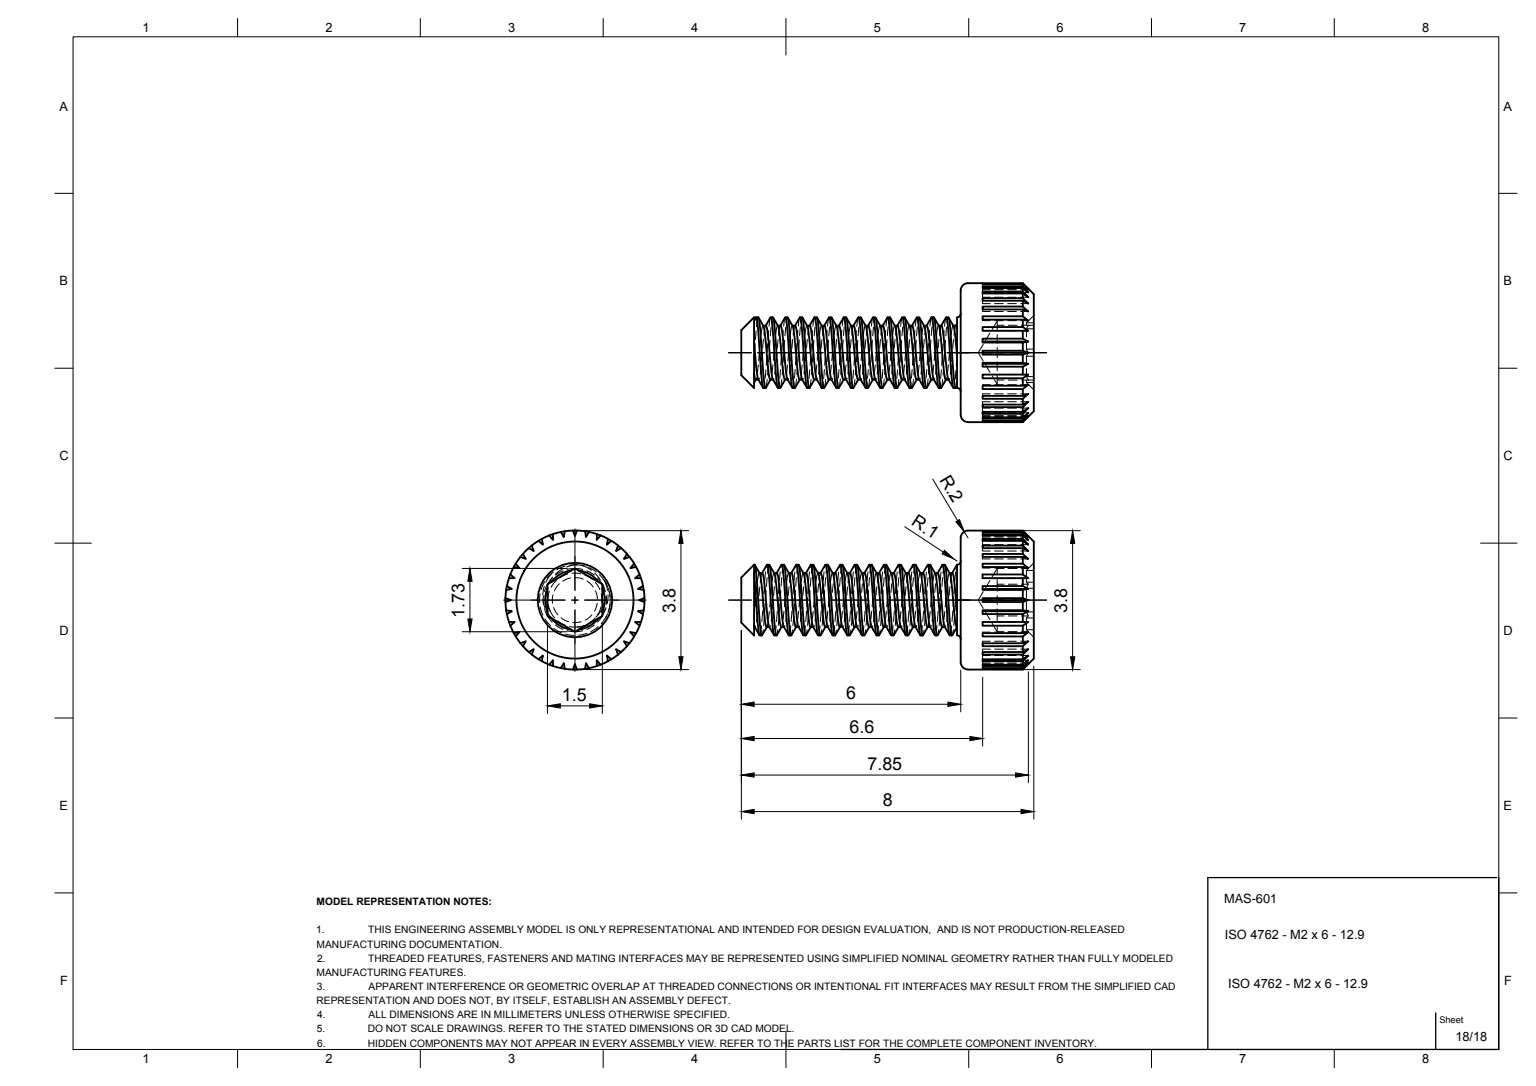
ISO-10303-21;
HEADER;
FILE_DESCRIPTION((''),'2;1');
FILE_NAME('ISO 4762 - M2 x 6 - 12.9.step','2026-10-06T07:37:42+05:00',(''),(''),'','','');
FILE_SCHEMA (('AUTOMOTIVE_DESIGN { 1 0 10303 214 3 1 1 }'));
ENDSEC;
DATA;
#10=MECHANICAL_DESIGN_GEOMETRIC_PRESENTATION_REPRESENTATION('',(#386),#18757);
#243=B_SPLINE_SURFACE_WITH_KNOTS('',3,3,((#16462,#16463,#16464,#16465,#16466,
#16467,#16468,#16469,#16470,#16471,#16472,#16473,#16474,#16475,#16476,#16477,
#16478,#16479,#16480,#16481,#16482,#16483,#16484,#16485,#16486,#16487,#16488,
#16489,#16490,#16491,#16492,#16493,#16494,#16495,#16496,#16497,#16498,#16499,
#16500,#16501,#16502,#16503,#16504,#16505,#16506,#16507,#16508,#16509,#16510,
#16511,#16512,#16513,#16514,#16515,#16516,#16517,#16518,#16519,#16520,#16521,
#16522,#16523,#16524,#16525,#16526,#16527,#16528,#16529,#16530,#16531,#16532,
#16533,#16534,#16535,#16536,#16537,#16538,#16539,#16540,#16541,#16542,#16543,
#16544,#16545,#16546,#16547,#16548,#16549,#16550,#16551,#16552,#16553,#16554),
(#16555,#16556,#16557,#16558,#16559,#16560,#16561,#16562,#16563,#16564,
#16565,#16566,#16567,#16568,#16569,#16570,#16571,#16572,#16573,#16574,#16575,
#16576,#16577,#16578,#16579,#16580,#16581,#16582,#16583,#16584,#16585,#16586,
#16587,#16588,#16589,#16590,#16591,#16592,#16593,#16594,#16595,#16596,#16597,
#16598,#16599,#16600,#16601,#16602,#16603,#16604,#16605,#16606,#16607,#16608,
#16609,#16610,#16611,#16612,#16613,#16614,#16615,#16616,#16617,#16618,#16619,
#16620,#16621,#16622,#16623,#16624,#16625,#16626,#16627,#16628,#16629,#16630,
#16631,#16632,#16633,#16634,#16635,#16636,#16637,#16638,#16639,#16640,#16641,
#16642,#16643,#16644,#16645,#16646,#16647),(#16648,#16649,#16650,#16651,
#16652,#16653,#16654,#16655,#16656,#16657,#16658,#16659,#16660,#16661,#16662,
#16663,#16664,#16665,#16666,#16667,#16668,#16669,#16670,#16671,#16672,#16673,
#16674,#16675,#16676,#16677,#16678,#16679,#16680,#16681,#16682,#16683,#16684,
#16685,#16686,#16687,#16688,#16689,#16690,#16691,#16692,#16693,#16694,#16695,
#16696,#16697,#16698,#16699,#16700,#16701,#16702,#16703,#16704,#16705,#16706,
#16707,#16708,#16709,#16710,#16711,#16712,#16713,#16714,#16715,#16716,#16717,
#16718,#16719,#16720,#16721,#16722,#16723,#16724,#16725,#16726,#16727,#16728,
#16729,#16730,#16731,#16732,#16733,#16734,#16735,#16736,#16737,#16738,#16739,
#16740),(#16741,#16742,#16743,#16744,#16745,#16746,#16747,#16748,#16749,
#16750,#16751,#16752,#16753,#16754,#16755,#16756,#16757,#16758,#16759,#16760,
#16761,#16762,#16763,#16764,#16765,#16766,#16767,#16768,#16769,#16770,#16771,
#16772,#16773,#16774,#16775,#16776,#16777,#16778,#16779,#16780,#16781,#16782,
#16783,#16784,#16785,#16786,#16787,#16788,#16789,#16790,#16791,#16792,#16793,
#16794,#16795,#16796,#16797,#16798,#16799,#16800,#16801,#16802,#16803,#16804,
#16805,#16806,#16807,#16808,#16809,#16810,#16811,#16812,#16813,#16814,#16815,
#16816,#16817,#16818,#16819,#16820,#16821,#16822,#16823,#16824,#16825,#16826,
#16827,#16828,#16829,#16830,#16831,#16832,#16833)),.UNSPECIFIED.,.F.,.F.,
 .F.,(4,4),(4,1,1,1,1,1,1,1,1,1,1,1,1,1,1,1,1,1,1,1,1,1,1,1,1,1,1,1,1,1,
1,1,1,1,1,1,1,1,1,1,1,1,1,1,1,1,1,1,1,1,1,1,1,1,1,1,1,1,1,1,1,1,1,1,1,1,
1,1,1,1,1,1,1,1,1,1,1,1,1,1,1,1,1,1,1,1,1,1,1,1,4),(0.,0.026298304761587),
(8.30929135176524,9.30089868691122,10.2925060220572,11.2841133572032,12.2757206923492,
13.2673280274952,14.2589353626411,15.2505426977871,16.2421500329331,17.2337573680791,
18.2253647032251,19.2169720383711,20.2085793735171,21.200186708663,22.191794043809,
23.183401378955,24.175008714101,25.166616049247,26.158223384393,27.149830719539,
28.1414380546849,29.1330453898309,30.1246527249769,31.1162600601229,32.1078673952689,
33.0994747304149,34.0910820655609,35.0826894007068,36.0742967358528,37.0659040709988,
38.0575114061448,39.0491187412908,40.0407260764368,41.0323334115828,42.0239407467287,
43.0155480818747,44.0071554170207,44.9987627521667,45.9903700873127,46.9819774224587,
47.9735847576047,48.9651920927506,49.9567994278966,50.9484067630426,51.9400140981886,
52.9316214333346,53.9232287684806,54.9148361036265,55.9064434387725,56.8980507739185,
57.8896581090645,58.8812654442105,59.8728727793565,60.8644801145025,61.8560874496484,
62.8476947847944,63.8393021199404,64.8309094550864,65.8225167902324,66.8141241253784,
67.8057314605244,68.7973387956703,69.7889461308163,70.7805534659623,71.7721608011083,
72.7637681362543,73.7553754714003,74.7469828065463,75.7385901416922,76.7301974768382,
77.7218048119842,78.7134121471302,79.7050194822762,80.6966268174222,81.6882341525682,
82.6798414877141,83.6714488228601,84.6630561580061,85.6546634931521,86.6462708282981,
87.6378781634441,88.62948549859,89.621092833736,90.612700168882,91.604307504028,
92.595914839174,93.58752217432,94.579129509466,95.5707368446119,96.5623441797579,
97.5539515149039),.UNSPECIFIED.) ;
#244=B_SPLINE_SURFACE_WITH_KNOTS('',3,3,((#17024,#17025,#17026,#17027,#17028,
#17029,#17030,#17031,#17032,#17033,#17034,#17035,#17036,#17037,#17038,#17039,
#17040,#17041,#17042,#17043,#17044,#17045,#17046,#17047,#17048,#17049,#17050,
#17051,#17052,#17053,#17054,#17055,#17056,#17057,#17058,#17059,#17060,#17061,
#17062,#17063,#17064,#17065,#17066,#17067,#17068,#17069,#17070,#17071,#17072,
#17073,#17074,#17075,#17076,#17077,#17078,#17079,#17080,#17081,#17082,#17083,
#17084,#17085,#17086,#17087,#17088,#17089,#17090,#17091,#17092,#17093,#17094,
#17095,#17096,#17097,#17098,#17099,#17100,#17101,#17102,#17103,#17104,#17105,
#17106,#17107,#17108,#17109,#17110,#17111,#17112,#17113,#17114,#17115,#17116),
(#17117,#17118,#17119,#17120,#17121,#17122,#17123,#17124,#17125,#17126,
#17127,#17128,#17129,#17130,#17131,#17132,#17133,#17134,#17135,#17136,#17137,
#17138,#17139,#17140,#17141,#17142,#17143,#17144,#17145,#17146,#17147,#17148,
#17149,#17150,#17151,#17152,#17153,#17154,#17155,#17156,#17157,#17158,#17159,
#17160,#17161,#17162,#17163,#17164,#17165,#17166,#17167,#17168,#17169,#17170,
#17171,#17172,#17173,#17174,#17175,#17176,#17177,#17178,#17179,#17180,#17181,
#17182,#17183,#17184,#17185,#17186,#17187,#17188,#17189,#17190,#17191,#17192,
#17193,#17194,#17195,#17196,#17197,#17198,#17199,#17200,#17201,#17202,#17203,
#17204,#17205,#17206,#17207,#17208,#17209),(#17210,#17211,#17212,#17213,
#17214,#17215,#17216,#17217,#17218,#17219,#17220,#17221,#17222,#17223,#17224,
#17225,#17226,#17227,#17228,#17229,#17230,#17231,#17232,#17233,#17234,#17235,
#17236,#17237,#17238,#17239,#17240,#17241,#17242,#17243,#17244,#17245,#17246,
#17247,#17248,#17249,#17250,#17251,#17252,#17253,#17254,#17255,#17256,#17257,
#17258,#17259,#17260,#17261,#17262,#17263,#17264,#17265,#17266,#17267,#17268,
#17269,#17270,#17271,#17272,#17273,#17274,#17275,#17276,#17277,#17278,#17279,
#17280,#17281,#17282,#17283,#17284,#17285,#17286,#17287,#17288,#17289,#17290,
#17291,#17292,#17293,#17294,#17295,#17296,#17297,#17298,#17299,#17300,#17301,
#17302),(#17303,#17304,#17305,#17306,#17307,#17308,#17309,#17310,#17311,
#17312,#17313,#17314,#17315,#17316,#17317,#17318,#17319,#17320,#17321,#17322,
#17323,#17324,#17325,#17326,#17327,#17328,#17329,#17330,#17331,#17332,#17333,
#17334,#17335,#17336,#17337,#17338,#17339,#17340,#17341,#17342,#17343,#17344,
#17345,#17346,#17347,#17348,#17349,#17350,#17351,#17352,#17353,#17354,#17355,
#17356,#17357,#17358,#17359,#17360,#17361,#17362,#17363,#17364,#17365,#17366,
#17367,#17368,#17369,#17370,#17371,#17372,#17373,#17374,#17375,#17376,#17377,
#17378,#17379,#17380,#17381,#17382,#17383,#17384,#17385,#17386,#17387,#17388,
#17389,#17390,#17391,#17392,#17393,#17394,#17395)),.UNSPECIFIED.,.F.,.F.,
 .F.,(4,4),(4,1,1,1,1,1,1,1,1,1,1,1,1,1,1,1,1,1,1,1,1,1,1,1,1,1,1,1,1,1,
1,1,1,1,1,1,1,1,1,1,1,1,1,1,1,1,1,1,1,1,1,1,1,1,1,1,1,1,1,1,1,1,1,1,1,1,
1,1,1,1,1,1,1,1,1,1,1,1,1,1,1,1,1,1,1,1,1,1,1,1,4),(0.,0.026298304761587),
(11.6163931973414,12.6080005324874,13.5996078676334,14.5912152027794,15.5828225379253,
16.5744298730713,17.5660372082173,18.5576445433633,19.5492518785093,20.5408592136553,
21.5324665488013,22.5240738839472,23.5156812190932,24.5072885542392,25.4988958893852,
26.4905032245312,27.4821105596772,28.4737178948232,29.4653252299691,30.4569325651151,
31.4485399002611,32.4401472354071,33.4317545705531,34.4233619056991,35.4149692408451,
36.406576575991,37.398183911137,38.389791246283,39.381398581429,40.373005916575,
41.364613251721,42.356220586867,43.3478279220129,44.3394352571589,45.3310425923049,
46.3226499274509,47.3142572625969,48.3058645977429,49.2974719328889,50.2890792680348,
51.2806866031808,52.2722939383268,53.2639012734728,54.2555086086188,55.2471159437648,
56.2387232789108,57.2303306140567,58.2219379492027,59.2135452843487,60.2051526194947,
61.1967599546407,62.1883672897867,63.1799746249327,64.1715819600786,65.1631892952246,
66.1547966303706,67.1464039655166,68.1380113006626,69.1296186358086,70.1212259709546,
71.1128333061005,72.1044406412465,73.0960479763925,74.0876553115385,75.0792626466845,
76.0708699818305,77.0624773169765,78.0540846521224,79.0456919872684,80.0372993224144,
81.0289066575604,82.0205139927064,83.0121213278524,84.0037286629984,84.9953359981443,
85.9869433332903,86.9785506684363,87.9701580035823,88.9617653387283,89.9533726738743,
90.9449800090203,91.9365873441662,92.9281946793122,93.9198020144582,94.9114093496042,
95.9030166847502,96.8946240198962,97.8862313550422,98.8778386901881,99.8694460253341,
100.86105336048),.UNSPECIFIED.) ;
#247=(
BOUNDED_CURVE()
B_SPLINE_CURVE(2,(#17435,#17436,#17437),.UNSPECIFIED.,.F.,.F.)
B_SPLINE_CURVE_WITH_KNOTS((3,3),(0.,0.0208203041101871),.UNSPECIFIED.)
CURVE()
GEOMETRIC_REPRESENTATION_ITEM()
RATIONAL_B_SPLINE_CURVE((1.,1.00198318129131,1.00207919474364))
REPRESENTATION_ITEM('')
) ;
#248=(
BOUNDED_CURVE()
B_SPLINE_CURVE(2,(#17441,#17442,#17443),.UNSPECIFIED.,.F.,.F.)
B_SPLINE_CURVE_WITH_KNOTS((3,3),(0.0229388536475348,0.0437591577578469),
 .UNSPECIFIED.)
CURVE()
GEOMETRIC_REPRESENTATION_ITEM()
RATIONAL_B_SPLINE_CURVE((1.00207919472777,1.00198318127619,1.))
REPRESENTATION_ITEM('')
) ;
#249=(
BOUNDED_CURVE()
B_SPLINE_CURVE(2,(#17736,#17737,#17738),.UNSPECIFIED.,.F.,.F.)
B_SPLINE_CURVE_WITH_KNOTS((3,3),(0.,0.020820304110201),.UNSPECIFIED.)
CURVE()
GEOMETRIC_REPRESENTATION_ITEM()
RATIONAL_B_SPLINE_CURVE((1.,1.00198318127951,1.00207919473126))
REPRESENTATION_ITEM('')
) ;
#250=(
BOUNDED_CURVE()
B_SPLINE_CURVE(2,(#17740,#17741,#17742),.UNSPECIFIED.,.F.,.F.)
B_SPLINE_CURVE_WITH_KNOTS((3,3),(0.0229388536477412,0.043759157757845),
 .UNSPECIFIED.)
CURVE()
GEOMETRIC_REPRESENTATION_ITEM()
RATIONAL_B_SPLINE_CURVE((1.00207919475953,1.00198318130646,1.))
REPRESENTATION_ITEM('')
) ;
#251=(
BOUNDED_CURVE()
B_SPLINE_CURVE(2,(#17750,#17751,#17752),.UNSPECIFIED.,.F.,.F.)
B_SPLINE_CURVE_WITH_KNOTS((3,3),(0.0229388536475751,0.0437591577578467),
 .UNSPECIFIED.)
CURVE()
GEOMETRIC_REPRESENTATION_ITEM()
RATIONAL_B_SPLINE_CURVE((1.00207919474459,1.00198318129223,1.))
REPRESENTATION_ITEM('')
) ;
#252=(
BOUNDED_CURVE()
B_SPLINE_CURVE(2,(#17754,#17755,#17756),.UNSPECIFIED.,.F.,.F.)
B_SPLINE_CURVE_WITH_KNOTS((3,3),(0.,0.0208203041102522),.UNSPECIFIED.)
CURVE()
GEOMETRIC_REPRESENTATION_ITEM()
RATIONAL_B_SPLINE_CURVE((1.,1.00198318129313,1.00207919474555))
REPRESENTATION_ITEM('')
) ;
#253=(
BOUNDED_CURVE()
B_SPLINE_CURVE(2,(#17757,#17758,#17759),.UNSPECIFIED.,.F.,.F.)
B_SPLINE_CURVE_WITH_KNOTS((3,3),(0.0229388536477059,0.0437591577578443),
 .UNSPECIFIED.)
CURVE()
GEOMETRIC_REPRESENTATION_ITEM()
RATIONAL_B_SPLINE_CURVE((1.00207919475079,1.00198318129812,1.))
REPRESENTATION_ITEM('')
) ;
#254=(
BOUNDED_CURVE()
B_SPLINE_CURVE(2,(#17761,#17762,#17763),.UNSPECIFIED.,.F.,.F.)
B_SPLINE_CURVE_WITH_KNOTS((3,3),(0.,0.0208203041101399),.UNSPECIFIED.)
CURVE()
GEOMETRIC_REPRESENTATION_ITEM()
RATIONAL_B_SPLINE_CURVE((1.,1.00198318129313,1.00207919474555))
REPRESENTATION_ITEM('')
) ;
#255=(
BOUNDED_CURVE()
B_SPLINE_CURVE(2,(#17764,#17765,#17766),.UNSPECIFIED.,.F.,.F.)
B_SPLINE_CURVE_WITH_KNOTS((3,3),(0.022938853647565,0.0437591577578454),
 .UNSPECIFIED.)
CURVE()
GEOMETRIC_REPRESENTATION_ITEM()
RATIONAL_B_SPLINE_CURVE((1.00207919472218,1.00198318127084,1.))
REPRESENTATION_ITEM('')
) ;
#256=(
BOUNDED_CURVE()
B_SPLINE_CURVE(2,(#17768,#17769,#17770),.UNSPECIFIED.,.F.,.F.)
B_SPLINE_CURVE_WITH_KNOTS((3,3),(0.,0.0208203041101981),.UNSPECIFIED.)
CURVE()
GEOMETRIC_REPRESENTATION_ITEM()
RATIONAL_B_SPLINE_CURVE((1.,1.00198318127317,1.00207919472462))
REPRESENTATION_ITEM('')
) ;
#257=(
BOUNDED_CURVE()
B_SPLINE_CURVE(2,(#17771,#17772,#17773),.UNSPECIFIED.,.F.,.F.)
B_SPLINE_CURVE_WITH_KNOTS((3,3),(0.0229388536476133,0.0437591577578448),
 .UNSPECIFIED.)
CURVE()
GEOMETRIC_REPRESENTATION_ITEM()
RATIONAL_B_SPLINE_CURVE((1.00207919472699,1.00198318127544,1.))
REPRESENTATION_ITEM('')
) ;
#258=(
BOUNDED_CURVE()
B_SPLINE_CURVE(2,(#17775,#17776,#17777),.UNSPECIFIED.,.F.,.F.)
B_SPLINE_CURVE_WITH_KNOTS((3,3),(0.,0.0208203041102164),.UNSPECIFIED.)
CURVE()
GEOMETRIC_REPRESENTATION_ITEM()
RATIONAL_B_SPLINE_CURVE((1.,1.00198318130011,1.00207919475286))
REPRESENTATION_ITEM('')
) ;
#259=(
BOUNDED_CURVE()
B_SPLINE_CURVE(2,(#17778,#17779,#17780),.UNSPECIFIED.,.F.,.F.)
B_SPLINE_CURVE_WITH_KNOTS((3,3),(0.022938853647606,0.0437591577578459),
 .UNSPECIFIED.)
CURVE()
GEOMETRIC_REPRESENTATION_ITEM()
RATIONAL_B_SPLINE_CURVE((1.00207919473573,1.00198318128377,1.))
REPRESENTATION_ITEM('')
) ;
#260=(
BOUNDED_CURVE()
B_SPLINE_CURVE(2,(#17782,#17783,#17784),.UNSPECIFIED.,.F.,.F.)
B_SPLINE_CURVE_WITH_KNOTS((3,3),(0.,0.0208203041102311),.UNSPECIFIED.)
CURVE()
GEOMETRIC_REPRESENTATION_ITEM()
RATIONAL_B_SPLINE_CURVE((1.,1.00198318129299,1.0020791947454))
REPRESENTATION_ITEM('')
) ;
#261=(
BOUNDED_CURVE()
B_SPLINE_CURVE(2,(#17785,#17786,#17787),.UNSPECIFIED.,.F.,.F.)
B_SPLINE_CURVE_WITH_KNOTS((3,3),(0.0229388536476449,0.0437591577578444),
 .UNSPECIFIED.)
CURVE()
GEOMETRIC_REPRESENTATION_ITEM()
RATIONAL_B_SPLINE_CURVE((1.0020791947485,1.00198318129594,1.))
REPRESENTATION_ITEM('')
) ;
#262=(
BOUNDED_CURVE()
B_SPLINE_CURVE(2,(#17789,#17790,#17791),.UNSPECIFIED.,.F.,.F.)
B_SPLINE_CURVE_WITH_KNOTS((3,3),(0.,0.0208203041101845),.UNSPECIFIED.)
CURVE()
GEOMETRIC_REPRESENTATION_ITEM()
RATIONAL_B_SPLINE_CURVE((1.,1.00198318129298,1.00207919474539))
REPRESENTATION_ITEM('')
) ;
#263=(
BOUNDED_CURVE()
B_SPLINE_CURVE(2,(#17792,#17793,#17794),.UNSPECIFIED.,.F.,.F.)
B_SPLINE_CURVE_WITH_KNOTS((3,3),(0.0229388536476154,0.0437591577578439),
 .UNSPECIFIED.)
CURVE()
GEOMETRIC_REPRESENTATION_ITEM()
RATIONAL_B_SPLINE_CURVE((1.00207919473424,1.00198318128235,1.))
REPRESENTATION_ITEM('')
) ;
#264=(
BOUNDED_CURVE()
B_SPLINE_CURVE(2,(#17796,#17797,#17798),.UNSPECIFIED.,.F.,.F.)
B_SPLINE_CURVE_WITH_KNOTS((3,3),(0.,0.0208203041102815),.UNSPECIFIED.)
CURVE()
GEOMETRIC_REPRESENTATION_ITEM()
RATIONAL_B_SPLINE_CURVE((1.,1.00198318127347,1.00207919472493))
REPRESENTATION_ITEM('')
) ;
#265=(
BOUNDED_CURVE()
B_SPLINE_CURVE(2,(#17799,#17800,#17801),.UNSPECIFIED.,.F.,.F.)
B_SPLINE_CURVE_WITH_KNOTS((3,3),(0.0229388536476481,0.0437591577578452),
 .UNSPECIFIED.)
CURVE()
GEOMETRIC_REPRESENTATION_ITEM()
RATIONAL_B_SPLINE_CURVE((1.00207919474569,1.00198318129326,1.))
REPRESENTATION_ITEM('')
) ;
#266=(
BOUNDED_CURVE()
B_SPLINE_CURVE(2,(#17803,#17804,#17805),.UNSPECIFIED.,.F.,.F.)
B_SPLINE_CURVE_WITH_KNOTS((3,3),(0.,0.0208203041101622),.UNSPECIFIED.)
CURVE()
GEOMETRIC_REPRESENTATION_ITEM()
RATIONAL_B_SPLINE_CURVE((1.,1.00198318130135,1.00207919475417))
REPRESENTATION_ITEM('')
) ;
#267=(
BOUNDED_CURVE()
B_SPLINE_CURVE(2,(#17806,#17807,#17808),.UNSPECIFIED.,.F.,.F.)
B_SPLINE_CURVE_WITH_KNOTS((3,3),(0.0229388536475943,0.0437591577578443),
 .UNSPECIFIED.)
CURVE()
GEOMETRIC_REPRESENTATION_ITEM()
RATIONAL_B_SPLINE_CURVE((1.00207919473131,1.00198318127955,1.))
REPRESENTATION_ITEM('')
) ;
#268=(
BOUNDED_CURVE()
B_SPLINE_CURVE(2,(#17810,#17811,#17812),.UNSPECIFIED.,.F.,.F.)
B_SPLINE_CURVE_WITH_KNOTS((3,3),(0.,0.0208203041102868),.UNSPECIFIED.)
CURVE()
GEOMETRIC_REPRESENTATION_ITEM()
RATIONAL_B_SPLINE_CURVE((1.,1.00198318127515,1.00207919472669))
REPRESENTATION_ITEM('')
) ;
#269=(
BOUNDED_CURVE()
B_SPLINE_CURVE(2,(#17813,#17814,#17815),.UNSPECIFIED.,.F.,.F.)
B_SPLINE_CURVE_WITH_KNOTS((3,3),(0.0229388536476239,0.0437591577578459),
 .UNSPECIFIED.)
CURVE()
GEOMETRIC_REPRESENTATION_ITEM()
RATIONAL_B_SPLINE_CURVE((1.00207919474537,1.00198318129297,1.))
REPRESENTATION_ITEM('')
) ;
#270=(
BOUNDED_CURVE()
B_SPLINE_CURVE(2,(#17817,#17818,#17819),.UNSPECIFIED.,.F.,.F.)
B_SPLINE_CURVE_WITH_KNOTS((3,3),(0.,0.0208203041102119),.UNSPECIFIED.)
CURVE()
GEOMETRIC_REPRESENTATION_ITEM()
RATIONAL_B_SPLINE_CURVE((1.,1.00198318128545,1.00207919473749))
REPRESENTATION_ITEM('')
) ;
#271=(
BOUNDED_CURVE()
B_SPLINE_CURVE(2,(#17820,#17821,#17822),.UNSPECIFIED.,.F.,.F.)
B_SPLINE_CURVE_WITH_KNOTS((3,3),(0.022938853647645,0.0437591577578424),
 .UNSPECIFIED.)
CURVE()
GEOMETRIC_REPRESENTATION_ITEM()
RATIONAL_B_SPLINE_CURVE((1.00207919473173,1.00198318127995,1.))
REPRESENTATION_ITEM('')
) ;
#272=(
BOUNDED_CURVE()
B_SPLINE_CURVE(2,(#17824,#17825,#17826),.UNSPECIFIED.,.F.,.F.)
B_SPLINE_CURVE_WITH_KNOTS((3,3),(0.,0.0208203041101933),.UNSPECIFIED.)
CURVE()
GEOMETRIC_REPRESENTATION_ITEM()
RATIONAL_B_SPLINE_CURVE((1.,1.00198318129507,1.00207919474759))
REPRESENTATION_ITEM('')
) ;
#273=(
BOUNDED_CURVE()
B_SPLINE_CURVE(2,(#17827,#17828,#17829),.UNSPECIFIED.,.F.,.F.)
B_SPLINE_CURVE_WITH_KNOTS((3,3),(0.0229388536476438,0.0437591577578434),
 .UNSPECIFIED.)
CURVE()
GEOMETRIC_REPRESENTATION_ITEM()
RATIONAL_B_SPLINE_CURVE((1.00207919475882,1.00198318130579,1.))
REPRESENTATION_ITEM('')
) ;
#274=(
BOUNDED_CURVE()
B_SPLINE_CURVE(2,(#17831,#17832,#17833),.UNSPECIFIED.,.F.,.F.)
B_SPLINE_CURVE_WITH_KNOTS((3,3),(0.,0.020820304110188),.UNSPECIFIED.)
CURVE()
GEOMETRIC_REPRESENTATION_ITEM()
RATIONAL_B_SPLINE_CURVE((1.,1.0019831812866,1.0020791947387))
REPRESENTATION_ITEM('')
) ;
#275=(
BOUNDED_CURVE()
B_SPLINE_CURVE(2,(#17834,#17835,#17836),.UNSPECIFIED.,.F.,.F.)
B_SPLINE_CURVE_WITH_KNOTS((3,3),(0.0229388536475715,0.0437591577578452),
 .UNSPECIFIED.)
CURVE()
GEOMETRIC_REPRESENTATION_ITEM()
RATIONAL_B_SPLINE_CURVE((1.00207919474451,1.00198318129215,1.))
REPRESENTATION_ITEM('')
) ;
#276=(
BOUNDED_CURVE()
B_SPLINE_CURVE(2,(#17838,#17839,#17840),.UNSPECIFIED.,.F.,.F.)
B_SPLINE_CURVE_WITH_KNOTS((3,3),(0.,0.0208203041102257),.UNSPECIFIED.)
CURVE()
GEOMETRIC_REPRESENTATION_ITEM()
RATIONAL_B_SPLINE_CURVE((1.,1.00198318129643,1.00207919474901))
REPRESENTATION_ITEM('')
) ;
#277=(
BOUNDED_CURVE()
B_SPLINE_CURVE(2,(#17841,#17842,#17843),.UNSPECIFIED.,.F.,.F.)
B_SPLINE_CURVE_WITH_KNOTS((3,3),(0.0229388536476128,0.0437591577578448),
 .UNSPECIFIED.)
CURVE()
GEOMETRIC_REPRESENTATION_ITEM()
RATIONAL_B_SPLINE_CURVE((1.00207919474488,1.0019831812925,1.))
REPRESENTATION_ITEM('')
) ;
#278=(
BOUNDED_CURVE()
B_SPLINE_CURVE(2,(#17845,#17846,#17847),.UNSPECIFIED.,.F.,.F.)
B_SPLINE_CURVE_WITH_KNOTS((3,3),(0.,0.0208203041102548),.UNSPECIFIED.)
CURVE()
GEOMETRIC_REPRESENTATION_ITEM()
RATIONAL_B_SPLINE_CURVE((1.,1.00198318128365,1.0020791947356))
REPRESENTATION_ITEM('')
) ;
#279=(
BOUNDED_CURVE()
B_SPLINE_CURVE(2,(#17848,#17849,#17850),.UNSPECIFIED.,.F.,.F.)
B_SPLINE_CURVE_WITH_KNOTS((3,3),(0.0229388536476842,0.0437591577578424),
 .UNSPECIFIED.)
CURVE()
GEOMETRIC_REPRESENTATION_ITEM()
RATIONAL_B_SPLINE_CURVE((1.00207919473831,1.00198318128623,1.))
REPRESENTATION_ITEM('')
) ;
#280=(
BOUNDED_CURVE()
B_SPLINE_CURVE(2,(#17852,#17853,#17854),.UNSPECIFIED.,.F.,.F.)
B_SPLINE_CURVE_WITH_KNOTS((3,3),(0.,0.0208203041101929),.UNSPECIFIED.)
CURVE()
GEOMETRIC_REPRESENTATION_ITEM()
RATIONAL_B_SPLINE_CURVE((1.,1.00198318129994,1.00207919475269))
REPRESENTATION_ITEM('')
) ;
#281=(
BOUNDED_CURVE()
B_SPLINE_CURVE(2,(#17855,#17856,#17857),.UNSPECIFIED.,.F.,.F.)
B_SPLINE_CURVE_WITH_KNOTS((3,3),(0.0229388536476416,0.0437591577578453),
 .UNSPECIFIED.)
CURVE()
GEOMETRIC_REPRESENTATION_ITEM()
RATIONAL_B_SPLINE_CURVE((1.0020791947507,1.00198318129804,1.))
REPRESENTATION_ITEM('')
) ;
#282=(
BOUNDED_CURVE()
B_SPLINE_CURVE(2,(#17859,#17860,#17861),.UNSPECIFIED.,.F.,.F.)
B_SPLINE_CURVE_WITH_KNOTS((3,3),(0.,0.0208203041102008),.UNSPECIFIED.)
CURVE()
GEOMETRIC_REPRESENTATION_ITEM()
RATIONAL_B_SPLINE_CURVE((1.,1.00198318128547,1.00207919473751))
REPRESENTATION_ITEM('')
) ;
#283=(
BOUNDED_CURVE()
B_SPLINE_CURVE(2,(#17862,#17863,#17864),.UNSPECIFIED.,.F.,.F.)
B_SPLINE_CURVE_WITH_KNOTS((3,3),(0.0229388536475931,0.0437591577578445),
 .UNSPECIFIED.)
CURVE()
GEOMETRIC_REPRESENTATION_ITEM()
RATIONAL_B_SPLINE_CURVE((1.00207919474108,1.00198318128887,1.))
REPRESENTATION_ITEM('')
) ;
#284=(
BOUNDED_CURVE()
B_SPLINE_CURVE(2,(#17866,#17867,#17868),.UNSPECIFIED.,.F.,.F.)
B_SPLINE_CURVE_WITH_KNOTS((3,3),(0.,0.0208203041102136),.UNSPECIFIED.)
CURVE()
GEOMETRIC_REPRESENTATION_ITEM()
RATIONAL_B_SPLINE_CURVE((1.,1.00198318127179,1.00207919472318))
REPRESENTATION_ITEM('')
) ;
#285=(
BOUNDED_CURVE()
B_SPLINE_CURVE(2,(#17869,#17870,#17871),.UNSPECIFIED.,.F.,.F.)
B_SPLINE_CURVE_WITH_KNOTS((3,3),(0.0229388536475417,0.0437591577578453),
 .UNSPECIFIED.)
CURVE()
GEOMETRIC_REPRESENTATION_ITEM()
RATIONAL_B_SPLINE_CURVE((1.00207919475326,1.0019831813005,1.))
REPRESENTATION_ITEM('')
) ;
#286=(
BOUNDED_CURVE()
B_SPLINE_CURVE(2,(#17873,#17874,#17875),.UNSPECIFIED.,.F.,.F.)
B_SPLINE_CURVE_WITH_KNOTS((3,3),(0.,0.0208203041102395),.UNSPECIFIED.)
CURVE()
GEOMETRIC_REPRESENTATION_ITEM()
RATIONAL_B_SPLINE_CURVE((1.,1.00198318130368,1.0020791947566))
REPRESENTATION_ITEM('')
) ;
#287=(
BOUNDED_CURVE()
B_SPLINE_CURVE(2,(#17876,#17877,#17878),.UNSPECIFIED.,.F.,.F.)
B_SPLINE_CURVE_WITH_KNOTS((3,3),(0.0229388536476164,0.0437591577578449),
 .UNSPECIFIED.)
CURVE()
GEOMETRIC_REPRESENTATION_ITEM()
RATIONAL_B_SPLINE_CURVE((1.00207919474665,1.00198318129418,1.))
REPRESENTATION_ITEM('')
) ;
#288=(
BOUNDED_CURVE()
B_SPLINE_CURVE(2,(#17880,#17881,#17882),.UNSPECIFIED.,.F.,.F.)
B_SPLINE_CURVE_WITH_KNOTS((3,3),(0.,0.0208203041102497),.UNSPECIFIED.)
CURVE()
GEOMETRIC_REPRESENTATION_ITEM()
RATIONAL_B_SPLINE_CURVE((1.,1.00198318126206,1.00207919471297))
REPRESENTATION_ITEM('')
) ;
#289=(
BOUNDED_CURVE()
B_SPLINE_CURVE(2,(#17883,#17884,#17885),.UNSPECIFIED.,.F.,.F.)
B_SPLINE_CURVE_WITH_KNOTS((3,3),(0.0229388536475813,0.0437591577578465),
 .UNSPECIFIED.)
CURVE()
GEOMETRIC_REPRESENTATION_ITEM()
RATIONAL_B_SPLINE_CURVE((1.00207919474568,1.00198318129326,1.))
REPRESENTATION_ITEM('')
) ;
#290=(
BOUNDED_CURVE()
B_SPLINE_CURVE(2,(#17887,#17888,#17889),.UNSPECIFIED.,.F.,.F.)
B_SPLINE_CURVE_WITH_KNOTS((3,3),(0.,0.0208203041102125),.UNSPECIFIED.)
CURVE()
GEOMETRIC_REPRESENTATION_ITEM()
RATIONAL_B_SPLINE_CURVE((1.,1.00198318129832,1.00207919475098))
REPRESENTATION_ITEM('')
) ;
#291=(
BOUNDED_CURVE()
B_SPLINE_CURVE(2,(#17890,#17891,#17892),.UNSPECIFIED.,.F.,.F.)
B_SPLINE_CURVE_WITH_KNOTS((3,3),(0.0229388536475884,0.043759157757846),
 .UNSPECIFIED.)
CURVE()
GEOMETRIC_REPRESENTATION_ITEM()
RATIONAL_B_SPLINE_CURVE((1.00207919473695,1.00198318128494,1.))
REPRESENTATION_ITEM('')
) ;
#292=(
BOUNDED_CURVE()
B_SPLINE_CURVE(2,(#17894,#17895,#17896),.UNSPECIFIED.,.F.,.F.)
B_SPLINE_CURVE_WITH_KNOTS((3,3),(0.,0.0208203041102161),.UNSPECIFIED.)
CURVE()
GEOMETRIC_REPRESENTATION_ITEM()
RATIONAL_B_SPLINE_CURVE((1.,1.00198318130551,1.00207919475853))
REPRESENTATION_ITEM('')
) ;
#293=(
BOUNDED_CURVE()
B_SPLINE_CURVE(2,(#17897,#17898,#17899),.UNSPECIFIED.,.F.,.F.)
B_SPLINE_CURVE_WITH_KNOTS((3,3),(0.0229388536476204,0.0437591577578463),
 .UNSPECIFIED.)
CURVE()
GEOMETRIC_REPRESENTATION_ITEM()
RATIONAL_B_SPLINE_CURVE((1.00207919473782,1.00198318128577,1.))
REPRESENTATION_ITEM('')
) ;
#294=(
BOUNDED_CURVE()
B_SPLINE_CURVE(2,(#17901,#17902,#17903),.UNSPECIFIED.,.F.,.F.)
B_SPLINE_CURVE_WITH_KNOTS((3,3),(0.,0.0208203041102228),.UNSPECIFIED.)
CURVE()
GEOMETRIC_REPRESENTATION_ITEM()
RATIONAL_B_SPLINE_CURVE((1.,1.00198318128961,1.00207919474186))
REPRESENTATION_ITEM('')
) ;
#295=(
BOUNDED_CURVE()
B_SPLINE_CURVE(2,(#17904,#17905,#17906),.UNSPECIFIED.,.F.,.F.)
B_SPLINE_CURVE_WITH_KNOTS((3,3),(0.0229388536476005,0.0437591577578455),
 .UNSPECIFIED.)
CURVE()
GEOMETRIC_REPRESENTATION_ITEM()
RATIONAL_B_SPLINE_CURVE((1.00207919472128,1.00198318126998,1.))
REPRESENTATION_ITEM('')
) ;
#296=(
BOUNDED_CURVE()
B_SPLINE_CURVE(2,(#17908,#17909,#17910),.UNSPECIFIED.,.F.,.F.)
B_SPLINE_CURVE_WITH_KNOTS((3,3),(0.,0.0208203041102323),.UNSPECIFIED.)
CURVE()
GEOMETRIC_REPRESENTATION_ITEM()
RATIONAL_B_SPLINE_CURVE((1.,1.00198318129082,1.00207919474313))
REPRESENTATION_ITEM('')
) ;
#297=(
BOUNDED_CURVE()
B_SPLINE_CURVE(2,(#17911,#17912,#17913),.UNSPECIFIED.,.F.,.F.)
B_SPLINE_CURVE_WITH_KNOTS((3,3),(0.0229388536476069,0.0437591577578452),
 .UNSPECIFIED.)
CURVE()
GEOMETRIC_REPRESENTATION_ITEM()
RATIONAL_B_SPLINE_CURVE((1.00207919474246,1.00198318129019,1.))
REPRESENTATION_ITEM('')
) ;
#298=(
BOUNDED_CURVE()
B_SPLINE_CURVE(2,(#17915,#17916,#17917),.UNSPECIFIED.,.F.,.F.)
B_SPLINE_CURVE_WITH_KNOTS((3,3),(0.,0.0208203041102477),.UNSPECIFIED.)
CURVE()
GEOMETRIC_REPRESENTATION_ITEM()
RATIONAL_B_SPLINE_CURVE((1.,1.00198318127836,1.00207919473006))
REPRESENTATION_ITEM('')
) ;
#299=(
BOUNDED_CURVE()
B_SPLINE_CURVE(2,(#17918,#17919,#17920),.UNSPECIFIED.,.F.,.F.)
B_SPLINE_CURVE_WITH_KNOTS((3,3),(0.0229388536476238,0.0437591577578459),
 .UNSPECIFIED.)
CURVE()
GEOMETRIC_REPRESENTATION_ITEM()
RATIONAL_B_SPLINE_CURVE((1.0020791947311,1.00198318127935,1.))
REPRESENTATION_ITEM('')
) ;
#300=(
BOUNDED_CURVE()
B_SPLINE_CURVE(2,(#17922,#17923,#17924),.UNSPECIFIED.,.F.,.F.)
B_SPLINE_CURVE_WITH_KNOTS((3,3),(0.,0.0208203041102102),.UNSPECIFIED.)
CURVE()
GEOMETRIC_REPRESENTATION_ITEM()
RATIONAL_B_SPLINE_CURVE((1.,1.00198318128188,1.00207919473375))
REPRESENTATION_ITEM('')
) ;
#301=(
BOUNDED_CURVE()
B_SPLINE_CURVE(2,(#17925,#17926,#17927),.UNSPECIFIED.,.F.,.F.)
B_SPLINE_CURVE_WITH_KNOTS((3,3),(0.0229388536476158,0.0437591577578472),
 .UNSPECIFIED.)
CURVE()
GEOMETRIC_REPRESENTATION_ITEM()
RATIONAL_B_SPLINE_CURVE((1.00207919475336,1.00198318130059,1.))
REPRESENTATION_ITEM('')
) ;
#302=(
BOUNDED_CURVE()
B_SPLINE_CURVE(2,(#17929,#17930,#17931),.UNSPECIFIED.,.F.,.F.)
B_SPLINE_CURVE_WITH_KNOTS((3,3),(0.,0.0208203041102333),.UNSPECIFIED.)
CURVE()
GEOMETRIC_REPRESENTATION_ITEM()
RATIONAL_B_SPLINE_CURVE((1.,1.00198318128675,1.00207919473886))
REPRESENTATION_ITEM('')
) ;
#303=(
BOUNDED_CURVE()
B_SPLINE_CURVE(2,(#17932,#17933,#17934),.UNSPECIFIED.,.F.,.F.)
B_SPLINE_CURVE_WITH_KNOTS((3,3),(0.0229388536476674,0.0437591577578436),
 .UNSPECIFIED.)
CURVE()
GEOMETRIC_REPRESENTATION_ITEM()
RATIONAL_B_SPLINE_CURVE((1.00207919473716,1.00198318128513,1.))
REPRESENTATION_ITEM('')
) ;
#304=(
BOUNDED_CURVE()
B_SPLINE_CURVE(2,(#17936,#17937,#17938),.UNSPECIFIED.,.F.,.F.)
B_SPLINE_CURVE_WITH_KNOTS((3,3),(0.,0.0208203041101914),.UNSPECIFIED.)
CURVE()
GEOMETRIC_REPRESENTATION_ITEM()
RATIONAL_B_SPLINE_CURVE((1.,1.00198318129795,1.00207919475061))
REPRESENTATION_ITEM('')
) ;
#305=(
BOUNDED_CURVE()
B_SPLINE_CURVE(2,(#17939,#17940,#17941),.UNSPECIFIED.,.F.,.F.)
B_SPLINE_CURVE_WITH_KNOTS((3,3),(0.0229388536476256,0.0437591577578441),
 .UNSPECIFIED.)
CURVE()
GEOMETRIC_REPRESENTATION_ITEM()
RATIONAL_B_SPLINE_CURVE((1.00207919474269,1.00198318129041,1.))
REPRESENTATION_ITEM('')
) ;
#306=(
BOUNDED_CURVE()
B_SPLINE_CURVE(2,(#17943,#17944,#17945),.UNSPECIFIED.,.F.,.F.)
B_SPLINE_CURVE_WITH_KNOTS((3,3),(0.,0.0208203041102649),.UNSPECIFIED.)
CURVE()
GEOMETRIC_REPRESENTATION_ITEM()
RATIONAL_B_SPLINE_CURVE((1.,1.00198318128372,1.00207919473568))
REPRESENTATION_ITEM('')
) ;
#307=(
BOUNDED_CURVE()
B_SPLINE_CURVE(2,(#17946,#17947,#17948),.UNSPECIFIED.,.F.,.F.)
B_SPLINE_CURVE_WITH_KNOTS((3,3),(0.0229388536476116,0.0437591577578462),
 .UNSPECIFIED.)
CURVE()
GEOMETRIC_REPRESENTATION_ITEM()
RATIONAL_B_SPLINE_CURVE((1.00207919474123,1.00198318128901,1.))
REPRESENTATION_ITEM('')
) ;
#308=(
BOUNDED_CURVE()
B_SPLINE_CURVE(2,(#17950,#17951,#17952),.UNSPECIFIED.,.F.,.F.)
B_SPLINE_CURVE_WITH_KNOTS((3,3),(0.,0.0208203041102467),.UNSPECIFIED.)
CURVE()
GEOMETRIC_REPRESENTATION_ITEM()
RATIONAL_B_SPLINE_CURVE((1.,1.00198318128474,1.00207919473675))
REPRESENTATION_ITEM('')
) ;
#309=(
BOUNDED_CURVE()
B_SPLINE_CURVE(2,(#17953,#17954,#17955),.UNSPECIFIED.,.F.,.F.)
B_SPLINE_CURVE_WITH_KNOTS((3,3),(0.0229388536476399,0.0437591577578457),
 .UNSPECIFIED.)
CURVE()
GEOMETRIC_REPRESENTATION_ITEM()
RATIONAL_B_SPLINE_CURVE((1.00207919474381,1.00198318129148,1.))
REPRESENTATION_ITEM('')
) ;
#310=(
BOUNDED_CURVE()
B_SPLINE_CURVE(2,(#17957,#17958,#17959),.UNSPECIFIED.,.F.,.F.)
B_SPLINE_CURVE_WITH_KNOTS((3,3),(0.,0.0208203041102079),.UNSPECIFIED.)
CURVE()
GEOMETRIC_REPRESENTATION_ITEM()
RATIONAL_B_SPLINE_CURVE((1.,1.00198318129612,1.00207919474868))
REPRESENTATION_ITEM('')
) ;
#311=(
BOUNDED_CURVE()
B_SPLINE_CURVE(2,(#17960,#17961,#17962),.UNSPECIFIED.,.F.,.F.)
B_SPLINE_CURVE_WITH_KNOTS((3,3),(0.0229388536475489,0.043759157757846),
 .UNSPECIFIED.)
CURVE()
GEOMETRIC_REPRESENTATION_ITEM()
RATIONAL_B_SPLINE_CURVE((1.00207919471265,1.00198318126176,1.))
REPRESENTATION_ITEM('')
) ;
#312=(
BOUNDED_CURVE()
B_SPLINE_CURVE(2,(#17964,#17965,#17966),.UNSPECIFIED.,.F.,.F.)
B_SPLINE_CURVE_WITH_KNOTS((3,3),(0.,0.020820304110324),.UNSPECIFIED.)
CURVE()
GEOMETRIC_REPRESENTATION_ITEM()
RATIONAL_B_SPLINE_CURVE((1.,1.00198318127347,1.00207919472492))
REPRESENTATION_ITEM('')
) ;
#313=(
BOUNDED_CURVE()
B_SPLINE_CURVE(2,(#17967,#17968,#17969),.UNSPECIFIED.,.F.,.F.)
B_SPLINE_CURVE_WITH_KNOTS((3,3),(0.0229388536476511,0.0437591577578447),
 .UNSPECIFIED.)
CURVE()
GEOMETRIC_REPRESENTATION_ITEM()
RATIONAL_B_SPLINE_CURVE((1.00207919473721,1.00198318128518,1.))
REPRESENTATION_ITEM('')
) ;
#314=(
BOUNDED_CURVE()
B_SPLINE_CURVE(2,(#17971,#17972,#17973),.UNSPECIFIED.,.F.,.F.)
B_SPLINE_CURVE_WITH_KNOTS((3,3),(0.,0.0208203041102687),.UNSPECIFIED.)
CURVE()
GEOMETRIC_REPRESENTATION_ITEM()
RATIONAL_B_SPLINE_CURVE((1.,1.00198318127639,1.002079194728))
REPRESENTATION_ITEM('')
) ;
#315=(
BOUNDED_CURVE()
B_SPLINE_CURVE(2,(#17974,#17975,#17976),.UNSPECIFIED.,.F.,.F.)
B_SPLINE_CURVE_WITH_KNOTS((3,3),(0.0229388536475813,0.0437591577578468),
 .UNSPECIFIED.)
CURVE()
GEOMETRIC_REPRESENTATION_ITEM()
RATIONAL_B_SPLINE_CURVE((1.00207919473967,1.00198318128753,1.))
REPRESENTATION_ITEM('')
) ;
#316=(
BOUNDED_CURVE()
B_SPLINE_CURVE(2,(#17978,#17979,#17980),.UNSPECIFIED.,.F.,.F.)
B_SPLINE_CURVE_WITH_KNOTS((3,3),(0.,0.020820304110235),.UNSPECIFIED.)
CURVE()
GEOMETRIC_REPRESENTATION_ITEM()
RATIONAL_B_SPLINE_CURVE((1.,1.00198318129245,1.00207919474483))
REPRESENTATION_ITEM('')
) ;
#317=(
BOUNDED_CURVE()
B_SPLINE_CURVE(2,(#17981,#17982,#17983),.UNSPECIFIED.,.F.,.F.)
B_SPLINE_CURVE_WITH_KNOTS((3,3),(0.0229388536476187,0.0437591577578467),
 .UNSPECIFIED.)
CURVE()
GEOMETRIC_REPRESENTATION_ITEM()
RATIONAL_B_SPLINE_CURVE((1.00207919475315,1.00198318130038,1.))
REPRESENTATION_ITEM('')
) ;
#318=(
BOUNDED_CURVE()
B_SPLINE_CURVE(2,(#17984,#17985,#17986),.UNSPECIFIED.,.F.,.F.)
B_SPLINE_CURVE_WITH_KNOTS((3,3),(0.,0.0208203041103129),.UNSPECIFIED.)
CURVE()
GEOMETRIC_REPRESENTATION_ITEM()
RATIONAL_B_SPLINE_CURVE((1.,1.00198318126409,1.00207919471509))
REPRESENTATION_ITEM('')
) ;
#319=(
BOUNDED_CURVE()
B_SPLINE_CURVE(2,(#18234,#18235,#18236),.UNSPECIFIED.,.F.,.F.)
B_SPLINE_CURVE_WITH_KNOTS((3,3),(0.,0.0136874154102615),.UNSPECIFIED.)
CURVE()
GEOMETRIC_REPRESENTATION_ITEM()
RATIONAL_B_SPLINE_CURVE((1.,1.0066910623624,1.00897713804962))
REPRESENTATION_ITEM('')
) ;
#320=(
BOUNDED_CURVE()
B_SPLINE_CURVE(2,(#18240,#18241,#18242),.UNSPECIFIED.,.F.,.F.)
B_SPLINE_CURVE_WITH_KNOTS((3,3),(0.0278942541126724,0.0415816695229389),
 .UNSPECIFIED.)
CURVE()
GEOMETRIC_REPRESENTATION_ITEM()
RATIONAL_B_SPLINE_CURVE((1.00897713804904,1.00669106236197,1.))
REPRESENTATION_ITEM('')
) ;
#321=(
BOUNDED_CURVE()
B_SPLINE_CURVE(2,(#18244,#18245,#18246),.UNSPECIFIED.,.F.,.F.)
B_SPLINE_CURVE_WITH_KNOTS((3,3),(0.,0.0136874154102685),.UNSPECIFIED.)
CURVE()
GEOMETRIC_REPRESENTATION_ITEM()
RATIONAL_B_SPLINE_CURVE((1.,1.00669106236162,1.00897713804858))
REPRESENTATION_ITEM('')
) ;
#322=(
BOUNDED_CURVE()
B_SPLINE_CURVE(2,(#18250,#18251,#18252),.UNSPECIFIED.,.F.,.F.)
B_SPLINE_CURVE_WITH_KNOTS((3,3),(0.0278942541126688,0.0415816695229383),
 .UNSPECIFIED.)
CURVE()
GEOMETRIC_REPRESENTATION_ITEM()
RATIONAL_B_SPLINE_CURVE((1.00897713804858,1.00669106236162,1.))
REPRESENTATION_ITEM('')
) ;
#323=(
BOUNDED_CURVE()
B_SPLINE_CURVE(2,(#18254,#18255,#18256),.UNSPECIFIED.,.F.,.F.)
B_SPLINE_CURVE_WITH_KNOTS((3,3),(0.,0.0136874154102617),.UNSPECIFIED.)
CURVE()
GEOMETRIC_REPRESENTATION_ITEM()
RATIONAL_B_SPLINE_CURVE((1.,1.0066910623619,1.00897713804895))
REPRESENTATION_ITEM('')
) ;
#324=(
BOUNDED_CURVE()
B_SPLINE_CURVE(2,(#18260,#18261,#18262),.UNSPECIFIED.,.F.,.F.)
B_SPLINE_CURVE_WITH_KNOTS((3,3),(0.0278942541126742,0.0415816695229357),
 .UNSPECIFIED.)
CURVE()
GEOMETRIC_REPRESENTATION_ITEM()
RATIONAL_B_SPLINE_CURVE((1.0089771380487,1.00669106236171,1.))
REPRESENTATION_ITEM('')
) ;
#325=(
BOUNDED_CURVE()
B_SPLINE_CURVE(2,(#18264,#18265,#18266),.UNSPECIFIED.,.F.,.F.)
B_SPLINE_CURVE_WITH_KNOTS((3,3),(0.,0.0136874154102619),.UNSPECIFIED.)
CURVE()
GEOMETRIC_REPRESENTATION_ITEM()
RATIONAL_B_SPLINE_CURVE((1.,1.00669106236241,1.00897713804963))
REPRESENTATION_ITEM('')
) ;
#326=(
BOUNDED_CURVE()
B_SPLINE_CURVE(2,(#18270,#18271,#18272),.UNSPECIFIED.,.F.,.F.)
B_SPLINE_CURVE_WITH_KNOTS((3,3),(0.0278942541126735,0.0415816695229364),
 .UNSPECIFIED.)
CURVE()
GEOMETRIC_REPRESENTATION_ITEM()
RATIONAL_B_SPLINE_CURVE((1.00897713804995,1.00669106236265,1.))
REPRESENTATION_ITEM('')
) ;
#327=(
BOUNDED_CURVE()
B_SPLINE_CURVE(2,(#18274,#18275,#18276),.UNSPECIFIED.,.F.,.F.)
B_SPLINE_CURVE_WITH_KNOTS((3,3),(0.,0.0136874154102649),.UNSPECIFIED.)
CURVE()
GEOMETRIC_REPRESENTATION_ITEM()
RATIONAL_B_SPLINE_CURVE((1.,1.00669106236169,1.00897713804866))
REPRESENTATION_ITEM('')
) ;
#328=(
BOUNDED_CURVE()
B_SPLINE_CURVE(2,(#18280,#18281,#18282),.UNSPECIFIED.,.F.,.F.)
B_SPLINE_CURVE_WITH_KNOTS((3,3),(0.0278942541126746,0.0415816695229368),
 .UNSPECIFIED.)
CURVE()
GEOMETRIC_REPRESENTATION_ITEM()
RATIONAL_B_SPLINE_CURVE((1.00897713804866,1.00669106236168,1.))
REPRESENTATION_ITEM('')
) ;
#329=(
BOUNDED_CURVE()
B_SPLINE_CURVE(2,(#18284,#18285,#18286),.UNSPECIFIED.,.F.,.F.)
B_SPLINE_CURVE_WITH_KNOTS((3,3),(0.,0.0136874154102616),.UNSPECIFIED.)
CURVE()
GEOMETRIC_REPRESENTATION_ITEM()
RATIONAL_B_SPLINE_CURVE((1.,1.00669106236177,1.00897713804877))
REPRESENTATION_ITEM('')
) ;
#330=(
BOUNDED_CURVE()
B_SPLINE_CURVE(2,(#18289,#18290,#18291),.UNSPECIFIED.,.F.,.F.)
B_SPLINE_CURVE_WITH_KNOTS((3,3),(0.0278942541126769,0.0415816695229329),
 .UNSPECIFIED.)
CURVE()
GEOMETRIC_REPRESENTATION_ITEM()
RATIONAL_B_SPLINE_CURVE((1.00897713804978,1.00669106236252,1.))
REPRESENTATION_ITEM('')
) ;
#337=TOROIDAL_SURFACE('',#10309,1.06675,0.1) ;
#338=TOROIDAL_SURFACE('',#10504,1.69999999999999,0.2) ;
#352=SHAPE_REPRESENTATION_RELATIONSHIP('SRR','None',#18870,#369) ;
#369=ADVANCED_BREP_SHAPE_REPRESENTATION('',(#403),#18753) ;
#386=STYLED_ITEM('',(#18964),#403) ;
#403=MANIFOLD_SOLID_BREP('ISO 4762 - M2 x 6 - 12.9',#9555) ;
#436=B_SPLINE_CURVE_WITH_KNOTS('',3,(#15304,#15305,#15306,#15307,#15308,
#15309,#15310,#15311,#15312,#15313),.UNSPECIFIED.,.F.,.F.,(4,3,3,4),(-4.09157007060749,
-3.96642934058395,-2.97482200543796,-2.06546402602177),.UNSPECIFIED.) ;
#437=B_SPLINE_CURVE_WITH_KNOTS('',3,(#15316,#15317,#15318,#15319,#15320,
#15321,#15322),.UNSPECIFIED.,.F.,.F.,(4,3,4),(0.,0.991607335145971,1.11548660900393),
 .UNSPECIFIED.) ;
#438=B_SPLINE_CURVE_WITH_KNOTS('',3,(#15327,#15328,#15329,#15330,#15331,
#15332,#15333,#15334,#15335,#15336,#15337,#15338,#15339,#15340,#15341,#15342,
#15343,#15344,#15345,#15346,#15347,#15348),.UNSPECIFIED.,.F.,.F.,(4,3,3,
3,3,3,3,4),(-10.3747553777871,-9.91607335145986,-8.92446601631388,-7.93285868116789,
-6.94125134602191,-5.94964401087592,-4.95803667572993,-4.09157007060749),
 .UNSPECIFIED.) ;
#439=B_SPLINE_CURVE_WITH_KNOTS('',3,(#15349,#15350,#15351,#15352,#15353,
#15354,#15355,#15356,#15357,#15358,#15359,#15360,#15361,#15362,#15363,#15364,
#15365,#15366,#15367,#15368,#15369,#15370),.UNSPECIFIED.,.F.,.F.,(4,3,3,
3,3,3,3,4),(1.11548660900393,1.98321467029196,2.97482200543794,3.96642934058392,
4.95803667572991,5.94964401087589,6.94125134602187,7.39867191618352),
 .UNSPECIFIED.) ;
#440=B_SPLINE_CURVE_WITH_KNOTS('',3,(#15375,#15376,#15377,#15378,#15379,
#15380,#15381,#15382,#15383,#15384,#15385,#15386,#15387,#15388,#15389,#15390,
#15391,#15392,#15393,#15394,#15395,#15396),.UNSPECIFIED.,.F.,.F.,(4,3,3,
3,3,3,3,4),(-16.6579406849667,-15.8657173623358,-14.8741100271898,-13.8825026920438,
-12.8908953568978,-11.8992880217518,-10.9076806866059,-10.3747553777871),
 .UNSPECIFIED.) ;
#441=B_SPLINE_CURVE_WITH_KNOTS('',3,(#15397,#15398,#15399,#15400,#15401,
#15402,#15403,#15404,#15405,#15406,#15407,#15408,#15409,#15410,#15411,#15412,
#15413,#15414,#15415,#15416,#15417,#15418),.UNSPECIFIED.,.F.,.F.,(4,3,3,
3,3,3,3,4),(7.39867191618352,7.93285868116786,8.92446601631384,9.91607335145983,
10.9076806866058,11.8992880217518,12.8908953568978,13.6818572233631),
 .UNSPECIFIED.) ;
#442=B_SPLINE_CURVE_WITH_KNOTS('',3,(#15423,#15424,#15425,#15426,#15427,
#15428,#15429,#15430,#15431,#15432,#15433,#15434,#15435,#15436,#15437,#15438,
#15439,#15440,#15441,#15442,#15443,#15444,#15445,#15446,#15447),
 .UNSPECIFIED.,.F.,.F.,(4,3,3,3,3,3,3,3,4),(-22.9411259921463,-22.8069687083577,
-21.8153613732117,-20.8237540380657,-19.8321467029197,-18.8405393677737,
-17.8489320326278,-16.8573246974818,-16.6579406849667),.UNSPECIFIED.) ;
#443=B_SPLINE_CURVE_WITH_KNOTS('',3,(#15448,#15449,#15450,#15451,#15452,
#15453,#15454,#15455,#15456,#15457,#15458,#15459,#15460,#15461,#15462,#15463,
#15464,#15465,#15466,#15467,#15468,#15469,#15470,#15471,#15472),
 .UNSPECIFIED.,.F.,.F.,(4,3,3,3,3,3,3,3,4),(13.6818572233631,13.8825026920438,
14.8741100271898,15.8657173623357,16.8573246974817,17.8489320326277,18.8405393677737,
19.8321467029197,19.9650425305427),.UNSPECIFIED.) ;
#444=B_SPLINE_CURVE_WITH_KNOTS('',3,(#15477,#15478,#15479,#15480,#15481,
#15482,#15483,#15484,#15485,#15486,#15487,#15488,#15489,#15490,#15491,#15492,
#15493,#15494,#15495,#15496,#15497,#15498),.UNSPECIFIED.,.F.,.F.,(4,3,3,
3,3,3,3,4),(-29.2243112993259,-28.7566127192336,-27.7650053840876,-26.7733980489416,
-25.7817907137956,-24.7901833786497,-23.7985760435037,-22.9411259921463),
 .UNSPECIFIED.) ;
#445=B_SPLINE_CURVE_WITH_KNOTS('',3,(#15499,#15500,#15501,#15502,#15503,
#15504,#15505,#15506,#15507,#15508,#15509,#15510,#15511,#15512,#15513,#15514,
#15515,#15516,#15517,#15518,#15519,#15520),.UNSPECIFIED.,.F.,.F.,(4,3,3,
3,3,3,3,4),(19.9650425305427,20.8237540380657,21.8153613732117,22.8069687083576,
23.7985760435036,24.7901833786496,25.7817907137956,26.2482278377223),
 .UNSPECIFIED.) ;
#446=B_SPLINE_CURVE_WITH_KNOTS('',3,(#15525,#15526,#15527,#15528,#15529,
#15530,#15531,#15532,#15533,#15534,#15535,#15536,#15537,#15538,#15539,#15540,
#15541,#15542,#15543,#15544,#15545,#15546),.UNSPECIFIED.,.F.,.F.,(4,3,3,
3,3,3,3,4),(-35.5074966065054,-34.7062567301095,-33.7146493949635,-32.7230420598175,
-31.7314347246716,-30.7398273895256,-29.7482200543796,-29.2243112993259),
 .UNSPECIFIED.) ;
#447=B_SPLINE_CURVE_WITH_KNOTS('',3,(#15547,#15548,#15549,#15550,#15551,
#15552,#15553,#15554,#15555,#15556,#15557,#15558,#15559,#15560,#15561,#15562,
#15563,#15564,#15565,#15566,#15567,#15568),.UNSPECIFIED.,.F.,.F.,(4,3,3,
3,3,3,3,4),(26.2482278377223,26.7733980489416,27.7650053840876,28.7566127192336,
29.7482200543795,30.7398273895255,31.7314347246715,32.5314131449019),
 .UNSPECIFIED.) ;
#448=B_SPLINE_CURVE_WITH_KNOTS('',3,(#15573,#15574,#15575,#15576,#15577,
#15578,#15579,#15580,#15581,#15582,#15583,#15584,#15585,#15586,#15587,#15588,
#15589,#15590,#15591,#15592,#15593,#15594,#15595,#15596,#15597),
 .UNSPECIFIED.,.F.,.F.,(4,3,3,3,3,3,3,3,4),(-41.790681913685,-41.6475080761314,
-40.6559007409854,-39.6642934058394,-38.6726860706935,-37.6810787355475,
-36.6894714004015,-35.6978640652555,-35.5074966065054),.UNSPECIFIED.) ;
#449=B_SPLINE_CURVE_WITH_KNOTS('',3,(#15598,#15599,#15600,#15601,#15602,
#15603,#15604,#15605,#15606,#15607,#15608,#15609,#15610,#15611,#15612,#15613,
#15614,#15615,#15616,#15617,#15618,#15619,#15620,#15621,#15622),
 .UNSPECIFIED.,.F.,.F.,(4,3,3,3,3,3,3,3,4),(32.5314131449019,32.7230420598175,
33.7146493949635,34.7062567301095,35.6978640652555,36.6894714004015,37.6810787355474,
38.6726860706934,38.8145984520815),.UNSPECIFIED.) ;
#450=B_SPLINE_CURVE_WITH_KNOTS('',3,(#15627,#15628,#15629,#15630,#15631,
#15632,#15633,#15634,#15635,#15636,#15637,#15638,#15639,#15640,#15641,#15642,
#15643,#15644,#15645,#15646,#15647,#15648),.UNSPECIFIED.,.F.,.F.,(4,3,3,
3,3,3,3,4),(-48.0738672208646,-47.5971520870073,-46.6055447518613,-45.6139374167154,
-44.6223300815694,-43.6307227464234,-42.6391154112774,-41.790681913685),
 .UNSPECIFIED.) ;
#451=B_SPLINE_CURVE_WITH_KNOTS('',3,(#15649,#15650,#15651,#15652,#15653,
#15654,#15655,#15656,#15657,#15658,#15659,#15660,#15661,#15662,#15663,#15664,
#15665,#15666,#15667,#15668,#15669,#15670),.UNSPECIFIED.,.F.,.F.,(4,3,3,
3,3,3,3,4),(38.8145984520815,39.6642934058394,40.6559007409854,41.6475080761314,
42.6391154112774,43.6307227464233,44.6223300815693,45.0977837592611),
 .UNSPECIFIED.) ;
#452=B_SPLINE_CURVE_WITH_KNOTS('',3,(#15675,#15676,#15677,#15678,#15679,
#15680,#15681,#15682,#15683,#15684,#15685,#15686,#15687,#15688,#15689,#15690,
#15691,#15692,#15693,#15694,#15695,#15696),.UNSPECIFIED.,.F.,.F.,(4,3,3,
3,3,3,3,4),(-54.3570525280442,-53.5467960978832,-52.5551887627373,-51.5635814275913,
-50.5719740924453,-49.5803667572993,-48.5887594221533,-48.0738672208646),
 .UNSPECIFIED.) ;
#453=B_SPLINE_CURVE_WITH_KNOTS('',3,(#15697,#15698,#15699,#15700,#15701,
#15702,#15703,#15704,#15705,#15706,#15707,#15708,#15709,#15710,#15711,#15712,
#15713,#15714,#15715,#15716,#15717,#15718),.UNSPECIFIED.,.F.,.F.,(4,3,3,
3,3,3,3,4),(45.0977837592611,45.6139374167153,46.6055447518613,47.5971520870073,
48.5887594221533,49.5803667572993,50.5719740924452,51.3809690664406),
 .UNSPECIFIED.) ;
#454=B_SPLINE_CURVE_WITH_KNOTS('',3,(#15723,#15724,#15725,#15726,#15727,
#15728,#15729,#15730,#15731,#15732,#15733,#15734,#15735,#15736,#15737,#15738,
#15739,#15740,#15741,#15742,#15743,#15744,#15745,#15746,#15747),
 .UNSPECIFIED.,.F.,.F.,(4,3,3,3,3,3,3,3,4),(-60.6402378352238,-60.4880474439051,
-59.4964401087592,-58.5048327736132,-57.5132254384672,-56.5216181033212,
-55.5300107681752,-54.5384034330292,-54.3570525280442),.UNSPECIFIED.) ;
#455=B_SPLINE_CURVE_WITH_KNOTS('',3,(#15748,#15749,#15750,#15751,#15752,
#15753,#15754,#15755,#15756,#15757,#15758,#15759,#15760,#15761,#15762,#15763,
#15764,#15765,#15766,#15767,#15768,#15769,#15770,#15771,#15772),
 .UNSPECIFIED.,.F.,.F.,(4,3,3,3,3,3,3,3,4),(51.3809690664406,51.5635814275912,
52.5551887627372,53.5467960978832,54.5384034330292,55.5300107681752,56.5216181033212,
57.5132254384671,57.6641543736202),.UNSPECIFIED.) ;
#456=B_SPLINE_CURVE_WITH_KNOTS('',3,(#15777,#15778,#15779,#15780,#15781,
#15782,#15783,#15784,#15785,#15786,#15787,#15788,#15789,#15790,#15791,#15792,
#15793,#15794,#15795,#15796,#15797,#15798),.UNSPECIFIED.,.F.,.F.,(4,3,3,
3,3,3,3,4),(-66.9234231424034,-66.437691454781,-65.4460841196351,-64.4544767844891,
-63.4628694493431,-62.4712621141971,-61.4796547790511,-60.6402378352238),
 .UNSPECIFIED.) ;
#457=B_SPLINE_CURVE_WITH_KNOTS('',3,(#15799,#15800,#15801,#15802,#15803,
#15804,#15805,#15806,#15807,#15808,#15809,#15810,#15811,#15812,#15813,#15814,
#15815,#15816,#15817,#15818,#15819,#15820),.UNSPECIFIED.,.F.,.F.,(4,3,3,
3,3,3,3,4),(57.6641543736202,58.5048327736131,59.4964401087591,60.4880474439051,
61.4796547790511,62.4712621141971,63.4628694493431,63.9473396807998),
 .UNSPECIFIED.) ;
#458=B_SPLINE_CURVE_WITH_KNOTS('',3,(#15825,#15826,#15827,#15828,#15829,
#15830,#15831,#15832,#15833,#15834,#15835,#15836,#15837,#15838,#15839,#15840,
#15841,#15842,#15843,#15844,#15845,#15846),.UNSPECIFIED.,.F.,.F.,(4,3,3,
3,3,3,3,4),(-73.206608449583,-72.387335465657,-71.395728130511,-70.404120795365,
-69.412513460219,-68.420906125073,-67.429298789927,-66.9234231424034),
 .UNSPECIFIED.) ;
#459=B_SPLINE_CURVE_WITH_KNOTS('',3,(#15847,#15848,#15849,#15850,#15851,
#15852,#15853,#15854,#15855,#15856,#15857,#15858,#15859,#15860,#15861,#15862,
#15863,#15864,#15865,#15866,#15867,#15868),.UNSPECIFIED.,.F.,.F.,(4,3,3,
3,3,3,3,4),(63.9473396807998,64.454476784489,65.446084119635,66.437691454781,
67.429298789927,68.420906125073,69.412513460219,70.2305249879794),
 .UNSPECIFIED.) ;
#460=B_SPLINE_CURVE_WITH_KNOTS('',3,(#15873,#15874,#15875,#15876,#15877,
#15878,#15879,#15880,#15881,#15882,#15883,#15884,#15885,#15886,#15887,#15888,
#15889,#15890,#15891,#15892,#15893,#15894,#15895,#15896,#15897),
 .UNSPECIFIED.,.F.,.F.,(4,3,3,3,3,3,3,3,4),(-79.4897937567626,-79.3285868116789,
-78.3369794765329,-77.3453721413869,-76.3537648062409,-75.3621574710949,
-74.3705501359489,-73.3789428008029,-73.206608449583),.UNSPECIFIED.) ;
#461=B_SPLINE_CURVE_WITH_KNOTS('',3,(#15898,#15899,#15900,#15901,#15902,
#15903,#15904,#15905,#15906,#15907,#15908,#15909,#15910,#15911,#15912,#15913,
#15914,#15915,#15916,#15917,#15918,#15919,#15920,#15921,#15922),
 .UNSPECIFIED.,.F.,.F.,(4,3,3,3,3,3,3,3,4),(70.2305249879794,70.4041207953649,
71.3957281305109,72.3873354656569,73.3789428008029,74.3705501359489,75.3621574710949,
76.3537648062409,76.513710295159),.UNSPECIFIED.) ;
#462=B_SPLINE_CURVE_WITH_KNOTS('',3,(#15927,#15928,#15929,#15930,#15931,
#15932,#15933,#15934,#15935,#15936,#15937,#15938,#15939,#15940,#15941,#15942,
#15943,#15944,#15945,#15946,#15947,#15948),.UNSPECIFIED.,.F.,.F.,(4,3,3,
3,3,3,3,4),(-85.7729790639422,-85.2782308225548,-84.2866234874088,-83.2950161522628,
-82.3034088171168,-81.3118014819708,-80.3201941468249,-79.4897937567626),
 .UNSPECIFIED.) ;
#463=B_SPLINE_CURVE_WITH_KNOTS('',3,(#15949,#15950,#15951,#15952,#15953,
#15954,#15955,#15956,#15957,#15958,#15959,#15960,#15961,#15962,#15963,#15964,
#15965,#15966,#15967,#15968,#15969,#15970),.UNSPECIFIED.,.F.,.F.,(4,3,3,
3,3,3,3,4),(76.513710295159,77.3453721413868,78.3369794765328,79.3285868116788,
80.3201941468248,81.3118014819708,82.3034088171167,82.7968956023386),
 .UNSPECIFIED.) ;
#464=B_SPLINE_CURVE_WITH_KNOTS('',3,(#15976,#15977,#15978,#15979,#15980),
 .UNSPECIFIED.,.F.,.F.,(4,1,4),(97.3893722612836,97.8862313550422,98.7955893344583),
 .UNSPECIFIED.) ;
#465=B_SPLINE_CURVE_WITH_KNOTS('',3,(#15983,#15984,#15985,#15986),
 .UNSPECIFIED.,.F.,.F.,(4,4),(97.3893722612836,97.5539515149039),
 .UNSPECIFIED.) ;
#466=B_SPLINE_CURVE_WITH_KNOTS('',3,(#15991,#15992,#15993,#15994,#15995,
#15996,#15997,#15998,#15999,#16000),.UNSPECIFIED.,.F.,.F.,(4,1,1,1,1,1,
1,4),(91.106186954104,91.9365873441662,92.9281946793122,93.9198020144582,
94.9114093496042,95.9030166847502,96.8946240198962,97.3893722612836),
 .UNSPECIFIED.) ;
#467=B_SPLINE_CURVE_WITH_KNOTS('',3,(#16001,#16002,#16003,#16004,#16005,
#16006,#16007,#16008,#16009,#16010),.UNSPECIFIED.,.F.,.F.,(4,1,1,1,1,1,
1,4),(91.106186954104,91.604307504028,92.595914839174,93.58752217432,94.579129509466,
95.5707368446119,96.5623441797579,97.3893722612836),.UNSPECIFIED.) ;
#468=B_SPLINE_CURVE_WITH_KNOTS('',3,(#16015,#16016,#16017,#16018,#16019,
#16020,#16021,#16022,#16023,#16024,#16025),.UNSPECIFIED.,.F.,.F.,(4,1,1,
1,1,1,1,1,4),(84.8230016469244,84.9953359981443,85.9869433332903,86.9785506684363,
87.9701580035823,88.9617653387283,89.9533726738743,90.9449800090203,91.106186954104),
 .UNSPECIFIED.) ;
#469=B_SPLINE_CURVE_WITH_KNOTS('',3,(#16026,#16027,#16028,#16029,#16030,
#16031,#16032,#16033,#16034,#16035),.UNSPECIFIED.,.F.,.F.,(4,1,1,1,1,1,
1,4),(84.8230016469244,85.6546634931521,86.6462708282981,87.6378781634441,
88.62948549859,89.621092833736,90.612700168882,91.106186954104),
 .UNSPECIFIED.) ;
#470=B_SPLINE_CURVE_WITH_KNOTS('',3,(#16040,#16041,#16042,#16043,#16044,
#16045,#16046,#16047,#16048,#16049),.UNSPECIFIED.,.F.,.F.,(4,1,1,1,1,1,
1,4),(78.5398163397448,79.0456919872684,80.0372993224144,81.0289066575604,
82.0205139927064,83.0121213278524,84.0037286629984,84.8230016469244),
 .UNSPECIFIED.) ;
#471=B_SPLINE_CURVE_WITH_KNOTS('',3,(#16050,#16051,#16052,#16053,#16054,
#16055,#16056,#16057,#16058,#16059,#16060),.UNSPECIFIED.,.F.,.F.,(4,1,1,
1,1,1,1,1,4),(78.5398163397448,78.7134121471302,79.7050194822762,80.6966268174222,
81.6882341525682,82.6798414877141,83.6714488228601,84.6630561580061,84.8230016469244),
 .UNSPECIFIED.) ;
#472=B_SPLINE_CURVE_WITH_KNOTS('',3,(#16065,#16066,#16067,#16068,#16069,
#16070,#16071,#16072,#16073,#16074),.UNSPECIFIED.,.F.,.F.,(4,1,1,1,1,1,
1,4),(72.2566310325652,73.0960479763925,74.0876553115385,75.0792626466845,
76.0708699818305,77.0624773169765,78.0540846521224,78.5398163397448),
 .UNSPECIFIED.) ;
#473=B_SPLINE_CURVE_WITH_KNOTS('',3,(#16075,#16076,#16077,#16078,#16079,
#16080,#16081,#16082,#16083,#16084),.UNSPECIFIED.,.F.,.F.,(4,1,1,1,1,1,
1,4),(72.2566310325652,72.7637681362543,73.7553754714003,74.7469828065463,
75.7385901416922,76.7301974768382,77.7218048119842,78.5398163397448),
 .UNSPECIFIED.) ;
#474=B_SPLINE_CURVE_WITH_KNOTS('',3,(#16089,#16090,#16091,#16092,#16093,
#16094,#16095,#16096,#16097,#16098,#16099),.UNSPECIFIED.,.F.,.F.,(4,1,1,
1,1,1,1,1,4),(65.9734457253856,66.1547966303706,67.1464039655166,68.1380113006626,
69.1296186358086,70.1212259709546,71.1128333061005,72.1044406412465,72.2566310325652),
 .UNSPECIFIED.) ;
#475=B_SPLINE_CURVE_WITH_KNOTS('',3,(#16100,#16101,#16102,#16103,#16104,
#16105,#16106,#16107,#16108,#16109),.UNSPECIFIED.,.F.,.F.,(4,1,1,1,1,1,
1,4),(65.9734457253856,66.8141241253784,67.8057314605244,68.7973387956703,
69.7889461308163,70.7805534659623,71.7721608011083,72.2566310325652),
 .UNSPECIFIED.) ;
#476=B_SPLINE_CURVE_WITH_KNOTS('',3,(#16114,#16115,#16116,#16117,#16118,
#16119,#16120,#16121,#16122,#16123),.UNSPECIFIED.,.F.,.F.,(4,1,1,1,1,1,
1,4),(59.690260418206,60.2051526194947,61.1967599546407,62.1883672897867,
63.1799746249327,64.1715819600786,65.1631892952246,65.9734457253856),
 .UNSPECIFIED.) ;
#477=B_SPLINE_CURVE_WITH_KNOTS('',3,(#16124,#16125,#16126,#16127,#16128,
#16129,#16130,#16131,#16132,#16133,#16134),.UNSPECIFIED.,.F.,.F.,(4,1,1,
1,1,1,1,1,4),(59.690260418206,59.8728727793565,60.8644801145025,61.8560874496484,
62.8476947847944,63.8393021199404,64.8309094550864,65.8225167902324,65.9734457253856),
 .UNSPECIFIED.) ;
#478=B_SPLINE_CURVE_WITH_KNOTS('',3,(#16139,#16140,#16141,#16142,#16143,
#16144,#16145,#16146,#16147,#16148),.UNSPECIFIED.,.F.,.F.,(4,1,1,1,1,1,
1,4),(53.4070751110264,54.2555086086188,55.2471159437648,56.2387232789108,
57.2303306140567,58.2219379492027,59.2135452843487,59.690260418206),
 .UNSPECIFIED.) ;
#479=B_SPLINE_CURVE_WITH_KNOTS('',3,(#16149,#16150,#16151,#16152,#16153,
#16154,#16155,#16156,#16157,#16158),.UNSPECIFIED.,.F.,.F.,(4,1,1,1,1,1,
1,4),(53.4070751110264,53.9232287684806,54.9148361036265,55.9064434387725,
56.8980507739185,57.8896581090645,58.8812654442105,59.690260418206),
 .UNSPECIFIED.) ;
#480=B_SPLINE_CURVE_WITH_KNOTS('',3,(#16163,#16164,#16165,#16166,#16167,
#16168,#16169,#16170,#16171,#16172,#16173),.UNSPECIFIED.,.F.,.F.,(4,1,1,
1,1,1,1,1,4),(47.1238898038468,47.3142572625969,48.3058645977429,49.2974719328889,
50.2890792680348,51.2806866031808,52.2722939383268,53.2639012734728,53.4070751110264),
 .UNSPECIFIED.) ;
#481=B_SPLINE_CURVE_WITH_KNOTS('',3,(#16174,#16175,#16176,#16177,#16178,
#16179,#16180,#16181,#16182,#16183),.UNSPECIFIED.,.F.,.F.,(4,1,1,1,1,1,
1,4),(47.1238898038469,47.9735847576047,48.9651920927506,49.9567994278966,
50.9484067630426,51.9400140981886,52.9316214333346,53.4070751110264),
 .UNSPECIFIED.) ;
#482=B_SPLINE_CURVE_WITH_KNOTS('',3,(#16188,#16189,#16190,#16191,#16192,
#16193,#16194,#16195,#16196,#16197),.UNSPECIFIED.,.F.,.F.,(4,1,1,1,1,1,
1,4),(40.8407044966673,41.364613251721,42.356220586867,43.3478279220129,
44.3394352571589,45.3310425923049,46.3226499274509,47.1238898038468),
 .UNSPECIFIED.) ;
#483=B_SPLINE_CURVE_WITH_KNOTS('',3,(#16198,#16199,#16200,#16201,#16202,
#16203,#16204,#16205,#16206,#16207,#16208),.UNSPECIFIED.,.F.,.F.,(4,1,1,
1,1,1,1,1,4),(40.8407044966673,41.0323334115828,42.0239407467287,43.0155480818747,
44.0071554170207,44.9987627521667,45.9903700873127,46.9819774224587,47.1238898038469),
 .UNSPECIFIED.) ;
#484=B_SPLINE_CURVE_WITH_KNOTS('',3,(#16213,#16214,#16215,#16216,#16217,
#16218,#16219,#16220,#16221,#16222),.UNSPECIFIED.,.F.,.F.,(4,1,1,1,1,1,
1,4),(34.5575191894877,35.4149692408451,36.406576575991,37.398183911137,
38.389791246283,39.381398581429,40.373005916575,40.8407044966673),
 .UNSPECIFIED.) ;
#485=B_SPLINE_CURVE_WITH_KNOTS('',3,(#16223,#16224,#16225,#16226,#16227,
#16228,#16229,#16230,#16231,#16232),.UNSPECIFIED.,.F.,.F.,(4,1,1,1,1,1,
1,4),(34.5575191894877,35.0826894007068,36.0742967358528,37.0659040709988,
38.0575114061448,39.0491187412908,40.0407260764368,40.8407044966673),
 .UNSPECIFIED.) ;
#486=B_SPLINE_CURVE_WITH_KNOTS('',3,(#16237,#16238,#16239,#16240,#16241,
#16242,#16243,#16244,#16245,#16246,#16247),.UNSPECIFIED.,.F.,.F.,(4,1,1,
1,1,1,1,1,4),(28.2743338823081,28.4737178948232,29.4653252299691,30.4569325651151,
31.4485399002611,32.4401472354071,33.4317545705531,34.4233619056991,34.5575191894877),
 .UNSPECIFIED.) ;
#487=B_SPLINE_CURVE_WITH_KNOTS('',3,(#16248,#16249,#16250,#16251,#16252,
#16253,#16254,#16255,#16256,#16257),.UNSPECIFIED.,.F.,.F.,(4,1,1,1,1,1,
1,4),(28.2743338823081,29.1330453898309,30.1246527249769,31.1162600601229,
32.1078673952689,33.0994747304149,34.0910820655609,34.5575191894877),
 .UNSPECIFIED.) ;
#488=B_SPLINE_CURVE_WITH_KNOTS('',3,(#16262,#16263,#16264,#16265,#16266,
#16267,#16268,#16269,#16270,#16271),.UNSPECIFIED.,.F.,.F.,(4,1,1,1,1,1,
1,4),(21.9911485751285,22.5240738839472,23.5156812190932,24.5072885542392,
25.4988958893852,26.4905032245312,27.4821105596772,28.2743338823081),
 .UNSPECIFIED.) ;
#489=B_SPLINE_CURVE_WITH_KNOTS('',3,(#16272,#16273,#16274,#16275,#16276,
#16277,#16278,#16279,#16280,#16281,#16282),.UNSPECIFIED.,.F.,.F.,(4,1,1,
1,1,1,1,1,4),(21.9911485751285,22.191794043809,23.183401378955,24.175008714101,
25.166616049247,26.158223384393,27.149830719539,28.1414380546849,28.2743338823081),
 .UNSPECIFIED.) ;
#490=B_SPLINE_CURVE_WITH_KNOTS('',3,(#16287,#16288,#16289,#16290,#16291,
#16292,#16293,#16294,#16295,#16296),.UNSPECIFIED.,.F.,.F.,(4,1,1,1,1,1,
1,4),(15.7079632679489,16.5744298730713,17.5660372082173,18.5576445433633,
19.5492518785093,20.5408592136553,21.5324665488013,21.9911485751285),
 .UNSPECIFIED.) ;
#491=B_SPLINE_CURVE_WITH_KNOTS('',3,(#16297,#16298,#16299,#16300,#16301,
#16302,#16303,#16304,#16305,#16306),.UNSPECIFIED.,.F.,.F.,(4,1,1,1,1,1,
1,4),(15.7079632679489,16.2421500329331,17.2337573680791,18.2253647032251,
19.2169720383711,20.2085793735171,21.200186708663,21.9911485751285),
 .UNSPECIFIED.) ;
#492=B_SPLINE_CURVE_WITH_KNOTS('',3,(#16309,#16310,#16311,#16312,#16313,
#16314,#16315,#16316,#16317,#16318,#16319,#16320,#16321,#16322,#16323,#16324,
#16325,#16326,#16327,#16328,#16329,#16330,#16331,#16332,#16333,#16334,#16335,
#16336,#16337,#16338,#16339,#16340,#16341,#16342,#16343,#16344,#16345,#16346,
#16347,#16348,#16349,#16350,#16351,#16352,#16353,#16354,#16355,#16356,#16357,
#16358,#16359,#16360,#16361,#16362,#16363,#16364,#16365,#16366,#16367,#16368,
#16369,#16370,#16371,#16372,#16373,#16374,#16375,#16376,#16377,#16378,#16379,
#16380,#16381),.UNSPECIFIED.,.F.,.F.,(4,3,3,3,3,3,3,3,3,3,3,3,3,3,3,3,3,
3,3,3,3,3,3,3,4),(-0.178587760439521,-0.172368112300629,-0.16226114537578,
-0.159089326739945,-0.156380108469748,-0.145604887663453,-0.13783812866639,
-0.135347956754248,-0.124003881288268,-0.112570095034531,-0.10661697955651,
-0.103666068884657,-0.0915123769018346,-0.0800733297891053,-0.0748448030148055,
-0.0719656171109528,-0.0694981620716388,-0.0575365254690618,-0.0452971625704305,
-0.0394202376900176,-0.0367681760664848,-0.0343241134637728,-0.0216317222431062,
-0.00902515542907539,0.),.UNSPECIFIED.) ;
#493=B_SPLINE_CURVE_WITH_KNOTS('',3,(#16386,#16387,#16388,#16389,#16390,
#16391,#16392,#16393,#16394,#16395,#16396,#16397,#16398,#16399,#16400,#16401,
#16402,#16403,#16404,#16405,#16406,#16407,#16408,#16409,#16410,#16411,#16412,
#16413,#16414,#16415,#16416,#16417,#16418,#16419,#16420,#16421,#16422,#16423,
#16424,#16425,#16426,#16427,#16428,#16429,#16430,#16431,#16432,#16433,#16434,
#16435,#16436,#16437,#16438,#16439,#16440,#16441,#16442,#16443,#16444,#16445,
#16446,#16447,#16448,#16449,#16450,#16451,#16452,#16453,#16454,#16455,#16456,
#16457,#16458,#16459,#16460,#16461),.UNSPECIFIED.,.F.,.F.,(4,3,3,3,3,3,
3,3,3,3,3,3,3,3,3,3,3,3,3,3,3,3,3,3,3,4),(-0.177567088092163,-0.169632484827244,
-0.158377014174832,-0.153923063489389,-0.149911964322871,-0.137452002442653,
-0.130219092088315,-0.127499132385944,-0.124937415025536,-0.112988182342971,
-0.101315560244917,-0.0957061865006923,-0.0929123724549286,-0.0906079023280744,
-0.0795887196079492,-0.0692772955064041,-0.0637952726223527,-0.0610743545148113,
-0.0587576989570135,-0.0475705807832961,-0.0365043130610792,-0.0315369939310658,
-0.0291564773895128,-0.0185494534857471,-0.00832706897214829,0.),
 .UNSPECIFIED.) ;
#494=B_SPLINE_CURVE_WITH_KNOTS('',3,(#16834,#16835,#16836,#16837,#16838,
#16839,#16840,#16841,#16842,#16843,#16844,#16845,#16846,#16847,#16848,#16849),
 .UNSPECIFIED.,.F.,.F.,(4,3,3,3,3,4),(82.7968956023386,83.2950161522627,
84.2866234874087,85.2782308225547,86.2698381577007,87.1791961371168),
 .UNSPECIFIED.) ;
#495=B_SPLINE_CURVE_WITH_KNOTS('',3,(#16851,#16852,#16853,#16854,#16855,
#16856,#16857,#16858,#16859,#16860,#16861,#16862,#16863,#16864,#16865,#16866,
#16867,#16868,#16869,#16870,#16871,#16872,#16873,#16874,#16875,#16876,#16877,
#16878,#16879,#16880,#16881,#16882,#16883,#16884,#16885,#16886,#16887,#16888,
#16889,#16890,#16891,#16892,#16893,#16894,#16895,#16896,#16897,#16898,#16899,
#16900,#16901,#16902,#16903,#16904,#16905,#16906,#16907,#16908,#16909,#16910,
#16911,#16912,#16913,#16914,#16915,#16916,#16917,#16918,#16919,#16920,#16921,
#16922,#16923),.UNSPECIFIED.,.F.,.F.,(4,3,3,3,3,3,3,3,3,3,3,3,3,3,3,3,3,
3,3,3,3,3,3,3,4),(-0.178587760439465,-0.17236811230058,-0.162261145375735,
-0.159089326536153,-0.156380108199469,-0.145604886686803,-0.137838126692299,
-0.135347954859556,-0.124003879153533,-0.112570093018921,-0.106616976888393,
-0.10366606834618,-0.0915123769018256,-0.0800733297890974,-0.0748448032652592,
-0.0719656187257878,-0.0694981625144281,-0.0575365255268622,-0.0452971622355605,
-0.0394202373519763,-0.0367681765917414,-0.0343241136941139,-0.0216317221625266,
-0.00902515635034675,0.),.UNSPECIFIED.) ;
#496=B_SPLINE_CURVE_WITH_KNOTS('',3,(#16924,#16925,#16926,#16927,#16928,
#16929,#16930,#16931,#16932),.UNSPECIFIED.,.F.,.F.,(4,1,1,1,1,1,4),(10.374755377787,
11.2841133572032,12.2757206923492,13.2673280274952,14.2589353626411,15.2505426977871,
15.7079632679489),.UNSPECIFIED.) ;
#497=B_SPLINE_CURVE_WITH_KNOTS('',3,(#16937,#16938,#16939,#16940,#16941,
#16942,#16943,#16944,#16945,#16946,#16947,#16948,#16949,#16950,#16951,#16952,
#16953,#16954,#16955,#16956,#16957,#16958,#16959,#16960,#16961,#16962,#16963,
#16964,#16965,#16966,#16967,#16968,#16969,#16970,#16971,#16972,#16973,#16974,
#16975,#16976,#16977,#16978,#16979,#16980,#16981,#16982,#16983,#16984,#16985,
#16986,#16987,#16988,#16989,#16990,#16991,#16992,#16993,#16994,#16995,#16996,
#16997,#16998,#16999,#17000,#17001,#17002,#17003,#17004,#17005,#17006,#17007,
#17008,#17009,#17010,#17011,#17012),.UNSPECIFIED.,.F.,.F.,(4,3,3,3,3,3,
3,3,3,3,3,3,3,3,3,3,3,3,3,3,3,3,3,3,3,4),(-0.177567088092174,-0.169632484827252,
-0.158377014174843,-0.153923063868584,-0.149911964428064,-0.13745200265245,
-0.130219092271891,-0.127499133676989,-0.124937417107909,-0.11298818500665,
-0.101315564042759,-0.0957061909767678,-0.0929123852241928,-0.0906079053022808,
-0.0795887196079767,-0.069277289277766,-0.0637952645839567,-0.0610743506682683,
-0.0587576970945015,-0.0475705789278521,-0.0365043101748255,-0.0315369900305327,
-0.0291564755179297,-0.0185494505299689,-0.00832706430112883,0.),
 .UNSPECIFIED.) ;
#498=B_SPLINE_CURVE_WITH_KNOTS('',3,(#17016,#17017,#17018,#17019,#17020,
#17021,#17022,#17023),.UNSPECIFIED.,.F.,.F.,(4,1,1,1,1,4),(11.6163931973414,
12.6080005324874,13.5996078676334,14.5912152027794,15.5828225379253,15.7079632679489),
 .UNSPECIFIED.) ;
#499=B_SPLINE_CURVE_WITH_KNOTS('',3,(#17396,#17397,#17398,#17399,#17400,
#17401,#17402,#17403,#17404,#17405,#17406,#17407,#17408),.UNSPECIFIED.,
 .F.,.F.,(4,3,3,3,4),(-89.2446601631387,-88.2530528279927,-87.2614454928467,
-86.2698381577008,-85.7729790639422),.UNSPECIFIED.) ;
#596=CYLINDRICAL_SURFACE('',#10271,0.96675) ;
#597=CYLINDRICAL_SURFACE('',#10273,0.96675) ;
#598=CYLINDRICAL_SURFACE('',#10274,0.96675) ;
#599=CYLINDRICAL_SURFACE('',#10275,0.96675) ;
#600=CYLINDRICAL_SURFACE('',#10276,0.96675) ;
#601=CYLINDRICAL_SURFACE('',#10277,0.96675) ;
#602=CYLINDRICAL_SURFACE('',#10278,0.96675) ;
#603=CYLINDRICAL_SURFACE('',#10279,0.96675) ;
#604=CYLINDRICAL_SURFACE('',#10280,0.96675) ;
#605=CYLINDRICAL_SURFACE('',#10281,0.96675) ;
#606=CYLINDRICAL_SURFACE('',#10282,0.96675) ;
#607=CYLINDRICAL_SURFACE('',#10283,0.96675) ;
#608=CYLINDRICAL_SURFACE('',#10284,0.96675) ;
#609=CYLINDRICAL_SURFACE('',#10285,0.96675) ;
#610=CYLINDRICAL_SURFACE('',#10286,0.739000000000001) ;
#611=CYLINDRICAL_SURFACE('',#10288,0.739000000000001) ;
#612=CYLINDRICAL_SURFACE('',#10289,0.739000000000001) ;
#613=CYLINDRICAL_SURFACE('',#10290,0.739000000000001) ;
#614=CYLINDRICAL_SURFACE('',#10291,0.739000000000001) ;
#615=CYLINDRICAL_SURFACE('',#10292,0.739000000000001) ;
#616=CYLINDRICAL_SURFACE('',#10293,0.739000000000001) ;
#617=CYLINDRICAL_SURFACE('',#10294,0.739000000000001) ;
#618=CYLINDRICAL_SURFACE('',#10295,0.739000000000001) ;
#619=CYLINDRICAL_SURFACE('',#10296,0.739000000000001) ;
#620=CYLINDRICAL_SURFACE('',#10297,0.739000000000001) ;
#621=CYLINDRICAL_SURFACE('',#10298,0.739000000000001) ;
#622=CYLINDRICAL_SURFACE('',#10299,0.739000000000001) ;
#623=CYLINDRICAL_SURFACE('',#10300,0.739000000000001) ;
#624=CYLINDRICAL_SURFACE('',#10308,0.739000000000001) ;
#625=CYLINDRICAL_SURFACE('',#10312,0.96675) ;
#626=CYLINDRICAL_SURFACE('',#10323,1.9) ;
#627=CYLINDRICAL_SURFACE('',#10515,0.816025403784444) ;
#628=CYLINDRICAL_SURFACE('',#10517,0.816025403784444) ;
#629=CYLINDRICAL_SURFACE('',#10519,0.816025403784444) ;
#630=CYLINDRICAL_SURFACE('',#10521,0.816025403784444) ;
#631=CYLINDRICAL_SURFACE('',#10523,0.816025403784444) ;
#632=CYLINDRICAL_SURFACE('',#10525,0.816025403784444) ;
#733=FACE_BOUND('',#2009,.T.) ;
#734=FACE_BOUND('',#2124,.T.) ;
#920=PLANE('',#10301) ;
#921=PLANE('',#10304) ;
#922=PLANE('',#10314) ;
#923=PLANE('',#10318) ;
#924=PLANE('',#10319) ;
#925=PLANE('',#10321) ;
#926=PLANE('',#10322) ;
#927=PLANE('',#10397) ;
#928=PLANE('',#10398) ;
#929=PLANE('',#10399) ;
#930=PLANE('',#10402) ;
#931=PLANE('',#10403) ;
#932=PLANE('',#10404) ;
#933=PLANE('',#10405) ;
#934=PLANE('',#10406) ;
#935=PLANE('',#10407) ;
#936=PLANE('',#10408) ;
#937=PLANE('',#10409) ;
#938=PLANE('',#10410) ;
#939=PLANE('',#10411) ;
#940=PLANE('',#10412) ;
#941=PLANE('',#10413) ;
#942=PLANE('',#10414) ;
#943=PLANE('',#10415) ;
#944=PLANE('',#10416) ;
#945=PLANE('',#10417) ;
#946=PLANE('',#10418) ;
#947=PLANE('',#10419) ;
#948=PLANE('',#10420) ;
#949=PLANE('',#10421) ;
#950=PLANE('',#10422) ;
#951=PLANE('',#10423) ;
#952=PLANE('',#10424) ;
#953=PLANE('',#10425) ;
#954=PLANE('',#10426) ;
#955=PLANE('',#10427) ;
#956=PLANE('',#10428) ;
#957=PLANE('',#10429) ;
#958=PLANE('',#10430) ;
#959=PLANE('',#10431) ;
#960=PLANE('',#10432) ;
#961=PLANE('',#10433) ;
#962=PLANE('',#10434) ;
#963=PLANE('',#10435) ;
#964=PLANE('',#10436) ;
#965=PLANE('',#10437) ;
#966=PLANE('',#10438) ;
#967=PLANE('',#10439) ;
#968=PLANE('',#10440) ;
#969=PLANE('',#10441) ;
#970=PLANE('',#10442) ;
#971=PLANE('',#10443) ;
#972=PLANE('',#10444) ;
#973=PLANE('',#10445) ;
#974=PLANE('',#10446) ;
#975=PLANE('',#10447) ;
#976=PLANE('',#10448) ;
#977=PLANE('',#10449) ;
#978=PLANE('',#10450) ;
#979=PLANE('',#10451) ;
#980=PLANE('',#10452) ;
#981=PLANE('',#10453) ;
#982=PLANE('',#10454) ;
#983=PLANE('',#10455) ;
#984=PLANE('',#10456) ;
#985=PLANE('',#10457) ;
#986=PLANE('',#10458) ;
#987=PLANE('',#10459) ;
#988=PLANE('',#10460) ;
#989=PLANE('',#10461) ;
#990=PLANE('',#10462) ;
#991=PLANE('',#10463) ;
#992=PLANE('',#10464) ;
#993=PLANE('',#10465) ;
#994=PLANE('',#10466) ;
#995=PLANE('',#10467) ;
#996=PLANE('',#10468) ;
#997=PLANE('',#10469) ;
#998=PLANE('',#10470) ;
#999=PLANE('',#10471) ;
#1000=PLANE('',#10472) ;
#1001=PLANE('',#10473) ;
#1002=PLANE('',#10474) ;
#1003=PLANE('',#10475) ;
#1004=PLANE('',#10476) ;
#1005=PLANE('',#10477) ;
#1006=PLANE('',#10478) ;
#1007=PLANE('',#10479) ;
#1008=PLANE('',#10480) ;
#1009=PLANE('',#10481) ;
#1010=PLANE('',#10482) ;
#1011=PLANE('',#10483) ;
#1012=PLANE('',#10484) ;
#1013=PLANE('',#10485) ;
#1014=PLANE('',#10486) ;
#1015=PLANE('',#10487) ;
#1016=PLANE('',#10488) ;
#1017=PLANE('',#10489) ;
#1018=PLANE('',#10490) ;
#1019=PLANE('',#10491) ;
#1020=PLANE('',#10492) ;
#1021=PLANE('',#10493) ;
#1022=PLANE('',#10494) ;
#1023=PLANE('',#10495) ;
#1024=PLANE('',#10496) ;
#1025=PLANE('',#10497) ;
#1026=PLANE('',#10498) ;
#1027=PLANE('',#10499) ;
#1028=PLANE('',#10500) ;
#1029=PLANE('',#10501) ;
#1030=PLANE('',#10502) ;
#1031=PLANE('',#10503) ;
#1032=PLANE('',#10506) ;
#1033=PLANE('',#10527) ;
#1034=PLANE('',#10528) ;
#1035=PLANE('',#10529) ;
#1036=PLANE('',#10530) ;
#1037=PLANE('',#10531) ;
#1038=PLANE('',#10532) ;
#1039=PLANE('',#10533) ;
#1040=PLANE('',#10534) ;
#1041=PLANE('',#10535) ;
#1042=PLANE('',#10536) ;
#1043=PLANE('',#10538) ;
#1044=PLANE('',#10540) ;
#1045=PLANE('',#10542) ;
#1046=PLANE('',#10544) ;
#1047=PLANE('',#10546) ;
#1048=PLANE('',#10549) ;
#1049=PLANE('',#10550) ;
#1050=PLANE('',#10551) ;
#1372=FACE_OUTER_BOUND('',#1973,.T.) ;
#1373=FACE_OUTER_BOUND('',#1974,.T.) ;
#1374=FACE_OUTER_BOUND('',#1975,.T.) ;
#1375=FACE_OUTER_BOUND('',#1976,.T.) ;
#1376=FACE_OUTER_BOUND('',#1977,.T.) ;
#1377=FACE_OUTER_BOUND('',#1978,.T.) ;
#1378=FACE_OUTER_BOUND('',#1979,.T.) ;
#1379=FACE_OUTER_BOUND('',#1980,.T.) ;
#1380=FACE_OUTER_BOUND('',#1981,.T.) ;
#1381=FACE_OUTER_BOUND('',#1982,.T.) ;
#1382=FACE_OUTER_BOUND('',#1983,.T.) ;
#1383=FACE_OUTER_BOUND('',#1984,.T.) ;
#1384=FACE_OUTER_BOUND('',#1985,.T.) ;
#1385=FACE_OUTER_BOUND('',#1986,.T.) ;
#1386=FACE_OUTER_BOUND('',#1987,.T.) ;
#1387=FACE_OUTER_BOUND('',#1988,.T.) ;
#1388=FACE_OUTER_BOUND('',#1989,.T.) ;
#1389=FACE_OUTER_BOUND('',#1990,.T.) ;
#1390=FACE_OUTER_BOUND('',#1991,.T.) ;
#1391=FACE_OUTER_BOUND('',#1992,.T.) ;
#1392=FACE_OUTER_BOUND('',#1993,.T.) ;
#1393=FACE_OUTER_BOUND('',#1994,.T.) ;
#1394=FACE_OUTER_BOUND('',#1995,.T.) ;
#1395=FACE_OUTER_BOUND('',#1996,.T.) ;
#1396=FACE_OUTER_BOUND('',#1997,.T.) ;
#1397=FACE_OUTER_BOUND('',#1998,.T.) ;
#1398=FACE_OUTER_BOUND('',#1999,.T.) ;
#1399=FACE_OUTER_BOUND('',#2000,.T.) ;
#1400=FACE_OUTER_BOUND('',#2001,.T.) ;
#1401=FACE_OUTER_BOUND('',#2002,.T.) ;
#1402=FACE_OUTER_BOUND('',#2003,.T.) ;
#1403=FACE_OUTER_BOUND('',#2004,.T.) ;
#1404=FACE_OUTER_BOUND('',#2005,.T.) ;
#1405=FACE_OUTER_BOUND('',#2006,.T.) ;
#1406=FACE_OUTER_BOUND('',#2007,.T.) ;
#1407=FACE_OUTER_BOUND('',#2008,.T.) ;
#1408=FACE_OUTER_BOUND('',#2010,.T.) ;
#1409=FACE_OUTER_BOUND('',#2011,.T.) ;
#1410=FACE_OUTER_BOUND('',#2012,.T.) ;
#1411=FACE_OUTER_BOUND('',#2013,.T.) ;
#1412=FACE_OUTER_BOUND('',#2014,.T.) ;
#1413=FACE_OUTER_BOUND('',#2015,.T.) ;
#1414=FACE_OUTER_BOUND('',#2016,.T.) ;
#1415=FACE_OUTER_BOUND('',#2017,.T.) ;
#1416=FACE_OUTER_BOUND('',#2018,.T.) ;
#1417=FACE_OUTER_BOUND('',#2019,.T.) ;
#1418=FACE_OUTER_BOUND('',#2020,.T.) ;
#1419=FACE_OUTER_BOUND('',#2021,.T.) ;
#1420=FACE_OUTER_BOUND('',#2022,.T.) ;
#1421=FACE_OUTER_BOUND('',#2023,.T.) ;
#1422=FACE_OUTER_BOUND('',#2024,.T.) ;
#1423=FACE_OUTER_BOUND('',#2025,.T.) ;
#1424=FACE_OUTER_BOUND('',#2026,.T.) ;
#1425=FACE_OUTER_BOUND('',#2027,.T.) ;
#1426=FACE_OUTER_BOUND('',#2028,.T.) ;
#1427=FACE_OUTER_BOUND('',#2029,.T.) ;
#1428=FACE_OUTER_BOUND('',#2030,.T.) ;
#1429=FACE_OUTER_BOUND('',#2031,.T.) ;
#1430=FACE_OUTER_BOUND('',#2032,.T.) ;
#1431=FACE_OUTER_BOUND('',#2033,.T.) ;
#1432=FACE_OUTER_BOUND('',#2034,.T.) ;
#1433=FACE_OUTER_BOUND('',#2035,.T.) ;
#1434=FACE_OUTER_BOUND('',#2036,.T.) ;
#1435=FACE_OUTER_BOUND('',#2037,.T.) ;
#1436=FACE_OUTER_BOUND('',#2038,.T.) ;
#1437=FACE_OUTER_BOUND('',#2039,.T.) ;
#1438=FACE_OUTER_BOUND('',#2040,.T.) ;
#1439=FACE_OUTER_BOUND('',#2041,.T.) ;
#1440=FACE_OUTER_BOUND('',#2042,.T.) ;
#1441=FACE_OUTER_BOUND('',#2043,.T.) ;
#1442=FACE_OUTER_BOUND('',#2044,.T.) ;
#1443=FACE_OUTER_BOUND('',#2045,.T.) ;
#1444=FACE_OUTER_BOUND('',#2046,.T.) ;
#1445=FACE_OUTER_BOUND('',#2047,.T.) ;
#1446=FACE_OUTER_BOUND('',#2048,.T.) ;
#1447=FACE_OUTER_BOUND('',#2049,.T.) ;
#1448=FACE_OUTER_BOUND('',#2050,.T.) ;
#1449=FACE_OUTER_BOUND('',#2051,.T.) ;
#1450=FACE_OUTER_BOUND('',#2052,.T.) ;
#1451=FACE_OUTER_BOUND('',#2053,.T.) ;
#1452=FACE_OUTER_BOUND('',#2054,.T.) ;
#1453=FACE_OUTER_BOUND('',#2055,.T.) ;
#1454=FACE_OUTER_BOUND('',#2056,.T.) ;
#1455=FACE_OUTER_BOUND('',#2057,.T.) ;
#1456=FACE_OUTER_BOUND('',#2058,.T.) ;
#1457=FACE_OUTER_BOUND('',#2059,.T.) ;
#1458=FACE_OUTER_BOUND('',#2060,.T.) ;
#1459=FACE_OUTER_BOUND('',#2061,.T.) ;
#1460=FACE_OUTER_BOUND('',#2062,.T.) ;
#1461=FACE_OUTER_BOUND('',#2063,.T.) ;
#1462=FACE_OUTER_BOUND('',#2064,.T.) ;
#1463=FACE_OUTER_BOUND('',#2065,.T.) ;
#1464=FACE_OUTER_BOUND('',#2066,.T.) ;
#1465=FACE_OUTER_BOUND('',#2067,.T.) ;
#1466=FACE_OUTER_BOUND('',#2068,.T.) ;
#1467=FACE_OUTER_BOUND('',#2069,.T.) ;
#1468=FACE_OUTER_BOUND('',#2070,.T.) ;
#1469=FACE_OUTER_BOUND('',#2071,.T.) ;
#1470=FACE_OUTER_BOUND('',#2072,.T.) ;
#1471=FACE_OUTER_BOUND('',#2073,.T.) ;
#1472=FACE_OUTER_BOUND('',#2074,.T.) ;
#1473=FACE_OUTER_BOUND('',#2075,.T.) ;
#1474=FACE_OUTER_BOUND('',#2076,.T.) ;
#1475=FACE_OUTER_BOUND('',#2077,.T.) ;
#1476=FACE_OUTER_BOUND('',#2078,.T.) ;
#1477=FACE_OUTER_BOUND('',#2079,.T.) ;
#1478=FACE_OUTER_BOUND('',#2080,.T.) ;
#1479=FACE_OUTER_BOUND('',#2081,.T.) ;
#1480=FACE_OUTER_BOUND('',#2082,.T.) ;
#1481=FACE_OUTER_BOUND('',#2083,.T.) ;
#1482=FACE_OUTER_BOUND('',#2084,.T.) ;
#1483=FACE_OUTER_BOUND('',#2085,.T.) ;
#1484=FACE_OUTER_BOUND('',#2086,.T.) ;
#1485=FACE_OUTER_BOUND('',#2087,.T.) ;
#1486=FACE_OUTER_BOUND('',#2088,.T.) ;
#1487=FACE_OUTER_BOUND('',#2089,.T.) ;
#1488=FACE_OUTER_BOUND('',#2090,.T.) ;
#1489=FACE_OUTER_BOUND('',#2091,.T.) ;
#1490=FACE_OUTER_BOUND('',#2092,.T.) ;
#1491=FACE_OUTER_BOUND('',#2093,.T.) ;
#1492=FACE_OUTER_BOUND('',#2094,.T.) ;
#1493=FACE_OUTER_BOUND('',#2095,.T.) ;
#1494=FACE_OUTER_BOUND('',#2096,.T.) ;
#1495=FACE_OUTER_BOUND('',#2097,.T.) ;
#1496=FACE_OUTER_BOUND('',#2098,.T.) ;
#1497=FACE_OUTER_BOUND('',#2099,.T.) ;
#1498=FACE_OUTER_BOUND('',#2100,.T.) ;
#1499=FACE_OUTER_BOUND('',#2101,.T.) ;
#1500=FACE_OUTER_BOUND('',#2102,.T.) ;
#1501=FACE_OUTER_BOUND('',#2103,.T.) ;
#1502=FACE_OUTER_BOUND('',#2104,.T.) ;
#1503=FACE_OUTER_BOUND('',#2105,.T.) ;
#1504=FACE_OUTER_BOUND('',#2106,.T.) ;
#1505=FACE_OUTER_BOUND('',#2107,.T.) ;
#1506=FACE_OUTER_BOUND('',#2108,.T.) ;
#1507=FACE_OUTER_BOUND('',#2109,.T.) ;
#1508=FACE_OUTER_BOUND('',#2110,.T.) ;
#1509=FACE_OUTER_BOUND('',#2111,.T.) ;
#1510=FACE_OUTER_BOUND('',#2112,.T.) ;
#1511=FACE_OUTER_BOUND('',#2113,.T.) ;
#1512=FACE_OUTER_BOUND('',#2114,.T.) ;
#1513=FACE_OUTER_BOUND('',#2115,.T.) ;
#1514=FACE_OUTER_BOUND('',#2116,.T.) ;
#1515=FACE_OUTER_BOUND('',#2117,.T.) ;
#1516=FACE_OUTER_BOUND('',#2118,.T.) ;
#1517=FACE_OUTER_BOUND('',#2119,.T.) ;
#1518=FACE_OUTER_BOUND('',#2120,.T.) ;
#1519=FACE_OUTER_BOUND('',#2121,.T.) ;
#1520=FACE_OUTER_BOUND('',#2122,.T.) ;
#1521=FACE_OUTER_BOUND('',#2123,.T.) ;
#1522=FACE_OUTER_BOUND('',#2125,.T.) ;
#1523=FACE_OUTER_BOUND('',#2126,.T.) ;
#1524=FACE_OUTER_BOUND('',#2127,.T.) ;
#1525=FACE_OUTER_BOUND('',#2128,.T.) ;
#1526=FACE_OUTER_BOUND('',#2129,.T.) ;
#1527=FACE_OUTER_BOUND('',#2130,.T.) ;
#1528=FACE_OUTER_BOUND('',#2131,.T.) ;
#1529=FACE_OUTER_BOUND('',#2132,.T.) ;
#1530=FACE_OUTER_BOUND('',#2133,.T.) ;
#1531=FACE_OUTER_BOUND('',#2134,.T.) ;
#1532=FACE_OUTER_BOUND('',#2135,.T.) ;
#1533=FACE_OUTER_BOUND('',#2136,.T.) ;
#1534=FACE_OUTER_BOUND('',#2137,.T.) ;
#1535=FACE_OUTER_BOUND('',#2138,.T.) ;
#1536=FACE_OUTER_BOUND('',#2139,.T.) ;
#1537=FACE_OUTER_BOUND('',#2140,.T.) ;
#1538=FACE_OUTER_BOUND('',#2141,.T.) ;
#1539=FACE_OUTER_BOUND('',#2142,.T.) ;
#1540=FACE_OUTER_BOUND('',#2143,.T.) ;
#1541=FACE_OUTER_BOUND('',#2144,.T.) ;
#1542=FACE_OUTER_BOUND('',#2145,.T.) ;
#1543=FACE_OUTER_BOUND('',#2146,.T.) ;
#1544=FACE_OUTER_BOUND('',#2147,.T.) ;
#1545=FACE_OUTER_BOUND('',#2148,.T.) ;
#1546=FACE_OUTER_BOUND('',#2149,.T.) ;
#1547=FACE_OUTER_BOUND('',#2150,.T.) ;
#1973=EDGE_LOOP('',(#7729,#7730,#7731,#7732)) ;
#1974=EDGE_LOOP('',(#7733,#7734,#7735,#7736)) ;
#1975=EDGE_LOOP('',(#7737,#7738,#7739,#7740)) ;
#1976=EDGE_LOOP('',(#7741,#7742,#7743,#7744)) ;
#1977=EDGE_LOOP('',(#7745,#7746,#7747,#7748)) ;
#1978=EDGE_LOOP('',(#7749,#7750,#7751,#7752)) ;
#1979=EDGE_LOOP('',(#7753,#7754,#7755,#7756)) ;
#1980=EDGE_LOOP('',(#7757,#7758,#7759,#7760)) ;
#1981=EDGE_LOOP('',(#7761,#7762,#7763,#7764)) ;
#1982=EDGE_LOOP('',(#7765,#7766,#7767,#7768)) ;
#1983=EDGE_LOOP('',(#7769,#7770,#7771,#7772)) ;
#1984=EDGE_LOOP('',(#7773,#7774,#7775,#7776)) ;
#1985=EDGE_LOOP('',(#7777,#7778,#7779,#7780)) ;
#1986=EDGE_LOOP('',(#7781,#7782,#7783,#7784)) ;
#1987=EDGE_LOOP('',(#7785,#7786,#7787,#7788)) ;
#1988=EDGE_LOOP('',(#7789,#7790,#7791,#7792)) ;
#1989=EDGE_LOOP('',(#7793,#7794,#7795,#7796)) ;
#1990=EDGE_LOOP('',(#7797,#7798,#7799,#7800)) ;
#1991=EDGE_LOOP('',(#7801,#7802,#7803,#7804)) ;
#1992=EDGE_LOOP('',(#7805,#7806,#7807,#7808)) ;
#1993=EDGE_LOOP('',(#7809,#7810,#7811,#7812)) ;
#1994=EDGE_LOOP('',(#7813,#7814,#7815,#7816)) ;
#1995=EDGE_LOOP('',(#7817,#7818,#7819,#7820)) ;
#1996=EDGE_LOOP('',(#7821,#7822,#7823,#7824)) ;
#1997=EDGE_LOOP('',(#7825,#7826,#7827,#7828)) ;
#1998=EDGE_LOOP('',(#7829,#7830,#7831,#7832)) ;
#1999=EDGE_LOOP('',(#7833,#7834,#7835,#7836)) ;
#2000=EDGE_LOOP('',(#7837,#7838,#7839,#7840)) ;
#2001=EDGE_LOOP('',(#7841,#7842,#7843,#7844,#7845)) ;
#2002=EDGE_LOOP('',(#7846,#7847,#7848,#7849,#7850,#7851,#7852,#7853,#7854,
#7855,#7856,#7857,#7858,#7859,#7860,#7861,#7862,#7863,#7864,#7865,#7866,
#7867,#7868,#7869,#7870,#7871,#7872,#7873,#7874,#7875,#7876,#7877)) ;
#2003=EDGE_LOOP('',(#7878,#7879,#7880,#7881,#7882)) ;
#2004=EDGE_LOOP('',(#7883,#7884,#7885,#7886)) ;
#2005=EDGE_LOOP('',(#7887,#7888,#7889,#7890,#7891,#7892,#7893,#7894,#7895,
#7896,#7897,#7898,#7899,#7900,#7901,#7902,#7903,#7904,#7905,#7906,#7907,
#7908,#7909,#7910,#7911,#7912,#7913,#7914,#7915,#7916,#7917,#7918)) ;
#2006=EDGE_LOOP('',(#7919,#7920,#7921,#7922,#7923,#7924)) ;
#2007=EDGE_LOOP('',(#7925,#7926,#7927,#7928)) ;
#2008=EDGE_LOOP('',(#7929)) ;
#2009=EDGE_LOOP('',(#7930)) ;
#2010=EDGE_LOOP('',(#7931,#7932,#7933,#7934,#7935,#7936)) ;
#2011=EDGE_LOOP('',(#7937)) ;
#2012=EDGE_LOOP('',(#7938,#7939,#7940)) ;
#2013=EDGE_LOOP('',(#7941,#7942,#7943,#7944)) ;
#2014=EDGE_LOOP('',(#7945,#7946,#7947,#7948)) ;
#2015=EDGE_LOOP('',(#7949,#7950,#7951,#7952,#7953,#7954,#7955,#7956,#7957,
#7958,#7959,#7960,#7961,#7962,#7963,#7964,#7965,#7966,#7967,#7968,#7969,
#7970,#7971,#7972,#7973,#7974,#7975,#7976,#7977,#7978,#7979,#7980,#7981,
#7982,#7983,#7984,#7985,#7986,#7987,#7988,#7989,#7990,#7991,#7992,#7993,
#7994,#7995,#7996,#7997,#7998,#7999,#8000,#8001,#8002,#8003,#8004,#8005,
#8006,#8007,#8008,#8009,#8010,#8011,#8012,#8013,#8014,#8015,#8016,#8017,
#8018,#8019,#8020,#8021,#8022,#8023,#8024,#8025,#8026,#8027,#8028,#8029,
#8030,#8031,#8032,#8033,#8034,#8035,#8036,#8037,#8038,#8039,#8040,#8041,
#8042,#8043,#8044,#8045,#8046,#8047,#8048,#8049,#8050,#8051,#8052,#8053,
#8054,#8055,#8056,#8057,#8058,#8059,#8060,#8061,#8062,#8063,#8064,#8065,
#8066,#8067,#8068,#8069,#8070,#8071,#8072,#8073,#8074,#8075,#8076,#8077,
#8078,#8079,#8080,#8081,#8082,#8083,#8084,#8085,#8086,#8087,#8088,#8089,
#8090,#8091,#8092,#8093,#8094,#8095,#8096)) ;
#2016=EDGE_LOOP('',(#8097,#8098,#8099,#8100)) ;
#2017=EDGE_LOOP('',(#8101,#8102,#8103,#8104)) ;
#2018=EDGE_LOOP('',(#8105,#8106,#8107)) ;
#2019=EDGE_LOOP('',(#8108,#8109,#8110,#8111,#8112,#8113,#8114,#8115,#8116,
#8117,#8118,#8119,#8120,#8121,#8122,#8123,#8124,#8125,#8126,#8127,#8128,
#8129,#8130,#8131,#8132,#8133,#8134,#8135,#8136,#8137,#8138,#8139,#8140,
#8141,#8142,#8143,#8144,#8145,#8146,#8147,#8148,#8149,#8150,#8151,#8152,
#8153,#8154,#8155,#8156,#8157,#8158,#8159,#8160,#8161,#8162,#8163,#8164,
#8165,#8166,#8167,#8168,#8169,#8170,#8171,#8172,#8173,#8174,#8175,#8176,
#8177,#8178,#8179,#8180,#8181,#8182,#8183,#8184,#8185,#8186,#8187,#8188,
#8189,#8190,#8191,#8192,#8193,#8194,#8195,#8196,#8197,#8198,#8199,#8200,
#8201,#8202,#8203,#8204,#8205,#8206,#8207,#8208,#8209,#8210,#8211,#8212,
#8213,#8214,#8215,#8216,#8217,#8218)) ;
#2020=EDGE_LOOP('',(#8219,#8220,#8221)) ;
#2021=EDGE_LOOP('',(#8222,#8223,#8224,#8225)) ;
#2022=EDGE_LOOP('',(#8226,#8227,#8228,#8229)) ;
#2023=EDGE_LOOP('',(#8230,#8231,#8232,#8233)) ;
#2024=EDGE_LOOP('',(#8234,#8235,#8236,#8237)) ;
#2025=EDGE_LOOP('',(#8238,#8239,#8240)) ;
#2026=EDGE_LOOP('',(#8241,#8242,#8243)) ;
#2027=EDGE_LOOP('',(#8244,#8245,#8246,#8247)) ;
#2028=EDGE_LOOP('',(#8248,#8249,#8250,#8251)) ;
#2029=EDGE_LOOP('',(#8252,#8253,#8254,#8255)) ;
#2030=EDGE_LOOP('',(#8256,#8257,#8258,#8259)) ;
#2031=EDGE_LOOP('',(#8260,#8261,#8262)) ;
#2032=EDGE_LOOP('',(#8263,#8264,#8265)) ;
#2033=EDGE_LOOP('',(#8266,#8267,#8268,#8269)) ;
#2034=EDGE_LOOP('',(#8270,#8271,#8272,#8273)) ;
#2035=EDGE_LOOP('',(#8274,#8275,#8276,#8277)) ;
#2036=EDGE_LOOP('',(#8278,#8279,#8280,#8281)) ;
#2037=EDGE_LOOP('',(#8282,#8283,#8284)) ;
#2038=EDGE_LOOP('',(#8285,#8286,#8287)) ;
#2039=EDGE_LOOP('',(#8288,#8289,#8290,#8291)) ;
#2040=EDGE_LOOP('',(#8292,#8293,#8294,#8295)) ;
#2041=EDGE_LOOP('',(#8296,#8297,#8298,#8299)) ;
#2042=EDGE_LOOP('',(#8300,#8301,#8302,#8303)) ;
#2043=EDGE_LOOP('',(#8304,#8305,#8306)) ;
#2044=EDGE_LOOP('',(#8307,#8308,#8309)) ;
#2045=EDGE_LOOP('',(#8310,#8311,#8312,#8313)) ;
#2046=EDGE_LOOP('',(#8314,#8315,#8316,#8317)) ;
#2047=EDGE_LOOP('',(#8318,#8319,#8320,#8321)) ;
#2048=EDGE_LOOP('',(#8322,#8323,#8324,#8325)) ;
#2049=EDGE_LOOP('',(#8326,#8327,#8328)) ;
#2050=EDGE_LOOP('',(#8329,#8330,#8331)) ;
#2051=EDGE_LOOP('',(#8332,#8333,#8334,#8335)) ;
#2052=EDGE_LOOP('',(#8336,#8337,#8338,#8339)) ;
#2053=EDGE_LOOP('',(#8340,#8341,#8342,#8343)) ;
#2054=EDGE_LOOP('',(#8344,#8345,#8346,#8347)) ;
#2055=EDGE_LOOP('',(#8348,#8349,#8350)) ;
#2056=EDGE_LOOP('',(#8351,#8352,#8353)) ;
#2057=EDGE_LOOP('',(#8354,#8355,#8356,#8357)) ;
#2058=EDGE_LOOP('',(#8358,#8359,#8360,#8361)) ;
#2059=EDGE_LOOP('',(#8362,#8363,#8364,#8365)) ;
#2060=EDGE_LOOP('',(#8366,#8367,#8368,#8369)) ;
#2061=EDGE_LOOP('',(#8370,#8371,#8372)) ;
#2062=EDGE_LOOP('',(#8373,#8374,#8375)) ;
#2063=EDGE_LOOP('',(#8376,#8377,#8378,#8379)) ;
#2064=EDGE_LOOP('',(#8380,#8381,#8382,#8383)) ;
#2065=EDGE_LOOP('',(#8384,#8385,#8386,#8387)) ;
#2066=EDGE_LOOP('',(#8388,#8389,#8390,#8391)) ;
#2067=EDGE_LOOP('',(#8392,#8393,#8394,#8395)) ;
#2068=EDGE_LOOP('',(#8396,#8397,#8398)) ;
#2069=EDGE_LOOP('',(#8399,#8400,#8401,#8402)) ;
#2070=EDGE_LOOP('',(#8403,#8404,#8405,#8406)) ;
#2071=EDGE_LOOP('',(#8407,#8408,#8409,#8410)) ;
#2072=EDGE_LOOP('',(#8411,#8412,#8413,#8414)) ;
#2073=EDGE_LOOP('',(#8415,#8416,#8417)) ;
#2074=EDGE_LOOP('',(#8418,#8419,#8420)) ;
#2075=EDGE_LOOP('',(#8421,#8422,#8423,#8424)) ;
#2076=EDGE_LOOP('',(#8425,#8426,#8427,#8428)) ;
#2077=EDGE_LOOP('',(#8429,#8430,#8431,#8432)) ;
#2078=EDGE_LOOP('',(#8433,#8434,#8435,#8436)) ;
#2079=EDGE_LOOP('',(#8437,#8438,#8439)) ;
#2080=EDGE_LOOP('',(#8440,#8441,#8442)) ;
#2081=EDGE_LOOP('',(#8443,#8444,#8445,#8446)) ;
#2082=EDGE_LOOP('',(#8447,#8448,#8449,#8450)) ;
#2083=EDGE_LOOP('',(#8451,#8452,#8453,#8454)) ;
#2084=EDGE_LOOP('',(#8455,#8456,#8457,#8458)) ;
#2085=EDGE_LOOP('',(#8459,#8460,#8461)) ;
#2086=EDGE_LOOP('',(#8462,#8463,#8464)) ;
#2087=EDGE_LOOP('',(#8465,#8466,#8467,#8468)) ;
#2088=EDGE_LOOP('',(#8469,#8470,#8471,#8472)) ;
#2089=EDGE_LOOP('',(#8473,#8474,#8475,#8476)) ;
#2090=EDGE_LOOP('',(#8477,#8478,#8479,#8480)) ;
#2091=EDGE_LOOP('',(#8481,#8482,#8483)) ;
#2092=EDGE_LOOP('',(#8484,#8485,#8486)) ;
#2093=EDGE_LOOP('',(#8487,#8488,#8489,#8490)) ;
#2094=EDGE_LOOP('',(#8491,#8492,#8493,#8494)) ;
#2095=EDGE_LOOP('',(#8495,#8496,#8497,#8498)) ;
#2096=EDGE_LOOP('',(#8499,#8500,#8501,#8502)) ;
#2097=EDGE_LOOP('',(#8503,#8504,#8505)) ;
#2098=EDGE_LOOP('',(#8506,#8507,#8508)) ;
#2099=EDGE_LOOP('',(#8509,#8510,#8511,#8512)) ;
#2100=EDGE_LOOP('',(#8513,#8514,#8515,#8516)) ;
#2101=EDGE_LOOP('',(#8517,#8518,#8519,#8520)) ;
#2102=EDGE_LOOP('',(#8521,#8522,#8523,#8524)) ;
#2103=EDGE_LOOP('',(#8525,#8526,#8527)) ;
#2104=EDGE_LOOP('',(#8528,#8529,#8530)) ;
#2105=EDGE_LOOP('',(#8531,#8532,#8533,#8534)) ;
#2106=EDGE_LOOP('',(#8535,#8536,#8537,#8538)) ;
#2107=EDGE_LOOP('',(#8539,#8540,#8541,#8542)) ;
#2108=EDGE_LOOP('',(#8543,#8544,#8545,#8546)) ;
#2109=EDGE_LOOP('',(#8547,#8548,#8549)) ;
#2110=EDGE_LOOP('',(#8550,#8551,#8552)) ;
#2111=EDGE_LOOP('',(#8553,#8554,#8555,#8556)) ;
#2112=EDGE_LOOP('',(#8557,#8558,#8559,#8560)) ;
#2113=EDGE_LOOP('',(#8561,#8562,#8563,#8564)) ;
#2114=EDGE_LOOP('',(#8565,#8566,#8567,#8568)) ;
#2115=EDGE_LOOP('',(#8569,#8570,#8571)) ;
#2116=EDGE_LOOP('',(#8572,#8573,#8574)) ;
#2117=EDGE_LOOP('',(#8575,#8576,#8577,#8578)) ;
#2118=EDGE_LOOP('',(#8579,#8580,#8581,#8582)) ;
#2119=EDGE_LOOP('',(#8583,#8584,#8585,#8586)) ;
#2120=EDGE_LOOP('',(#8587,#8588,#8589,#8590)) ;
#2121=EDGE_LOOP('',(#8591,#8592,#8593)) ;
#2122=EDGE_LOOP('',(#8594,#8595,#8596,#8597)) ;
#2123=EDGE_LOOP('',(#8598)) ;
#2124=EDGE_LOOP('',(#8599)) ;
#2125=EDGE_LOOP('',(#8600,#8601,#8602,#8603,#8604,#8605,#8606,#8607,#8608,
#8609,#8610,#8611,#8612,#8613,#8614,#8615,#8616,#8617,#8618,#8619,#8620)) ;
#2126=EDGE_LOOP('',(#8621,#8622,#8623,#8624)) ;
#2127=EDGE_LOOP('',(#8625,#8626,#8627,#8628)) ;
#2128=EDGE_LOOP('',(#8629,#8630,#8631,#8632)) ;
#2129=EDGE_LOOP('',(#8633,#8634,#8635,#8636)) ;
#2130=EDGE_LOOP('',(#8637,#8638,#8639,#8640)) ;
#2131=EDGE_LOOP('',(#8641,#8642,#8643,#8644)) ;
#2132=EDGE_LOOP('',(#8645,#8646,#8647,#8648,#8649,#8650,#8651,#8652)) ;
#2133=EDGE_LOOP('',(#8653,#8654,#8655,#8656,#8657,#8658,#8659,#8660)) ;
#2134=EDGE_LOOP('',(#8661,#8662,#8663,#8664,#8665,#8666,#8667,#8668)) ;
#2135=EDGE_LOOP('',(#8669,#8670)) ;
#2136=EDGE_LOOP('',(#8671,#8672)) ;
#2137=EDGE_LOOP('',(#8673,#8674)) ;
#2138=EDGE_LOOP('',(#8675,#8676)) ;
#2139=EDGE_LOOP('',(#8677,#8678)) ;
#2140=EDGE_LOOP('',(#8679,#8680)) ;
#2141=EDGE_LOOP('',(#8681,#8682)) ;
#2142=EDGE_LOOP('',(#8683,#8684)) ;
#2143=EDGE_LOOP('',(#8685,#8686)) ;
#2144=EDGE_LOOP('',(#8687,#8688)) ;
#2145=EDGE_LOOP('',(#8689,#8690)) ;
#2146=EDGE_LOOP('',(#8691,#8692)) ;
#2147=EDGE_LOOP('',(#8693,#8694,#8695,#8696,#8697,#8698,#8699,#8700)) ;
#2148=EDGE_LOOP('',(#8701,#8702,#8703,#8704,#8705,#8706,#8707,#8708)) ;
#2149=EDGE_LOOP('',(#8709,#8710,#8711,#8712,#8713,#8714,#8715,#8716)) ;
#2150=EDGE_LOOP('',(#8717,#8718,#8719,#8720,#8721,#8722,#8723,#8724)) ;
#2671=LINE('',#15302,#3442) ;
#2672=LINE('',#15326,#3443) ;
#2673=LINE('',#15374,#3444) ;
#2674=LINE('',#15422,#3445) ;
#2675=LINE('',#15476,#3446) ;
#2676=LINE('',#15524,#3447) ;
#2677=LINE('',#15572,#3448) ;
#2678=LINE('',#15626,#3449) ;
#2679=LINE('',#15674,#3450) ;
#2680=LINE('',#15722,#3451) ;
#2681=LINE('',#15776,#3452) ;
#2682=LINE('',#15824,#3453) ;
#2683=LINE('',#15872,#3454) ;
#2684=LINE('',#15926,#3455) ;
#2685=LINE('',#15974,#3456) ;
#2686=LINE('',#15990,#3457) ;
#2687=LINE('',#16014,#3458) ;
#2688=LINE('',#16039,#3459) ;
#2689=LINE('',#16064,#3460) ;
#2690=LINE('',#16088,#3461) ;
#2691=LINE('',#16113,#3462) ;
#2692=LINE('',#16138,#3463) ;
#2693=LINE('',#16162,#3464) ;
#2694=LINE('',#16187,#3465) ;
#2695=LINE('',#16212,#3466) ;
#2696=LINE('',#16236,#3467) ;
#2697=LINE('',#16261,#3468) ;
#2698=LINE('',#16286,#3469) ;
#2699=LINE('',#17420,#3470) ;
#2700=LINE('',#17428,#3471) ;
#2701=LINE('',#17429,#3472) ;
#2702=LINE('',#17432,#3473) ;
#2703=LINE('',#17434,#3474) ;
#2704=LINE('',#17440,#3475) ;
#2705=LINE('',#17448,#3476) ;
#2706=LINE('',#17452,#3477) ;
#2707=LINE('',#17456,#3478) ;
#2708=LINE('',#17460,#3479) ;
#2709=LINE('',#17464,#3480) ;
#2710=LINE('',#17468,#3481) ;
#2711=LINE('',#17472,#3482) ;
#2712=LINE('',#17476,#3483) ;
#2713=LINE('',#17480,#3484) ;
#2714=LINE('',#17484,#3485) ;
#2715=LINE('',#17488,#3486) ;
#2716=LINE('',#17492,#3487) ;
#2717=LINE('',#17496,#3488) ;
#2718=LINE('',#17500,#3489) ;
#2719=LINE('',#17504,#3490) ;
#2720=LINE('',#17508,#3491) ;
#2721=LINE('',#17512,#3492) ;
#2722=LINE('',#17516,#3493) ;
#2723=LINE('',#17520,#3494) ;
#2724=LINE('',#17524,#3495) ;
#2725=LINE('',#17528,#3496) ;
#2726=LINE('',#17532,#3497) ;
#2727=LINE('',#17536,#3498) ;
#2728=LINE('',#17540,#3499) ;
#2729=LINE('',#17544,#3500) ;
#2730=LINE('',#17548,#3501) ;
#2731=LINE('',#17552,#3502) ;
#2732=LINE('',#17556,#3503) ;
#2733=LINE('',#17560,#3504) ;
#2734=LINE('',#17564,#3505) ;
#2735=LINE('',#17568,#3506) ;
#2736=LINE('',#17572,#3507) ;
#2737=LINE('',#17576,#3508) ;
#2738=LINE('',#17580,#3509) ;
#2739=LINE('',#17584,#3510) ;
#2740=LINE('',#17588,#3511) ;
#2741=LINE('',#17592,#3512) ;
#2742=LINE('',#17596,#3513) ;
#2743=LINE('',#17601,#3514) ;
#2744=LINE('',#17605,#3515) ;
#2745=LINE('',#17609,#3516) ;
#2746=LINE('',#17613,#3517) ;
#2747=LINE('',#17617,#3518) ;
#2748=LINE('',#17621,#3519) ;
#2749=LINE('',#17625,#3520) ;
#2750=LINE('',#17629,#3521) ;
#2751=LINE('',#17633,#3522) ;
#2752=LINE('',#17637,#3523) ;
#2753=LINE('',#17641,#3524) ;
#2754=LINE('',#17645,#3525) ;
#2755=LINE('',#17649,#3526) ;
#2756=LINE('',#17653,#3527) ;
#2757=LINE('',#17657,#3528) ;
#2758=LINE('',#17661,#3529) ;
#2759=LINE('',#17665,#3530) ;
#2760=LINE('',#17669,#3531) ;
#2761=LINE('',#17673,#3532) ;
#2762=LINE('',#17677,#3533) ;
#2763=LINE('',#17681,#3534) ;
#2764=LINE('',#17685,#3535) ;
#2765=LINE('',#17689,#3536) ;
#2766=LINE('',#17693,#3537) ;
#2767=LINE('',#17697,#3538) ;
#2768=LINE('',#17701,#3539) ;
#2769=LINE('',#17705,#3540) ;
#2770=LINE('',#17709,#3541) ;
#2771=LINE('',#17713,#3542) ;
#2772=LINE('',#17717,#3543) ;
#2773=LINE('',#17721,#3544) ;
#2774=LINE('',#17725,#3545) ;
#2775=LINE('',#17729,#3546) ;
#2776=LINE('',#17733,#3547) ;
#2777=LINE('',#17735,#3548) ;
#2778=LINE('',#17743,#3549) ;
#2779=LINE('',#17749,#3550) ;
#2780=LINE('',#17989,#3551) ;
#2781=LINE('',#17990,#3552) ;
#2782=LINE('',#17992,#3553) ;
#2783=LINE('',#17996,#3554) ;
#2784=LINE('',#17997,#3555) ;
#2785=LINE('',#17999,#3556) ;
#2786=LINE('',#18003,#3557) ;
#2787=LINE('',#18004,#3558) ;
#2788=LINE('',#18006,#3559) ;
#2789=LINE('',#18010,#3560) ;
#2790=LINE('',#18011,#3561) ;
#2791=LINE('',#18013,#3562) ;
#2792=LINE('',#18017,#3563) ;
#2793=LINE('',#18018,#3564) ;
#2794=LINE('',#18020,#3565) ;
#2795=LINE('',#18024,#3566) ;
#2796=LINE('',#18025,#3567) ;
#2797=LINE('',#18027,#3568) ;
#2798=LINE('',#18031,#3569) ;
#2799=LINE('',#18032,#3570) ;
#2800=LINE('',#18034,#3571) ;
#2801=LINE('',#18038,#3572) ;
#2802=LINE('',#18039,#3573) ;
#2803=LINE('',#18041,#3574) ;
#2804=LINE('',#18045,#3575) ;
#2805=LINE('',#18046,#3576) ;
#2806=LINE('',#18048,#3577) ;
#2807=LINE('',#18052,#3578) ;
#2808=LINE('',#18053,#3579) ;
#2809=LINE('',#18055,#3580) ;
#2810=LINE('',#18059,#3581) ;
#2811=LINE('',#18060,#3582) ;
#2812=LINE('',#18062,#3583) ;
#2813=LINE('',#18066,#3584) ;
#2814=LINE('',#18067,#3585) ;
#2815=LINE('',#18069,#3586) ;
#2816=LINE('',#18073,#3587) ;
#2817=LINE('',#18074,#3588) ;
#2818=LINE('',#18076,#3589) ;
#2819=LINE('',#18080,#3590) ;
#2820=LINE('',#18081,#3591) ;
#2821=LINE('',#18083,#3592) ;
#2822=LINE('',#18087,#3593) ;
#2823=LINE('',#18088,#3594) ;
#2824=LINE('',#18090,#3595) ;
#2825=LINE('',#18094,#3596) ;
#2826=LINE('',#18095,#3597) ;
#2827=LINE('',#18097,#3598) ;
#2828=LINE('',#18101,#3599) ;
#2829=LINE('',#18102,#3600) ;
#2830=LINE('',#18104,#3601) ;
#2831=LINE('',#18108,#3602) ;
#2832=LINE('',#18109,#3603) ;
#2833=LINE('',#18111,#3604) ;
#2834=LINE('',#18115,#3605) ;
#2835=LINE('',#18116,#3606) ;
#2836=LINE('',#18118,#3607) ;
#2837=LINE('',#18122,#3608) ;
#2838=LINE('',#18123,#3609) ;
#2839=LINE('',#18125,#3610) ;
#2840=LINE('',#18129,#3611) ;
#2841=LINE('',#18130,#3612) ;
#2842=LINE('',#18132,#3613) ;
#2843=LINE('',#18136,#3614) ;
#2844=LINE('',#18137,#3615) ;
#2845=LINE('',#18139,#3616) ;
#2846=LINE('',#18143,#3617) ;
#2847=LINE('',#18144,#3618) ;
#2848=LINE('',#18146,#3619) ;
#2849=LINE('',#18150,#3620) ;
#2850=LINE('',#18151,#3621) ;
#2851=LINE('',#18153,#3622) ;
#2852=LINE('',#18157,#3623) ;
#2853=LINE('',#18158,#3624) ;
#2854=LINE('',#18160,#3625) ;
#2855=LINE('',#18164,#3626) ;
#2856=LINE('',#18165,#3627) ;
#2857=LINE('',#18167,#3628) ;
#2858=LINE('',#18171,#3629) ;
#2859=LINE('',#18172,#3630) ;
#2860=LINE('',#18174,#3631) ;
#2861=LINE('',#18178,#3632) ;
#2862=LINE('',#18179,#3633) ;
#2863=LINE('',#18181,#3634) ;
#2864=LINE('',#18185,#3635) ;
#2865=LINE('',#18186,#3636) ;
#2866=LINE('',#18188,#3637) ;
#2867=LINE('',#18192,#3638) ;
#2868=LINE('',#18193,#3639) ;
#2869=LINE('',#18195,#3640) ;
#2870=LINE('',#18199,#3641) ;
#2871=LINE('',#18200,#3642) ;
#2872=LINE('',#18202,#3643) ;
#2873=LINE('',#18206,#3644) ;
#2874=LINE('',#18207,#3645) ;
#2875=LINE('',#18209,#3646) ;
#2876=LINE('',#18213,#3647) ;
#2877=LINE('',#18214,#3648) ;
#2878=LINE('',#18216,#3649) ;
#2879=LINE('',#18220,#3650) ;
#2880=LINE('',#18221,#3651) ;
#2881=LINE('',#18223,#3652) ;
#2882=LINE('',#18232,#3653) ;
#2883=LINE('',#18294,#3654) ;
#2884=LINE('',#18296,#3655) ;
#2885=LINE('',#18300,#3656) ;
#2886=LINE('',#18302,#3657) ;
#2887=LINE('',#18306,#3658) ;
#2888=LINE('',#18309,#3659) ;
#2889=LINE('',#18312,#3660) ;
#2890=LINE('',#18314,#3661) ;
#2891=LINE('',#18318,#3662) ;
#2892=LINE('',#18321,#3663) ;
#2893=LINE('',#18324,#3664) ;
#2894=LINE('',#18327,#3665) ;
#2895=LINE('',#18329,#3666) ;
#2896=LINE('',#18331,#3667) ;
#2897=LINE('',#18333,#3668) ;
#2898=LINE('',#18334,#3669) ;
#2899=LINE('',#18336,#3670) ;
#2900=LINE('',#18338,#3671) ;
#2901=LINE('',#18339,#3672) ;
#2902=LINE('',#18341,#3673) ;
#2903=LINE('',#18343,#3674) ;
#2904=LINE('',#18344,#3675) ;
#2905=LINE('',#18348,#3676) ;
#2906=LINE('',#18351,#3677) ;
#2907=LINE('',#18353,#3678) ;
#2908=LINE('',#18356,#3679) ;
#2909=LINE('',#18366,#3680) ;
#2910=LINE('',#18369,#3681) ;
#2911=LINE('',#18373,#3682) ;
#2912=LINE('',#18375,#3683) ;
#2913=LINE('',#18377,#3684) ;
#3442=VECTOR('',#12203,0.999999999999996) ;
#3443=VECTOR('',#12208,0.999999999999996) ;
#3444=VECTOR('',#12211,0.999999999999996) ;
#3445=VECTOR('',#12214,0.999999999999996) ;
#3446=VECTOR('',#12217,0.999999999999996) ;
#3447=VECTOR('',#12220,0.999999999999996) ;
#3448=VECTOR('',#12223,0.999999999999996) ;
#3449=VECTOR('',#12226,0.999999999999996) ;
#3450=VECTOR('',#12229,0.999999999999996) ;
#3451=VECTOR('',#12232,0.999999999999996) ;
#3452=VECTOR('',#12235,0.999999999999996) ;
#3453=VECTOR('',#12238,0.999999999999996) ;
#3454=VECTOR('',#12241,0.999999999999996) ;
#3455=VECTOR('',#12244,0.999999999999996) ;
#3456=VECTOR('',#12247,0.739000000000001) ;
#3457=VECTOR('',#12252,0.739000000000001) ;
#3458=VECTOR('',#12255,0.739000000000001) ;
#3459=VECTOR('',#12258,0.739000000000001) ;
#3460=VECTOR('',#12261,0.739000000000001) ;
#3461=VECTOR('',#12264,0.739000000000001) ;
#3462=VECTOR('',#12267,0.739000000000001) ;
#3463=VECTOR('',#12270,0.739000000000001) ;
#3464=VECTOR('',#12273,0.739000000000001) ;
#3465=VECTOR('',#12276,0.739000000000001) ;
#3466=VECTOR('',#12279,0.739000000000001) ;
#3467=VECTOR('',#12282,0.739000000000001) ;
#3468=VECTOR('',#12285,0.739000000000001) ;
#3469=VECTOR('',#12288,0.739000000000001) ;
#3470=VECTOR('',#12321,0.79175) ;
#3471=VECTOR('',#12330,10.) ;
#3472=VECTOR('',#12331,10.) ;
#3473=VECTOR('',#12334,10.) ;
#3474=VECTOR('',#12335,10.) ;
#3475=VECTOR('',#12338,10.) ;
#3476=VECTOR('',#12343,10.) ;
#3477=VECTOR('',#12346,10.) ;
#3478=VECTOR('',#12349,10.) ;
#3479=VECTOR('',#12352,10.) ;
#3480=VECTOR('',#12355,10.) ;
#3481=VECTOR('',#12358,10.) ;
#3482=VECTOR('',#12361,10.) ;
#3483=VECTOR('',#12364,10.) ;
#3484=VECTOR('',#12367,10.) ;
#3485=VECTOR('',#12370,10.) ;
#3486=VECTOR('',#12373,10.) ;
#3487=VECTOR('',#12376,10.) ;
#3488=VECTOR('',#12379,10.) ;
#3489=VECTOR('',#12382,10.) ;
#3490=VECTOR('',#12385,10.) ;
#3491=VECTOR('',#12388,10.) ;
#3492=VECTOR('',#12391,10.) ;
#3493=VECTOR('',#12394,10.) ;
#3494=VECTOR('',#12397,10.) ;
#3495=VECTOR('',#12400,10.) ;
#3496=VECTOR('',#12403,10.) ;
#3497=VECTOR('',#12406,10.) ;
#3498=VECTOR('',#12409,10.) ;
#3499=VECTOR('',#12412,10.) ;
#3500=VECTOR('',#12415,10.) ;
#3501=VECTOR('',#12418,10.) ;
#3502=VECTOR('',#12421,10.) ;
#3503=VECTOR('',#12424,10.) ;
#3504=VECTOR('',#12427,10.) ;
#3505=VECTOR('',#12430,10.) ;
#3506=VECTOR('',#12433,10.) ;
#3507=VECTOR('',#12436,10.) ;
#3508=VECTOR('',#12439,10.) ;
#3509=VECTOR('',#12442,10.) ;
#3510=VECTOR('',#12445,10.) ;
#3511=VECTOR('',#12448,10.) ;
#3512=VECTOR('',#12451,10.) ;
#3513=VECTOR('',#12454,1.9) ;
#3514=VECTOR('',#12459,10.) ;
#3515=VECTOR('',#12462,10.) ;
#3516=VECTOR('',#12465,10.) ;
#3517=VECTOR('',#12468,10.) ;
#3518=VECTOR('',#12471,10.) ;
#3519=VECTOR('',#12474,10.) ;
#3520=VECTOR('',#12477,10.) ;
#3521=VECTOR('',#12480,10.) ;
#3522=VECTOR('',#12483,10.) ;
#3523=VECTOR('',#12486,10.) ;
#3524=VECTOR('',#12489,10.) ;
#3525=VECTOR('',#12492,10.) ;
#3526=VECTOR('',#12495,10.) ;
#3527=VECTOR('',#12498,10.) ;
#3528=VECTOR('',#12501,10.) ;
#3529=VECTOR('',#12504,10.) ;
#3530=VECTOR('',#12507,10.) ;
#3531=VECTOR('',#12510,10.) ;
#3532=VECTOR('',#12513,10.) ;
#3533=VECTOR('',#12516,10.) ;
#3534=VECTOR('',#12519,10.) ;
#3535=VECTOR('',#12522,10.) ;
#3536=VECTOR('',#12525,10.) ;
#3537=VECTOR('',#12528,10.) ;
#3538=VECTOR('',#12531,10.) ;
#3539=VECTOR('',#12534,10.) ;
#3540=VECTOR('',#12537,10.) ;
#3541=VECTOR('',#12540,10.) ;
#3542=VECTOR('',#12543,10.) ;
#3543=VECTOR('',#12546,10.) ;
#3544=VECTOR('',#12549,10.) ;
#3545=VECTOR('',#12552,10.) ;
#3546=VECTOR('',#12555,10.) ;
#3547=VECTOR('',#12560,10.) ;
#3548=VECTOR('',#12561,10.) ;
#3549=VECTOR('',#12564,10.) ;
#3550=VECTOR('',#12571,1.75) ;
#3551=VECTOR('',#12574,10.) ;
#3552=VECTOR('',#12575,10.) ;
#3553=VECTOR('',#12578,10.) ;
#3554=VECTOR('',#12583,10.) ;
#3555=VECTOR('',#12584,10.) ;
#3556=VECTOR('',#12587,10.) ;
#3557=VECTOR('',#12592,10.) ;
#3558=VECTOR('',#12593,10.) ;
#3559=VECTOR('',#12596,10.) ;
#3560=VECTOR('',#12601,10.) ;
#3561=VECTOR('',#12602,10.) ;
#3562=VECTOR('',#12605,10.) ;
#3563=VECTOR('',#12610,10.) ;
#3564=VECTOR('',#12611,10.) ;
#3565=VECTOR('',#12614,10.) ;
#3566=VECTOR('',#12619,10.) ;
#3567=VECTOR('',#12620,10.) ;
#3568=VECTOR('',#12623,10.) ;
#3569=VECTOR('',#12628,10.) ;
#3570=VECTOR('',#12629,10.) ;
#3571=VECTOR('',#12632,10.) ;
#3572=VECTOR('',#12637,10.) ;
#3573=VECTOR('',#12638,10.) ;
#3574=VECTOR('',#12641,10.) ;
#3575=VECTOR('',#12646,10.) ;
#3576=VECTOR('',#12647,10.) ;
#3577=VECTOR('',#12650,10.) ;
#3578=VECTOR('',#12655,10.) ;
#3579=VECTOR('',#12656,10.) ;
#3580=VECTOR('',#12659,10.) ;
#3581=VECTOR('',#12664,10.) ;
#3582=VECTOR('',#12665,10.) ;
#3583=VECTOR('',#12668,10.) ;
#3584=VECTOR('',#12673,10.) ;
#3585=VECTOR('',#12674,10.) ;
#3586=VECTOR('',#12677,10.) ;
#3587=VECTOR('',#12682,10.) ;
#3588=VECTOR('',#12683,10.) ;
#3589=VECTOR('',#12686,10.) ;
#3590=VECTOR('',#12691,10.) ;
#3591=VECTOR('',#12692,10.) ;
#3592=VECTOR('',#12695,10.) ;
#3593=VECTOR('',#12700,10.) ;
#3594=VECTOR('',#12701,10.) ;
#3595=VECTOR('',#12704,10.) ;
#3596=VECTOR('',#12709,10.) ;
#3597=VECTOR('',#12710,10.) ;
#3598=VECTOR('',#12713,10.) ;
#3599=VECTOR('',#12718,10.) ;
#3600=VECTOR('',#12719,10.) ;
#3601=VECTOR('',#12722,10.) ;
#3602=VECTOR('',#12727,10.) ;
#3603=VECTOR('',#12728,10.) ;
#3604=VECTOR('',#12731,10.) ;
#3605=VECTOR('',#12736,10.) ;
#3606=VECTOR('',#12737,10.) ;
#3607=VECTOR('',#12740,10.) ;
#3608=VECTOR('',#12745,10.) ;
#3609=VECTOR('',#12746,10.) ;
#3610=VECTOR('',#12749,10.) ;
#3611=VECTOR('',#12754,10.) ;
#3612=VECTOR('',#12755,10.) ;
#3613=VECTOR('',#12758,10.) ;
#3614=VECTOR('',#12763,10.) ;
#3615=VECTOR('',#12764,10.) ;
#3616=VECTOR('',#12767,10.) ;
#3617=VECTOR('',#12772,10.) ;
#3618=VECTOR('',#12773,10.) ;
#3619=VECTOR('',#12776,10.) ;
#3620=VECTOR('',#12781,10.) ;
#3621=VECTOR('',#12782,10.) ;
#3622=VECTOR('',#12785,10.) ;
#3623=VECTOR('',#12790,10.) ;
#3624=VECTOR('',#12791,10.) ;
#3625=VECTOR('',#12794,10.) ;
#3626=VECTOR('',#12799,10.) ;
#3627=VECTOR('',#12800,10.) ;
#3628=VECTOR('',#12803,10.) ;
#3629=VECTOR('',#12808,10.) ;
#3630=VECTOR('',#12809,10.) ;
#3631=VECTOR('',#12812,10.) ;
#3632=VECTOR('',#12817,10.) ;
#3633=VECTOR('',#12818,10.) ;
#3634=VECTOR('',#12821,10.) ;
#3635=VECTOR('',#12826,10.) ;
#3636=VECTOR('',#12827,10.) ;
#3637=VECTOR('',#12830,10.) ;
#3638=VECTOR('',#12835,10.) ;
#3639=VECTOR('',#12836,10.) ;
#3640=VECTOR('',#12839,10.) ;
#3641=VECTOR('',#12844,10.) ;
#3642=VECTOR('',#12845,10.) ;
#3643=VECTOR('',#12848,10.) ;
#3644=VECTOR('',#12853,10.) ;
#3645=VECTOR('',#12854,10.) ;
#3646=VECTOR('',#12857,10.) ;
#3647=VECTOR('',#12862,10.) ;
#3648=VECTOR('',#12863,10.) ;
#3649=VECTOR('',#12866,10.) ;
#3650=VECTOR('',#12871,10.) ;
#3651=VECTOR('',#12872,10.) ;
#3652=VECTOR('',#12875,10.) ;
#3653=VECTOR('',#12888,0.916025403784442) ;
#3654=VECTOR('',#12903,10.) ;
#3655=VECTOR('',#12904,10.) ;
#3656=VECTOR('',#12909,10.) ;
#3657=VECTOR('',#12910,10.) ;
#3658=VECTOR('',#12915,10.) ;
#3659=VECTOR('',#12918,10.) ;
#3660=VECTOR('',#12921,10.) ;
#3661=VECTOR('',#12922,10.) ;
#3662=VECTOR('',#12927,10.) ;
#3663=VECTOR('',#12930,10.) ;
#3664=VECTOR('',#12933,10.) ;
#3665=VECTOR('',#12936,10.) ;
#3666=VECTOR('',#12939,10.) ;
#3667=VECTOR('',#12940,10.) ;
#3668=VECTOR('',#12941,10.) ;
#3669=VECTOR('',#12942,10.) ;
#3670=VECTOR('',#12945,10.) ;
#3671=VECTOR('',#12946,10.) ;
#3672=VECTOR('',#12947,10.) ;
#3673=VECTOR('',#12950,10.) ;
#3674=VECTOR('',#12951,10.) ;
#3675=VECTOR('',#12952,10.) ;
#3676=VECTOR('',#12959,10.) ;
#3677=VECTOR('',#12964,10.) ;
#3678=VECTOR('',#12967,10.) ;
#3679=VECTOR('',#12970,10.) ;
#3680=VECTOR('',#12987,10.) ;
#3681=VECTOR('',#12992,10.) ;
#3682=VECTOR('',#12997,0.866025403784434) ;
#3683=VECTOR('',#13000,10.) ;
#3684=VECTOR('',#13003,10.) ;
#3999=CIRCLE('',#10272,0.96675) ;
#4000=CIRCLE('',#10287,0.739000000000001) ;
#4001=CIRCLE('',#10302,0.96675) ;
#4002=CIRCLE('',#10303,0.96675) ;
#4003=CIRCLE('',#10305,0.96675) ;
#4004=CIRCLE('',#10306,0.739000000000001) ;
#4005=CIRCLE('',#10307,0.96675) ;
#4006=CIRCLE('',#10310,0.1) ;
#4007=CIRCLE('',#10311,1.06675) ;
#4008=CIRCLE('',#10313,0.96675) ;
#4009=CIRCLE('',#10315,1.69999999999999) ;
#4010=CIRCLE('',#10317,0.616749999999999) ;
#4011=CIRCLE('',#10320,1.9) ;
#4012=CIRCLE('',#10324,1.9) ;
#4013=CIRCLE('',#10325,1.9) ;
#4014=CIRCLE('',#10326,1.9) ;
#4015=CIRCLE('',#10327,1.9) ;
#4016=CIRCLE('',#10328,1.9) ;
#4017=CIRCLE('',#10329,1.9) ;
#4018=CIRCLE('',#10330,1.9) ;
#4019=CIRCLE('',#10331,1.9) ;
#4020=CIRCLE('',#10332,1.9) ;
#4021=CIRCLE('',#10333,1.9) ;
#4022=CIRCLE('',#10334,1.9) ;
#4023=CIRCLE('',#10335,1.9) ;
#4024=CIRCLE('',#10336,1.9) ;
#4025=CIRCLE('',#10337,1.9) ;
#4026=CIRCLE('',#10338,1.9) ;
#4027=CIRCLE('',#10339,1.9) ;
#4028=CIRCLE('',#10340,1.9) ;
#4029=CIRCLE('',#10341,1.9) ;
#4030=CIRCLE('',#10342,1.9) ;
#4031=CIRCLE('',#10343,1.9) ;
#4032=CIRCLE('',#10344,1.9) ;
#4033=CIRCLE('',#10345,1.9) ;
#4034=CIRCLE('',#10346,1.9) ;
#4035=CIRCLE('',#10347,1.9) ;
#4036=CIRCLE('',#10348,1.9) ;
#4037=CIRCLE('',#10349,1.9) ;
#4038=CIRCLE('',#10350,1.9) ;
#4039=CIRCLE('',#10351,1.9) ;
#4040=CIRCLE('',#10352,1.9) ;
#4041=CIRCLE('',#10353,1.9) ;
#4042=CIRCLE('',#10354,1.9) ;
#4043=CIRCLE('',#10355,1.9) ;
#4044=CIRCLE('',#10356,1.9) ;
#4045=CIRCLE('',#10357,1.9) ;
#4046=CIRCLE('',#10358,1.9) ;
#4047=CIRCLE('',#10359,1.9) ;
#4048=CIRCLE('',#10360,1.9) ;
#4049=CIRCLE('',#10361,1.9) ;
#4050=CIRCLE('',#10362,1.9) ;
#4051=CIRCLE('',#10363,1.9) ;
#4052=CIRCLE('',#10364,1.9) ;
#4053=CIRCLE('',#10365,1.9) ;
#4054=CIRCLE('',#10366,1.9) ;
#4055=CIRCLE('',#10367,1.9) ;
#4056=CIRCLE('',#10368,1.9) ;
#4057=CIRCLE('',#10369,1.9) ;
#4058=CIRCLE('',#10370,1.9) ;
#4059=CIRCLE('',#10371,1.9) ;
#4060=CIRCLE('',#10372,1.9) ;
#4061=CIRCLE('',#10373,1.9) ;
#4062=CIRCLE('',#10374,1.9) ;
#4063=CIRCLE('',#10375,1.9) ;
#4064=CIRCLE('',#10376,1.9) ;
#4065=CIRCLE('',#10377,1.9) ;
#4066=CIRCLE('',#10378,1.9) ;
#4067=CIRCLE('',#10379,1.9) ;
#4068=CIRCLE('',#10380,1.9) ;
#4069=CIRCLE('',#10381,1.9) ;
#4070=CIRCLE('',#10382,1.9) ;
#4071=CIRCLE('',#10383,1.9) ;
#4072=CIRCLE('',#10384,1.9) ;
#4073=CIRCLE('',#10385,1.9) ;
#4074=CIRCLE('',#10386,1.9) ;
#4075=CIRCLE('',#10387,1.9) ;
#4076=CIRCLE('',#10388,1.9) ;
#4077=CIRCLE('',#10389,1.9) ;
#4078=CIRCLE('',#10390,1.9) ;
#4079=CIRCLE('',#10391,1.9) ;
#4080=CIRCLE('',#10392,1.9) ;
#4081=CIRCLE('',#10393,1.9) ;
#4082=CIRCLE('',#10394,1.9) ;
#4083=CIRCLE('',#10395,1.9) ;
#4084=CIRCLE('',#10396,1.9) ;
#4085=CIRCLE('',#10401,1.6) ;
#4086=CIRCLE('',#10505,0.2) ;
#4087=CIRCLE('',#10507,1.01602540378444) ;
#4088=CIRCLE('',#10509,0.816025403784444) ;
#4089=CIRCLE('',#10510,0.816025403784444) ;
#4090=CIRCLE('',#10511,0.816025403784444) ;
#4091=CIRCLE('',#10512,0.816025403784444) ;
#4092=CIRCLE('',#10513,0.816025403784444) ;
#4093=CIRCLE('',#10514,0.816025403784444) ;
#4094=CIRCLE('',#10516,0.816025403784444) ;
#4095=CIRCLE('',#10518,0.816025403784444) ;
#4096=CIRCLE('',#10520,0.816025403784444) ;
#4097=CIRCLE('',#10522,0.816025403784444) ;
#4098=CIRCLE('',#10524,0.816025403784444) ;
#4099=CIRCLE('',#10526,0.816025403784444) ;
#4100=CIRCLE('',#10537,0.866025403784434) ;
#4101=CIRCLE('',#10539,0.866025403784434) ;
#4102=CIRCLE('',#10541,0.866025403784434) ;
#4103=CIRCLE('',#10543,0.866025403784434) ;
#4104=CIRCLE('',#10545,0.866025403784434) ;
#4105=CIRCLE('',#10547,0.866025403784434) ;
#4604=VERTEX_POINT('',#15300) ;
#4605=VERTEX_POINT('',#15301) ;
#4606=VERTEX_POINT('',#15303) ;
#4607=VERTEX_POINT('',#15314) ;
#4608=VERTEX_POINT('',#15324) ;
#4609=VERTEX_POINT('',#15325) ;
#4610=VERTEX_POINT('',#15372) ;
#4611=VERTEX_POINT('',#15373) ;
#4612=VERTEX_POINT('',#15420) ;
#4613=VERTEX_POINT('',#15421) ;
#4614=VERTEX_POINT('',#15474) ;
#4615=VERTEX_POINT('',#15475) ;
#4616=VERTEX_POINT('',#15522) ;
#4617=VERTEX_POINT('',#15523) ;
#4618=VERTEX_POINT('',#15570) ;
#4619=VERTEX_POINT('',#15571) ;
#4620=VERTEX_POINT('',#15624) ;
#4621=VERTEX_POINT('',#15625) ;
#4622=VERTEX_POINT('',#15672) ;
#4623=VERTEX_POINT('',#15673) ;
#4624=VERTEX_POINT('',#15720) ;
#4625=VERTEX_POINT('',#15721) ;
#4626=VERTEX_POINT('',#15774) ;
#4627=VERTEX_POINT('',#15775) ;
#4628=VERTEX_POINT('',#15822) ;
#4629=VERTEX_POINT('',#15823) ;
#4630=VERTEX_POINT('',#15870) ;
#4631=VERTEX_POINT('',#15871) ;
#4632=VERTEX_POINT('',#15924) ;
#4633=VERTEX_POINT('',#15925) ;
#4634=VERTEX_POINT('',#15972) ;
#4635=VERTEX_POINT('',#15973) ;
#4636=VERTEX_POINT('',#15975) ;
#4637=VERTEX_POINT('',#15981) ;
#4638=VERTEX_POINT('',#15988) ;
#4639=VERTEX_POINT('',#15989) ;
#4640=VERTEX_POINT('',#16012) ;
#4641=VERTEX_POINT('',#16013) ;
#4642=VERTEX_POINT('',#16037) ;
#4643=VERTEX_POINT('',#16038) ;
#4644=VERTEX_POINT('',#16062) ;
#4645=VERTEX_POINT('',#16063) ;
#4646=VERTEX_POINT('',#16086) ;
#4647=VERTEX_POINT('',#16087) ;
#4648=VERTEX_POINT('',#16111) ;
#4649=VERTEX_POINT('',#16112) ;
#4650=VERTEX_POINT('',#16136) ;
#4651=VERTEX_POINT('',#16137) ;
#4652=VERTEX_POINT('',#16160) ;
#4653=VERTEX_POINT('',#16161) ;
#4654=VERTEX_POINT('',#16185) ;
#4655=VERTEX_POINT('',#16186) ;
#4656=VERTEX_POINT('',#16210) ;
#4657=VERTEX_POINT('',#16211) ;
#4658=VERTEX_POINT('',#16234) ;
#4659=VERTEX_POINT('',#16235) ;
#4660=VERTEX_POINT('',#16259) ;
#4661=VERTEX_POINT('',#16260) ;
#4662=VERTEX_POINT('',#16284) ;
#4663=VERTEX_POINT('',#16285) ;
#4664=VERTEX_POINT('',#16308) ;
#4665=VERTEX_POINT('',#16382) ;
#4666=VERTEX_POINT('',#16384) ;
#4667=VERTEX_POINT('',#16850) ;
#4668=VERTEX_POINT('',#16934) ;
#4669=VERTEX_POINT('',#16936) ;
#4670=VERTEX_POINT('',#17410) ;
#4671=VERTEX_POINT('',#17416) ;
#4672=VERTEX_POINT('',#17419) ;
#4673=VERTEX_POINT('',#17424) ;
#4674=VERTEX_POINT('',#17425) ;
#4675=VERTEX_POINT('',#17427) ;
#4676=VERTEX_POINT('',#17431) ;
#4677=VERTEX_POINT('',#17433) ;
#4678=VERTEX_POINT('',#17439) ;
#4679=VERTEX_POINT('',#17445) ;
#4680=VERTEX_POINT('',#17447) ;
#4681=VERTEX_POINT('',#17449) ;
#4682=VERTEX_POINT('',#17451) ;
#4683=VERTEX_POINT('',#17453) ;
#4684=VERTEX_POINT('',#17455) ;
#4685=VERTEX_POINT('',#17457) ;
#4686=VERTEX_POINT('',#17459) ;
#4687=VERTEX_POINT('',#17461) ;
#4688=VERTEX_POINT('',#17463) ;
#4689=VERTEX_POINT('',#17465) ;
#4690=VERTEX_POINT('',#17467) ;
#4691=VERTEX_POINT('',#17469) ;
#4692=VERTEX_POINT('',#17471) ;
#4693=VERTEX_POINT('',#17473) ;
#4694=VERTEX_POINT('',#17475) ;
#4695=VERTEX_POINT('',#17477) ;
#4696=VERTEX_POINT('',#17479) ;
#4697=VERTEX_POINT('',#17481) ;
#4698=VERTEX_POINT('',#17483) ;
#4699=VERTEX_POINT('',#17485) ;
#4700=VERTEX_POINT('',#17487) ;
#4701=VERTEX_POINT('',#17489) ;
#4702=VERTEX_POINT('',#17491) ;
#4703=VERTEX_POINT('',#17493) ;
#4704=VERTEX_POINT('',#17495) ;
#4705=VERTEX_POINT('',#17497) ;
#4706=VERTEX_POINT('',#17499) ;
#4707=VERTEX_POINT('',#17501) ;
#4708=VERTEX_POINT('',#17503) ;
#4709=VERTEX_POINT('',#17505) ;
#4710=VERTEX_POINT('',#17507) ;
#4711=VERTEX_POINT('',#17509) ;
#4712=VERTEX_POINT('',#17511) ;
#4713=VERTEX_POINT('',#17513) ;
#4714=VERTEX_POINT('',#17515) ;
#4715=VERTEX_POINT('',#17517) ;
#4716=VERTEX_POINT('',#17519) ;
#4717=VERTEX_POINT('',#17521) ;
#4718=VERTEX_POINT('',#17523) ;
#4719=VERTEX_POINT('',#17525) ;
#4720=VERTEX_POINT('',#17527) ;
#4721=VERTEX_POINT('',#17529) ;
#4722=VERTEX_POINT('',#17531) ;
#4723=VERTEX_POINT('',#17533) ;
#4724=VERTEX_POINT('',#17535) ;
#4725=VERTEX_POINT('',#17537) ;
#4726=VERTEX_POINT('',#17539) ;
#4727=VERTEX_POINT('',#17541) ;
#4728=VERTEX_POINT('',#17543) ;
#4729=VERTEX_POINT('',#17545) ;
#4730=VERTEX_POINT('',#17547) ;
#4731=VERTEX_POINT('',#17549) ;
#4732=VERTEX_POINT('',#17551) ;
#4733=VERTEX_POINT('',#17553) ;
#4734=VERTEX_POINT('',#17555) ;
#4735=VERTEX_POINT('',#17557) ;
#4736=VERTEX_POINT('',#17559) ;
#4737=VERTEX_POINT('',#17561) ;
#4738=VERTEX_POINT('',#17563) ;
#4739=VERTEX_POINT('',#17565) ;
#4740=VERTEX_POINT('',#17567) ;
#4741=VERTEX_POINT('',#17569) ;
#4742=VERTEX_POINT('',#17571) ;
#4743=VERTEX_POINT('',#17573) ;
#4744=VERTEX_POINT('',#17575) ;
#4745=VERTEX_POINT('',#17577) ;
#4746=VERTEX_POINT('',#17579) ;
#4747=VERTEX_POINT('',#17581) ;
#4748=VERTEX_POINT('',#17583) ;
#4749=VERTEX_POINT('',#17585) ;
#4750=VERTEX_POINT('',#17587) ;
#4751=VERTEX_POINT('',#17589) ;
#4752=VERTEX_POINT('',#17591) ;
#4753=VERTEX_POINT('',#17593) ;
#4754=VERTEX_POINT('',#17595) ;
#4755=VERTEX_POINT('',#17598) ;
#4756=VERTEX_POINT('',#17600) ;
#4757=VERTEX_POINT('',#17602) ;
#4758=VERTEX_POINT('',#17604) ;
#4759=VERTEX_POINT('',#17606) ;
#4760=VERTEX_POINT('',#17608) ;
#4761=VERTEX_POINT('',#17610) ;
#4762=VERTEX_POINT('',#17612) ;
#4763=VERTEX_POINT('',#17614) ;
#4764=VERTEX_POINT('',#17616) ;
#4765=VERTEX_POINT('',#17618) ;
#4766=VERTEX_POINT('',#17620) ;
#4767=VERTEX_POINT('',#17622) ;
#4768=VERTEX_POINT('',#17624) ;
#4769=VERTEX_POINT('',#17626) ;
#4770=VERTEX_POINT('',#17628) ;
#4771=VERTEX_POINT('',#17630) ;
#4772=VERTEX_POINT('',#17632) ;
#4773=VERTEX_POINT('',#17634) ;
#4774=VERTEX_POINT('',#17636) ;
#4775=VERTEX_POINT('',#17638) ;
#4776=VERTEX_POINT('',#17640) ;
#4777=VERTEX_POINT('',#17642) ;
#4778=VERTEX_POINT('',#17644) ;
#4779=VERTEX_POINT('',#17646) ;
#4780=VERTEX_POINT('',#17648) ;
#4781=VERTEX_POINT('',#17650) ;
#4782=VERTEX_POINT('',#17652) ;
#4783=VERTEX_POINT('',#17654) ;
#4784=VERTEX_POINT('',#17656) ;
#4785=VERTEX_POINT('',#17658) ;
#4786=VERTEX_POINT('',#17660) ;
#4787=VERTEX_POINT('',#17662) ;
#4788=VERTEX_POINT('',#17664) ;
#4789=VERTEX_POINT('',#17666) ;
#4790=VERTEX_POINT('',#17668) ;
#4791=VERTEX_POINT('',#17670) ;
#4792=VERTEX_POINT('',#17672) ;
#4793=VERTEX_POINT('',#17674) ;
#4794=VERTEX_POINT('',#17676) ;
#4795=VERTEX_POINT('',#17678) ;
#4796=VERTEX_POINT('',#17680) ;
#4797=VERTEX_POINT('',#17682) ;
#4798=VERTEX_POINT('',#17684) ;
#4799=VERTEX_POINT('',#17686) ;
#4800=VERTEX_POINT('',#17688) ;
#4801=VERTEX_POINT('',#17690) ;
#4802=VERTEX_POINT('',#17692) ;
#4803=VERTEX_POINT('',#17694) ;
#4804=VERTEX_POINT('',#17696) ;
#4805=VERTEX_POINT('',#17698) ;
#4806=VERTEX_POINT('',#17700) ;
#4807=VERTEX_POINT('',#17702) ;
#4808=VERTEX_POINT('',#17704) ;
#4809=VERTEX_POINT('',#17706) ;
#4810=VERTEX_POINT('',#17708) ;
#4811=VERTEX_POINT('',#17710) ;
#4812=VERTEX_POINT('',#17712) ;
#4813=VERTEX_POINT('',#17714) ;
#4814=VERTEX_POINT('',#17716) ;
#4815=VERTEX_POINT('',#17718) ;
#4816=VERTEX_POINT('',#17720) ;
#4817=VERTEX_POINT('',#17722) ;
#4818=VERTEX_POINT('',#17724) ;
#4819=VERTEX_POINT('',#17726) ;
#4820=VERTEX_POINT('',#17728) ;
#4821=VERTEX_POINT('',#17732) ;
#4822=VERTEX_POINT('',#17734) ;
#4823=VERTEX_POINT('',#17746) ;
#4824=VERTEX_POINT('',#17748) ;
#4825=VERTEX_POINT('',#17753) ;
#4826=VERTEX_POINT('',#17760) ;
#4827=VERTEX_POINT('',#17767) ;
#4828=VERTEX_POINT('',#17774) ;
#4829=VERTEX_POINT('',#17781) ;
#4830=VERTEX_POINT('',#17788) ;
#4831=VERTEX_POINT('',#17795) ;
#4832=VERTEX_POINT('',#17802) ;
#4833=VERTEX_POINT('',#17809) ;
#4834=VERTEX_POINT('',#17816) ;
#4835=VERTEX_POINT('',#17823) ;
#4836=VERTEX_POINT('',#17830) ;
#4837=VERTEX_POINT('',#17837) ;
#4838=VERTEX_POINT('',#17844) ;
#4839=VERTEX_POINT('',#17851) ;
#4840=VERTEX_POINT('',#17858) ;
#4841=VERTEX_POINT('',#17865) ;
#4842=VERTEX_POINT('',#17872) ;
#4843=VERTEX_POINT('',#17879) ;
#4844=VERTEX_POINT('',#17886) ;
#4845=VERTEX_POINT('',#17893) ;
#4846=VERTEX_POINT('',#17900) ;
#4847=VERTEX_POINT('',#17907) ;
#4848=VERTEX_POINT('',#17914) ;
#4849=VERTEX_POINT('',#17921) ;
#4850=VERTEX_POINT('',#17928) ;
#4851=VERTEX_POINT('',#17935) ;
#4852=VERTEX_POINT('',#17942) ;
#4853=VERTEX_POINT('',#17949) ;
#4854=VERTEX_POINT('',#17956) ;
#4855=VERTEX_POINT('',#17963) ;
#4856=VERTEX_POINT('',#17970) ;
#4857=VERTEX_POINT('',#17977) ;
#4858=VERTEX_POINT('',#17988) ;
#4859=VERTEX_POINT('',#17995) ;
#4860=VERTEX_POINT('',#18002) ;
#4861=VERTEX_POINT('',#18009) ;
#4862=VERTEX_POINT('',#18016) ;
#4863=VERTEX_POINT('',#18023) ;
#4864=VERTEX_POINT('',#18030) ;
#4865=VERTEX_POINT('',#18037) ;
#4866=VERTEX_POINT('',#18044) ;
#4867=VERTEX_POINT('',#18051) ;
#4868=VERTEX_POINT('',#18058) ;
#4869=VERTEX_POINT('',#18065) ;
#4870=VERTEX_POINT('',#18072) ;
#4871=VERTEX_POINT('',#18079) ;
#4872=VERTEX_POINT('',#18086) ;
#4873=VERTEX_POINT('',#18093) ;
#4874=VERTEX_POINT('',#18100) ;
#4875=VERTEX_POINT('',#18107) ;
#4876=VERTEX_POINT('',#18114) ;
#4877=VERTEX_POINT('',#18121) ;
#4878=VERTEX_POINT('',#18128) ;
#4879=VERTEX_POINT('',#18135) ;
#4880=VERTEX_POINT('',#18142) ;
#4881=VERTEX_POINT('',#18149) ;
#4882=VERTEX_POINT('',#18156) ;
#4883=VERTEX_POINT('',#18163) ;
#4884=VERTEX_POINT('',#18170) ;
#4885=VERTEX_POINT('',#18177) ;
#4886=VERTEX_POINT('',#18184) ;
#4887=VERTEX_POINT('',#18191) ;
#4888=VERTEX_POINT('',#18198) ;
#4889=VERTEX_POINT('',#18205) ;
#4890=VERTEX_POINT('',#18212) ;
#4891=VERTEX_POINT('',#18219) ;
#4892=VERTEX_POINT('',#18228) ;
#4893=VERTEX_POINT('',#18231) ;
#4894=VERTEX_POINT('',#18233) ;
#4895=VERTEX_POINT('',#18237) ;
#4896=VERTEX_POINT('',#18239) ;
#4897=VERTEX_POINT('',#18243) ;
#4898=VERTEX_POINT('',#18247) ;
#4899=VERTEX_POINT('',#18249) ;
#4900=VERTEX_POINT('',#18253) ;
#4901=VERTEX_POINT('',#18257) ;
#4902=VERTEX_POINT('',#18259) ;
#4903=VERTEX_POINT('',#18263) ;
#4904=VERTEX_POINT('',#18267) ;
#4905=VERTEX_POINT('',#18269) ;
#4906=VERTEX_POINT('',#18273) ;
#4907=VERTEX_POINT('',#18277) ;
#4908=VERTEX_POINT('',#18279) ;
#4909=VERTEX_POINT('',#18283) ;
#4910=VERTEX_POINT('',#18287) ;
#4911=VERTEX_POINT('',#18293) ;
#4912=VERTEX_POINT('',#18295) ;
#4913=VERTEX_POINT('',#18299) ;
#4914=VERTEX_POINT('',#18301) ;
#4915=VERTEX_POINT('',#18305) ;
#4916=VERTEX_POINT('',#18307) ;
#4917=VERTEX_POINT('',#18311) ;
#4918=VERTEX_POINT('',#18313) ;
#4919=VERTEX_POINT('',#18317) ;
#4920=VERTEX_POINT('',#18319) ;
#4921=VERTEX_POINT('',#18323) ;
#4922=VERTEX_POINT('',#18325) ;
#4923=VERTEX_POINT('',#18330) ;
#4924=VERTEX_POINT('',#18332) ;
#4925=VERTEX_POINT('',#18337) ;
#4926=VERTEX_POINT('',#18342) ;
#4927=VERTEX_POINT('',#18355) ;
#4928=VERTEX_POINT('',#18365) ;
#4929=VERTEX_POINT('',#18372) ;
#5711=EDGE_CURVE('',#4604,#4605,#2671,.T.) ;
#5712=EDGE_CURVE('',#4604,#4606,#436,.T.) ;
#5713=EDGE_CURVE('',#4607,#4606,#3999,.T.) ;
#5714=EDGE_CURVE('',#4607,#4605,#437,.T.) ;
#5715=EDGE_CURVE('',#4608,#4609,#2672,.T.) ;
#5716=EDGE_CURVE('',#4608,#4604,#438,.T.) ;
#5717=EDGE_CURVE('',#4605,#4609,#439,.T.) ;
#5718=EDGE_CURVE('',#4610,#4611,#2673,.T.) ;
#5719=EDGE_CURVE('',#4610,#4608,#440,.T.) ;
#5720=EDGE_CURVE('',#4609,#4611,#441,.T.) ;
#5721=EDGE_CURVE('',#4612,#4613,#2674,.T.) ;
#5722=EDGE_CURVE('',#4612,#4610,#442,.T.) ;
#5723=EDGE_CURVE('',#4611,#4613,#443,.T.) ;
#5724=EDGE_CURVE('',#4614,#4615,#2675,.T.) ;
#5725=EDGE_CURVE('',#4614,#4612,#444,.T.) ;
#5726=EDGE_CURVE('',#4613,#4615,#445,.T.) ;
#5727=EDGE_CURVE('',#4616,#4617,#2676,.T.) ;
#5728=EDGE_CURVE('',#4616,#4614,#446,.T.) ;
#5729=EDGE_CURVE('',#4615,#4617,#447,.T.) ;
#5730=EDGE_CURVE('',#4618,#4619,#2677,.T.) ;
#5731=EDGE_CURVE('',#4618,#4616,#448,.T.) ;
#5732=EDGE_CURVE('',#4617,#4619,#449,.T.) ;
#5733=EDGE_CURVE('',#4620,#4621,#2678,.T.) ;
#5734=EDGE_CURVE('',#4620,#4618,#450,.T.) ;
#5735=EDGE_CURVE('',#4619,#4621,#451,.T.) ;
#5736=EDGE_CURVE('',#4622,#4623,#2679,.T.) ;
#5737=EDGE_CURVE('',#4622,#4620,#452,.T.) ;
#5738=EDGE_CURVE('',#4621,#4623,#453,.T.) ;
#5739=EDGE_CURVE('',#4624,#4625,#2680,.T.) ;
#5740=EDGE_CURVE('',#4624,#4622,#454,.T.) ;
#5741=EDGE_CURVE('',#4623,#4625,#455,.T.) ;
#5742=EDGE_CURVE('',#4626,#4627,#2681,.T.) ;
#5743=EDGE_CURVE('',#4626,#4624,#456,.T.) ;
#5744=EDGE_CURVE('',#4625,#4627,#457,.T.) ;
#5745=EDGE_CURVE('',#4628,#4629,#2682,.T.) ;
#5746=EDGE_CURVE('',#4628,#4626,#458,.T.) ;
#5747=EDGE_CURVE('',#4627,#4629,#459,.T.) ;
#5748=EDGE_CURVE('',#4630,#4631,#2683,.T.) ;
#5749=EDGE_CURVE('',#4630,#4628,#460,.T.) ;
#5750=EDGE_CURVE('',#4629,#4631,#461,.T.) ;
#5751=EDGE_CURVE('',#4632,#4633,#2684,.T.) ;
#5752=EDGE_CURVE('',#4632,#4630,#462,.T.) ;
#5753=EDGE_CURVE('',#4631,#4633,#463,.T.) ;
#5754=EDGE_CURVE('',#4634,#4635,#2685,.T.) ;
#5755=EDGE_CURVE('',#4634,#4636,#464,.T.) ;
#5756=EDGE_CURVE('',#4637,#4636,#4000,.T.) ;
#5757=EDGE_CURVE('',#4635,#4637,#465,.T.) ;
#5758=EDGE_CURVE('',#4638,#4639,#2686,.T.) ;
#5759=EDGE_CURVE('',#4638,#4634,#466,.T.) ;
#5760=EDGE_CURVE('',#4639,#4635,#467,.T.) ;
#5761=EDGE_CURVE('',#4640,#4641,#2687,.T.) ;
#5762=EDGE_CURVE('',#4640,#4638,#468,.T.) ;
#5763=EDGE_CURVE('',#4641,#4639,#469,.T.) ;
#5764=EDGE_CURVE('',#4642,#4643,#2688,.T.) ;
#5765=EDGE_CURVE('',#4642,#4640,#470,.T.) ;
#5766=EDGE_CURVE('',#4643,#4641,#471,.T.) ;
#5767=EDGE_CURVE('',#4644,#4645,#2689,.T.) ;
#5768=EDGE_CURVE('',#4644,#4642,#472,.T.) ;
#5769=EDGE_CURVE('',#4645,#4643,#473,.T.) ;
#5770=EDGE_CURVE('',#4646,#4647,#2690,.T.) ;
#5771=EDGE_CURVE('',#4646,#4644,#474,.T.) ;
#5772=EDGE_CURVE('',#4647,#4645,#475,.T.) ;
#5773=EDGE_CURVE('',#4648,#4649,#2691,.T.) ;
#5774=EDGE_CURVE('',#4648,#4646,#476,.T.) ;
#5775=EDGE_CURVE('',#4649,#4647,#477,.T.) ;
#5776=EDGE_CURVE('',#4650,#4651,#2692,.T.) ;
#5777=EDGE_CURVE('',#4650,#4648,#478,.T.) ;
#5778=EDGE_CURVE('',#4651,#4649,#479,.T.) ;
#5779=EDGE_CURVE('',#4652,#4653,#2693,.T.) ;
#5780=EDGE_CURVE('',#4652,#4650,#480,.T.) ;
#5781=EDGE_CURVE('',#4653,#4651,#481,.T.) ;
#5782=EDGE_CURVE('',#4654,#4655,#2694,.T.) ;
#5783=EDGE_CURVE('',#4654,#4652,#482,.T.) ;
#5784=EDGE_CURVE('',#4655,#4653,#483,.T.) ;
#5785=EDGE_CURVE('',#4656,#4657,#2695,.T.) ;
#5786=EDGE_CURVE('',#4656,#4654,#484,.T.) ;
#5787=EDGE_CURVE('',#4657,#4655,#485,.T.) ;
#5788=EDGE_CURVE('',#4658,#4659,#2696,.T.) ;
#5789=EDGE_CURVE('',#4658,#4656,#486,.T.) ;
#5790=EDGE_CURVE('',#4659,#4657,#487,.T.) ;
#5791=EDGE_CURVE('',#4660,#4661,#2697,.T.) ;
#5792=EDGE_CURVE('',#4660,#4658,#488,.T.) ;
#5793=EDGE_CURVE('',#4661,#4659,#489,.T.) ;
#5794=EDGE_CURVE('',#4662,#4663,#2698,.T.) ;
#5795=EDGE_CURVE('',#4662,#4660,#490,.T.) ;
#5796=EDGE_CURVE('',#4663,#4661,#491,.T.) ;
#5797=EDGE_CURVE('',#4636,#4664,#492,.T.) ;
#5798=EDGE_CURVE('',#4665,#4664,#4001,.T.) ;
#5799=EDGE_CURVE('',#4666,#4665,#4002,.T.) ;
#5800=EDGE_CURVE('',#4666,#4637,#493,.T.) ;
#5801=EDGE_CURVE('',#4633,#4666,#494,.T.) ;
#5802=EDGE_CURVE('',#4667,#4607,#495,.T.) ;
#5803=EDGE_CURVE('',#4667,#4663,#496,.T.) ;
#5804=EDGE_CURVE('',#4606,#4668,#4003,.T.) ;
#5805=EDGE_CURVE('',#4606,#4669,#497,.T.) ;
#5806=EDGE_CURVE('',#4669,#4667,#4004,.T.) ;
#5807=EDGE_CURVE('',#4668,#4607,#4005,.T.) ;
#5808=EDGE_CURVE('',#4669,#4662,#498,.T.) ;
#5809=EDGE_CURVE('',#4664,#4632,#499,.T.) ;
#5810=EDGE_CURVE('',#4668,#4670,#4006,.T.) ;
#5811=EDGE_CURVE('',#4670,#4670,#4007,.T.) ;
#5812=EDGE_CURVE('',#4664,#4666,#4008,.T.) ;
#5813=EDGE_CURVE('',#4671,#4671,#4009,.T.) ;
#5814=EDGE_CURVE('',#4665,#4672,#2699,.T.) ;
#5815=EDGE_CURVE('',#4672,#4672,#4010,.T.) ;
#5816=EDGE_CURVE('',#4673,#4674,#4011,.T.) ;
#5817=EDGE_CURVE('',#4675,#4673,#2700,.T.) ;
#5818=EDGE_CURVE('',#4674,#4675,#2701,.T.) ;
#5819=EDGE_CURVE('',#4674,#4676,#2702,.T.) ;
#5820=EDGE_CURVE('',#4677,#4675,#2703,.T.) ;
#5821=EDGE_CURVE('',#4676,#4677,#247,.T.) ;
#5822=EDGE_CURVE('',#4678,#4673,#2704,.T.) ;
#5823=EDGE_CURVE('',#4677,#4678,#248,.T.) ;
#5824=EDGE_CURVE('',#4679,#4676,#4012,.T.) ;
#5825=EDGE_CURVE('',#4679,#4680,#2705,.T.) ;
#5826=EDGE_CURVE('',#4680,#4681,#4013,.T.) ;
#5827=EDGE_CURVE('',#4681,#4682,#2706,.T.) ;
#5828=EDGE_CURVE('',#4683,#4682,#4014,.T.) ;
#5829=EDGE_CURVE('',#4683,#4684,#2707,.T.) ;
#5830=EDGE_CURVE('',#4684,#4685,#4015,.T.) ;
#5831=EDGE_CURVE('',#4685,#4686,#2708,.T.) ;
#5832=EDGE_CURVE('',#4687,#4686,#4016,.T.) ;
#5833=EDGE_CURVE('',#4687,#4688,#2709,.T.) ;
#5834=EDGE_CURVE('',#4688,#4689,#4017,.T.) ;
#5835=EDGE_CURVE('',#4689,#4690,#2710,.T.) ;
#5836=EDGE_CURVE('',#4691,#4690,#4018,.T.) ;
#5837=EDGE_CURVE('',#4691,#4692,#2711,.T.) ;
#5838=EDGE_CURVE('',#4692,#4693,#4019,.T.) ;
#5839=EDGE_CURVE('',#4693,#4694,#2712,.T.) ;
#5840=EDGE_CURVE('',#4695,#4694,#4020,.T.) ;
#5841=EDGE_CURVE('',#4695,#4696,#2713,.T.) ;
#5842=EDGE_CURVE('',#4696,#4697,#4021,.T.) ;
#5843=EDGE_CURVE('',#4697,#4698,#2714,.T.) ;
#5844=EDGE_CURVE('',#4699,#4698,#4022,.T.) ;
#5845=EDGE_CURVE('',#4699,#4700,#2715,.T.) ;
#5846=EDGE_CURVE('',#4700,#4701,#4023,.T.) ;
#5847=EDGE_CURVE('',#4701,#4702,#2716,.T.) ;
#5848=EDGE_CURVE('',#4703,#4702,#4024,.T.) ;
#5849=EDGE_CURVE('',#4703,#4704,#2717,.T.) ;
#5850=EDGE_CURVE('',#4704,#4705,#4025,.T.) ;
#5851=EDGE_CURVE('',#4705,#4706,#2718,.T.) ;
#5852=EDGE_CURVE('',#4707,#4706,#4026,.T.) ;
#5853=EDGE_CURVE('',#4707,#4708,#2719,.T.) ;
#5854=EDGE_CURVE('',#4708,#4709,#4027,.T.) ;
#5855=EDGE_CURVE('',#4709,#4710,#2720,.T.) ;
#5856=EDGE_CURVE('',#4711,#4710,#4028,.T.) ;
#5857=EDGE_CURVE('',#4711,#4712,#2721,.T.) ;
#5858=EDGE_CURVE('',#4712,#4713,#4029,.T.) ;
#5859=EDGE_CURVE('',#4713,#4714,#2722,.T.) ;
#5860=EDGE_CURVE('',#4715,#4714,#4030,.T.) ;
#5861=EDGE_CURVE('',#4715,#4716,#2723,.T.) ;
#5862=EDGE_CURVE('',#4716,#4717,#4031,.T.) ;
#5863=EDGE_CURVE('',#4717,#4718,#2724,.T.) ;
#5864=EDGE_CURVE('',#4719,#4718,#4032,.T.) ;
#5865=EDGE_CURVE('',#4719,#4720,#2725,.T.) ;
#5866=EDGE_CURVE('',#4720,#4721,#4033,.T.) ;
#5867=EDGE_CURVE('',#4721,#4722,#2726,.T.) ;
#5868=EDGE_CURVE('',#4723,#4722,#4034,.T.) ;
#5869=EDGE_CURVE('',#4723,#4724,#2727,.T.) ;
#5870=EDGE_CURVE('',#4724,#4725,#4035,.T.) ;
#5871=EDGE_CURVE('',#4725,#4726,#2728,.T.) ;
#5872=EDGE_CURVE('',#4727,#4726,#4036,.T.) ;
#5873=EDGE_CURVE('',#4727,#4728,#2729,.T.) ;
#5874=EDGE_CURVE('',#4728,#4729,#4037,.T.) ;
#5875=EDGE_CURVE('',#4729,#4730,#2730,.T.) ;
#5876=EDGE_CURVE('',#4731,#4730,#4038,.T.) ;
#5877=EDGE_CURVE('',#4731,#4732,#2731,.T.) ;
#5878=EDGE_CURVE('',#4732,#4733,#4039,.T.) ;
#5879=EDGE_CURVE('',#4733,#4734,#2732,.T.) ;
#5880=EDGE_CURVE('',#4735,#4734,#4040,.T.) ;
#5881=EDGE_CURVE('',#4735,#4736,#2733,.T.) ;
#5882=EDGE_CURVE('',#4736,#4737,#4041,.T.) ;
#5883=EDGE_CURVE('',#4737,#4738,#2734,.T.) ;
#5884=EDGE_CURVE('',#4739,#4738,#4042,.T.) ;
#5885=EDGE_CURVE('',#4739,#4740,#2735,.T.) ;
#5886=EDGE_CURVE('',#4740,#4741,#4043,.T.) ;
#5887=EDGE_CURVE('',#4741,#4742,#2736,.T.) ;
#5888=EDGE_CURVE('',#4743,#4742,#4044,.T.) ;
#5889=EDGE_CURVE('',#4743,#4744,#2737,.T.) ;
#5890=EDGE_CURVE('',#4744,#4745,#4045,.T.) ;
#5891=EDGE_CURVE('',#4745,#4746,#2738,.T.) ;
#5892=EDGE_CURVE('',#4747,#4746,#4046,.T.) ;
#5893=EDGE_CURVE('',#4747,#4748,#2739,.T.) ;
#5894=EDGE_CURVE('',#4748,#4749,#4047,.T.) ;
#5895=EDGE_CURVE('',#4749,#4750,#2740,.T.) ;
#5896=EDGE_CURVE('',#4751,#4750,#4048,.T.) ;
#5897=EDGE_CURVE('',#4751,#4752,#2741,.T.) ;
#5898=EDGE_CURVE('',#4752,#4753,#4049,.T.) ;
#5899=EDGE_CURVE('',#4753,#4754,#2742,.T.) ;
#5900=EDGE_CURVE('',#4754,#4754,#4050,.T.) ;
#5901=EDGE_CURVE('',#4753,#4755,#4051,.T.) ;
#5902=EDGE_CURVE('',#4755,#4756,#2743,.T.) ;
#5903=EDGE_CURVE('',#4757,#4756,#4052,.T.) ;
#5904=EDGE_CURVE('',#4757,#4758,#2744,.T.) ;
#5905=EDGE_CURVE('',#4758,#4759,#4053,.T.) ;
#5906=EDGE_CURVE('',#4759,#4760,#2745,.T.) ;
#5907=EDGE_CURVE('',#4761,#4760,#4054,.T.) ;
#5908=EDGE_CURVE('',#4761,#4762,#2746,.T.) ;
#5909=EDGE_CURVE('',#4762,#4763,#4055,.T.) ;
#5910=EDGE_CURVE('',#4763,#4764,#2747,.T.) ;
#5911=EDGE_CURVE('',#4765,#4764,#4056,.T.) ;
#5912=EDGE_CURVE('',#4765,#4766,#2748,.T.) ;
#5913=EDGE_CURVE('',#4766,#4767,#4057,.T.) ;
#5914=EDGE_CURVE('',#4767,#4768,#2749,.T.) ;
#5915=EDGE_CURVE('',#4769,#4768,#4058,.T.) ;
#5916=EDGE_CURVE('',#4769,#4770,#2750,.T.) ;
#5917=EDGE_CURVE('',#4770,#4771,#4059,.T.) ;
#5918=EDGE_CURVE('',#4771,#4772,#2751,.T.) ;
#5919=EDGE_CURVE('',#4773,#4772,#4060,.T.) ;
#5920=EDGE_CURVE('',#4773,#4774,#2752,.T.) ;
#5921=EDGE_CURVE('',#4774,#4775,#4061,.T.) ;
#5922=EDGE_CURVE('',#4775,#4776,#2753,.T.) ;
#5923=EDGE_CURVE('',#4777,#4776,#4062,.T.) ;
#5924=EDGE_CURVE('',#4777,#4778,#2754,.T.) ;
#5925=EDGE_CURVE('',#4778,#4779,#4063,.T.) ;
#5926=EDGE_CURVE('',#4779,#4780,#2755,.T.) ;
#5927=EDGE_CURVE('',#4781,#4780,#4064,.T.) ;
#5928=EDGE_CURVE('',#4781,#4782,#2756,.T.) ;
#5929=EDGE_CURVE('',#4782,#4783,#4065,.T.) ;
#5930=EDGE_CURVE('',#4783,#4784,#2757,.T.) ;
#5931=EDGE_CURVE('',#4785,#4784,#4066,.T.) ;
#5932=EDGE_CURVE('',#4785,#4786,#2758,.T.) ;
#5933=EDGE_CURVE('',#4786,#4787,#4067,.T.) ;
#5934=EDGE_CURVE('',#4787,#4788,#2759,.T.) ;
#5935=EDGE_CURVE('',#4789,#4788,#4068,.T.) ;
#5936=EDGE_CURVE('',#4789,#4790,#2760,.T.) ;
#5937=EDGE_CURVE('',#4790,#4791,#4069,.T.) ;
#5938=EDGE_CURVE('',#4791,#4792,#2761,.T.) ;
#5939=EDGE_CURVE('',#4793,#4792,#4070,.T.) ;
#5940=EDGE_CURVE('',#4793,#4794,#2762,.T.) ;
#5941=EDGE_CURVE('',#4794,#4795,#4071,.T.) ;
#5942=EDGE_CURVE('',#4795,#4796,#2763,.T.) ;
#5943=EDGE_CURVE('',#4797,#4796,#4072,.T.) ;
#5944=EDGE_CURVE('',#4797,#4798,#2764,.T.) ;
#5945=EDGE_CURVE('',#4798,#4799,#4073,.T.) ;
#5946=EDGE_CURVE('',#4799,#4800,#2765,.T.) ;
#5947=EDGE_CURVE('',#4801,#4800,#4074,.T.) ;
#5948=EDGE_CURVE('',#4801,#4802,#2766,.T.) ;
#5949=EDGE_CURVE('',#4802,#4803,#4075,.T.) ;
#5950=EDGE_CURVE('',#4803,#4804,#2767,.T.) ;
#5951=EDGE_CURVE('',#4805,#4804,#4076,.T.) ;
#5952=EDGE_CURVE('',#4805,#4806,#2768,.T.) ;
#5953=EDGE_CURVE('',#4806,#4807,#4077,.T.) ;
#5954=EDGE_CURVE('',#4807,#4808,#2769,.T.) ;
#5955=EDGE_CURVE('',#4809,#4808,#4078,.T.) ;
#5956=EDGE_CURVE('',#4809,#4810,#2770,.T.) ;
#5957=EDGE_CURVE('',#4810,#4811,#4079,.T.) ;
#5958=EDGE_CURVE('',#4811,#4812,#2771,.T.) ;
#5959=EDGE_CURVE('',#4813,#4812,#4080,.T.) ;
#5960=EDGE_CURVE('',#4813,#4814,#2772,.T.) ;
#5961=EDGE_CURVE('',#4814,#4815,#4081,.T.) ;
#5962=EDGE_CURVE('',#4815,#4816,#2773,.T.) ;
#5963=EDGE_CURVE('',#4817,#4816,#4082,.T.) ;
#5964=EDGE_CURVE('',#4817,#4818,#2774,.T.) ;
#5965=EDGE_CURVE('',#4818,#4819,#4083,.T.) ;
#5966=EDGE_CURVE('',#4819,#4820,#2775,.T.) ;
#5967=EDGE_CURVE('',#4678,#4820,#4084,.T.) ;
#5968=EDGE_CURVE('',#4819,#4821,#2776,.T.) ;
#5969=EDGE_CURVE('',#4822,#4821,#2777,.T.) ;
#5970=EDGE_CURVE('',#4820,#4822,#249,.T.) ;
#5971=EDGE_CURVE('',#4822,#4817,#250,.T.) ;
#5972=EDGE_CURVE('',#4821,#4818,#2778,.T.) ;
#5973=EDGE_CURVE('',#4823,#4823,#4085,.T.) ;
#5974=EDGE_CURVE('',#4823,#4824,#2779,.T.) ;
#5975=EDGE_CURVE('',#4824,#4751,#251,.T.) ;
#5976=EDGE_CURVE('',#4750,#4825,#252,.T.) ;
#5977=EDGE_CURVE('',#4825,#4747,#253,.T.) ;
#5978=EDGE_CURVE('',#4746,#4826,#254,.T.) ;
#5979=EDGE_CURVE('',#4826,#4743,#255,.T.) ;
#5980=EDGE_CURVE('',#4742,#4827,#256,.T.) ;
#5981=EDGE_CURVE('',#4827,#4739,#257,.T.) ;
#5982=EDGE_CURVE('',#4738,#4828,#258,.T.) ;
#5983=EDGE_CURVE('',#4828,#4735,#259,.T.) ;
#5984=EDGE_CURVE('',#4734,#4829,#260,.T.) ;
#5985=EDGE_CURVE('',#4829,#4731,#261,.T.) ;
#5986=EDGE_CURVE('',#4730,#4830,#262,.T.) ;
#5987=EDGE_CURVE('',#4830,#4727,#263,.T.) ;
#5988=EDGE_CURVE('',#4726,#4831,#264,.T.) ;
#5989=EDGE_CURVE('',#4831,#4723,#265,.T.) ;
#5990=EDGE_CURVE('',#4722,#4832,#266,.T.) ;
#5991=EDGE_CURVE('',#4832,#4719,#267,.T.) ;
#5992=EDGE_CURVE('',#4718,#4833,#268,.T.) ;
#5993=EDGE_CURVE('',#4833,#4715,#269,.T.) ;
#5994=EDGE_CURVE('',#4714,#4834,#270,.T.) ;
#5995=EDGE_CURVE('',#4834,#4711,#271,.T.) ;
#5996=EDGE_CURVE('',#4710,#4835,#272,.T.) ;
#5997=EDGE_CURVE('',#4835,#4707,#273,.T.) ;
#5998=EDGE_CURVE('',#4706,#4836,#274,.T.) ;
#5999=EDGE_CURVE('',#4836,#4703,#275,.T.) ;
#6000=EDGE_CURVE('',#4702,#4837,#276,.T.) ;
#6001=EDGE_CURVE('',#4837,#4699,#277,.T.) ;
#6002=EDGE_CURVE('',#4698,#4838,#278,.T.) ;
#6003=EDGE_CURVE('',#4838,#4695,#279,.T.) ;
#6004=EDGE_CURVE('',#4694,#4839,#280,.T.) ;
#6005=EDGE_CURVE('',#4839,#4691,#281,.T.) ;
#6006=EDGE_CURVE('',#4690,#4840,#282,.T.) ;
#6007=EDGE_CURVE('',#4840,#4687,#283,.T.) ;
#6008=EDGE_CURVE('',#4686,#4841,#284,.T.) ;
#6009=EDGE_CURVE('',#4841,#4683,#285,.T.) ;
#6010=EDGE_CURVE('',#4682,#4842,#286,.T.) ;
#6011=EDGE_CURVE('',#4842,#4679,#287,.T.) ;
#6012=EDGE_CURVE('',#4816,#4843,#288,.T.) ;
#6013=EDGE_CURVE('',#4843,#4813,#289,.T.) ;
#6014=EDGE_CURVE('',#4812,#4844,#290,.T.) ;
#6015=EDGE_CURVE('',#4844,#4809,#291,.T.) ;
#6016=EDGE_CURVE('',#4808,#4845,#292,.T.) ;
#6017=EDGE_CURVE('',#4845,#4805,#293,.T.) ;
#6018=EDGE_CURVE('',#4804,#4846,#294,.T.) ;
#6019=EDGE_CURVE('',#4846,#4801,#295,.T.) ;
#6020=EDGE_CURVE('',#4800,#4847,#296,.T.) ;
#6021=EDGE_CURVE('',#4847,#4797,#297,.T.) ;
#6022=EDGE_CURVE('',#4796,#4848,#298,.T.) ;
#6023=EDGE_CURVE('',#4848,#4793,#299,.T.) ;
#6024=EDGE_CURVE('',#4792,#4849,#300,.T.) ;
#6025=EDGE_CURVE('',#4849,#4789,#301,.T.) ;
#6026=EDGE_CURVE('',#4788,#4850,#302,.T.) ;
#6027=EDGE_CURVE('',#4850,#4785,#303,.T.) ;
#6028=EDGE_CURVE('',#4784,#4851,#304,.T.) ;
#6029=EDGE_CURVE('',#4851,#4781,#305,.T.) ;
#6030=EDGE_CURVE('',#4780,#4852,#306,.T.) ;
#6031=EDGE_CURVE('',#4852,#4777,#307,.T.) ;
#6032=EDGE_CURVE('',#4776,#4853,#308,.T.) ;
#6033=EDGE_CURVE('',#4853,#4773,#309,.T.) ;
#6034=EDGE_CURVE('',#4772,#4854,#310,.T.) ;
#6035=EDGE_CURVE('',#4854,#4769,#311,.T.) ;
#6036=EDGE_CURVE('',#4768,#4855,#312,.T.) ;
#6037=EDGE_CURVE('',#4855,#4765,#313,.T.) ;
#6038=EDGE_CURVE('',#4764,#4856,#314,.T.) ;
#6039=EDGE_CURVE('',#4856,#4761,#315,.T.) ;
#6040=EDGE_CURVE('',#4760,#4857,#316,.T.) ;
#6041=EDGE_CURVE('',#4857,#4757,#317,.T.) ;
#6042=EDGE_CURVE('',#4756,#4824,#318,.T.) ;
#6043=EDGE_CURVE('',#4858,#4814,#2780,.T.) ;
#6044=EDGE_CURVE('',#4815,#4858,#2781,.T.) ;
#6045=EDGE_CURVE('',#4843,#4858,#2782,.T.) ;
#6046=EDGE_CURVE('',#4811,#4859,#2783,.T.) ;
#6047=EDGE_CURVE('',#4844,#4859,#2784,.T.) ;
#6048=EDGE_CURVE('',#4859,#4810,#2785,.T.) ;
#6049=EDGE_CURVE('',#4860,#4806,#2786,.T.) ;
#6050=EDGE_CURVE('',#4807,#4860,#2787,.T.) ;
#6051=EDGE_CURVE('',#4845,#4860,#2788,.T.) ;
#6052=EDGE_CURVE('',#4803,#4861,#2789,.T.) ;
#6053=EDGE_CURVE('',#4846,#4861,#2790,.T.) ;
#6054=EDGE_CURVE('',#4861,#4802,#2791,.T.) ;
#6055=EDGE_CURVE('',#4862,#4798,#2792,.T.) ;
#6056=EDGE_CURVE('',#4799,#4862,#2793,.T.) ;
#6057=EDGE_CURVE('',#4847,#4862,#2794,.T.) ;
#6058=EDGE_CURVE('',#4795,#4863,#2795,.T.) ;
#6059=EDGE_CURVE('',#4848,#4863,#2796,.T.) ;
#6060=EDGE_CURVE('',#4863,#4794,#2797,.T.) ;
#6061=EDGE_CURVE('',#4864,#4790,#2798,.T.) ;
#6062=EDGE_CURVE('',#4791,#4864,#2799,.T.) ;
#6063=EDGE_CURVE('',#4849,#4864,#2800,.T.) ;
#6064=EDGE_CURVE('',#4787,#4865,#2801,.T.) ;
#6065=EDGE_CURVE('',#4850,#4865,#2802,.T.) ;
#6066=EDGE_CURVE('',#4865,#4786,#2803,.T.) ;
#6067=EDGE_CURVE('',#4866,#4782,#2804,.T.) ;
#6068=EDGE_CURVE('',#4783,#4866,#2805,.T.) ;
#6069=EDGE_CURVE('',#4851,#4866,#2806,.T.) ;
#6070=EDGE_CURVE('',#4779,#4867,#2807,.T.) ;
#6071=EDGE_CURVE('',#4852,#4867,#2808,.T.) ;
#6072=EDGE_CURVE('',#4867,#4778,#2809,.T.) ;
#6073=EDGE_CURVE('',#4868,#4774,#2810,.T.) ;
#6074=EDGE_CURVE('',#4775,#4868,#2811,.T.) ;
#6075=EDGE_CURVE('',#4853,#4868,#2812,.T.) ;
#6076=EDGE_CURVE('',#4771,#4869,#2813,.T.) ;
#6077=EDGE_CURVE('',#4854,#4869,#2814,.T.) ;
#6078=EDGE_CURVE('',#4869,#4770,#2815,.T.) ;
#6079=EDGE_CURVE('',#4870,#4766,#2816,.T.) ;
#6080=EDGE_CURVE('',#4767,#4870,#2817,.T.) ;
#6081=EDGE_CURVE('',#4855,#4870,#2818,.T.) ;
#6082=EDGE_CURVE('',#4763,#4871,#2819,.T.) ;
#6083=EDGE_CURVE('',#4856,#4871,#2820,.T.) ;
#6084=EDGE_CURVE('',#4871,#4762,#2821,.T.) ;
#6085=EDGE_CURVE('',#4872,#4758,#2822,.T.) ;
#6086=EDGE_CURVE('',#4759,#4872,#2823,.T.) ;
#6087=EDGE_CURVE('',#4857,#4872,#2824,.T.) ;
#6088=EDGE_CURVE('',#4755,#4873,#2825,.T.) ;
#6089=EDGE_CURVE('',#4824,#4873,#2826,.T.) ;
#6090=EDGE_CURVE('',#4873,#4752,#2827,.T.) ;
#6091=EDGE_CURVE('',#4874,#4748,#2828,.T.) ;
#6092=EDGE_CURVE('',#4749,#4874,#2829,.T.) ;
#6093=EDGE_CURVE('',#4825,#4874,#2830,.T.) ;
#6094=EDGE_CURVE('',#4745,#4875,#2831,.T.) ;
#6095=EDGE_CURVE('',#4826,#4875,#2832,.T.) ;
#6096=EDGE_CURVE('',#4875,#4744,#2833,.T.) ;
#6097=EDGE_CURVE('',#4876,#4740,#2834,.T.) ;
#6098=EDGE_CURVE('',#4741,#4876,#2835,.T.) ;
#6099=EDGE_CURVE('',#4827,#4876,#2836,.T.) ;
#6100=EDGE_CURVE('',#4737,#4877,#2837,.T.) ;
#6101=EDGE_CURVE('',#4828,#4877,#2838,.T.) ;
#6102=EDGE_CURVE('',#4877,#4736,#2839,.T.) ;
#6103=EDGE_CURVE('',#4878,#4732,#2840,.T.) ;
#6104=EDGE_CURVE('',#4733,#4878,#2841,.T.) ;
#6105=EDGE_CURVE('',#4829,#4878,#2842,.T.) ;
#6106=EDGE_CURVE('',#4729,#4879,#2843,.T.) ;
#6107=EDGE_CURVE('',#4830,#4879,#2844,.T.) ;
#6108=EDGE_CURVE('',#4879,#4728,#2845,.T.) ;
#6109=EDGE_CURVE('',#4880,#4724,#2846,.T.) ;
#6110=EDGE_CURVE('',#4725,#4880,#2847,.T.) ;
#6111=EDGE_CURVE('',#4831,#4880,#2848,.T.) ;
#6112=EDGE_CURVE('',#4721,#4881,#2849,.T.) ;
#6113=EDGE_CURVE('',#4832,#4881,#2850,.T.) ;
#6114=EDGE_CURVE('',#4881,#4720,#2851,.T.) ;
#6115=EDGE_CURVE('',#4882,#4716,#2852,.T.) ;
#6116=EDGE_CURVE('',#4717,#4882,#2853,.T.) ;
#6117=EDGE_CURVE('',#4833,#4882,#2854,.T.) ;
#6118=EDGE_CURVE('',#4713,#4883,#2855,.T.) ;
#6119=EDGE_CURVE('',#4834,#4883,#2856,.T.) ;
#6120=EDGE_CURVE('',#4883,#4712,#2857,.T.) ;
#6121=EDGE_CURVE('',#4884,#4708,#2858,.T.) ;
#6122=EDGE_CURVE('',#4709,#4884,#2859,.T.) ;
#6123=EDGE_CURVE('',#4835,#4884,#2860,.T.) ;
#6124=EDGE_CURVE('',#4705,#4885,#2861,.T.) ;
#6125=EDGE_CURVE('',#4836,#4885,#2862,.T.) ;
#6126=EDGE_CURVE('',#4885,#4704,#2863,.T.) ;
#6127=EDGE_CURVE('',#4886,#4700,#2864,.T.) ;
#6128=EDGE_CURVE('',#4701,#4886,#2865,.T.) ;
#6129=EDGE_CURVE('',#4837,#4886,#2866,.T.) ;
#6130=EDGE_CURVE('',#4697,#4887,#2867,.T.) ;
#6131=EDGE_CURVE('',#4838,#4887,#2868,.T.) ;
#6132=EDGE_CURVE('',#4887,#4696,#2869,.T.) ;
#6133=EDGE_CURVE('',#4888,#4692,#2870,.T.) ;
#6134=EDGE_CURVE('',#4693,#4888,#2871,.T.) ;
#6135=EDGE_CURVE('',#4839,#4888,#2872,.T.) ;
#6136=EDGE_CURVE('',#4689,#4889,#2873,.T.) ;
#6137=EDGE_CURVE('',#4840,#4889,#2874,.T.) ;
#6138=EDGE_CURVE('',#4889,#4688,#2875,.T.) ;
#6139=EDGE_CURVE('',#4890,#4684,#2876,.T.) ;
#6140=EDGE_CURVE('',#4685,#4890,#2877,.T.) ;
#6141=EDGE_CURVE('',#4841,#4890,#2878,.T.) ;
#6142=EDGE_CURVE('',#4681,#4891,#2879,.T.) ;
#6143=EDGE_CURVE('',#4842,#4891,#2880,.T.) ;
#6144=EDGE_CURVE('',#4891,#4680,#2881,.T.) ;
#6145=EDGE_CURVE('',#4671,#4754,#4086,.T.) ;
#6146=EDGE_CURVE('',#4892,#4892,#4087,.T.) ;
#6147=EDGE_CURVE('',#4892,#4893,#2882,.T.) ;
#6148=EDGE_CURVE('',#4894,#4893,#319,.T.) ;
#6149=EDGE_CURVE('',#4894,#4895,#4088,.T.) ;
#6150=EDGE_CURVE('',#4896,#4895,#320,.T.) ;
#6151=EDGE_CURVE('',#4897,#4896,#321,.T.) ;
#6152=EDGE_CURVE('',#4897,#4898,#4089,.T.) ;
#6153=EDGE_CURVE('',#4899,#4898,#322,.T.) ;
#6154=EDGE_CURVE('',#4900,#4899,#323,.T.) ;
#6155=EDGE_CURVE('',#4900,#4901,#4090,.T.) ;
#6156=EDGE_CURVE('',#4902,#4901,#324,.T.) ;
#6157=EDGE_CURVE('',#4903,#4902,#325,.T.) ;
#6158=EDGE_CURVE('',#4903,#4904,#4091,.T.) ;
#6159=EDGE_CURVE('',#4905,#4904,#326,.T.) ;
#6160=EDGE_CURVE('',#4906,#4905,#327,.T.) ;
#6161=EDGE_CURVE('',#4906,#4907,#4092,.T.) ;
#6162=EDGE_CURVE('',#4908,#4907,#328,.T.) ;
#6163=EDGE_CURVE('',#4909,#4908,#329,.T.) ;
#6164=EDGE_CURVE('',#4909,#4910,#4093,.T.) ;
#6165=EDGE_CURVE('',#4893,#4910,#330,.T.) ;
#6166=EDGE_CURVE('',#4901,#4911,#2883,.T.) ;
#6167=EDGE_CURVE('',#4912,#4900,#2884,.T.) ;
#6168=EDGE_CURVE('',#4911,#4912,#4094,.T.) ;
#6169=EDGE_CURVE('',#4904,#4913,#2885,.T.) ;
#6170=EDGE_CURVE('',#4914,#4903,#2886,.T.) ;
#6171=EDGE_CURVE('',#4913,#4914,#4095,.T.) ;
#6172=EDGE_CURVE('',#4915,#4897,#2887,.T.) ;
#6173=EDGE_CURVE('',#4916,#4915,#4096,.T.) ;
#6174=EDGE_CURVE('',#4898,#4916,#2888,.T.) ;
#6175=EDGE_CURVE('',#4907,#4917,#2889,.T.) ;
#6176=EDGE_CURVE('',#4918,#4906,#2890,.T.) ;
#6177=EDGE_CURVE('',#4917,#4918,#4097,.T.) ;
#6178=EDGE_CURVE('',#4919,#4894,#2891,.T.) ;
#6179=EDGE_CURVE('',#4920,#4919,#4098,.T.) ;
#6180=EDGE_CURVE('',#4895,#4920,#2892,.T.) ;
#6181=EDGE_CURVE('',#4921,#4909,#2893,.T.) ;
#6182=EDGE_CURVE('',#4922,#4921,#4099,.T.) ;
#6183=EDGE_CURVE('',#4910,#4922,#2894,.T.) ;
#6184=EDGE_CURVE('',#4918,#4917,#2895,.T.) ;
#6185=EDGE_CURVE('',#4905,#4923,#2896,.T.) ;
#6186=EDGE_CURVE('',#4923,#4924,#2897,.T.) ;
#6187=EDGE_CURVE('',#4908,#4924,#2898,.T.) ;
#6188=EDGE_CURVE('',#4914,#4913,#2899,.T.) ;
#6189=EDGE_CURVE('',#4902,#4925,#2900,.T.) ;
#6190=EDGE_CURVE('',#4925,#4923,#2901,.T.) ;
#6191=EDGE_CURVE('',#4912,#4911,#2902,.T.) ;
#6192=EDGE_CURVE('',#4899,#4926,#2903,.T.) ;
#6193=EDGE_CURVE('',#4926,#4925,#2904,.T.) ;
#6194=EDGE_CURVE('',#4915,#4916,#2905,.T.) ;
#6195=EDGE_CURVE('',#4919,#4920,#2906,.T.) ;
#6196=EDGE_CURVE('',#4921,#4922,#2907,.T.) ;
#6197=EDGE_CURVE('',#4927,#4926,#2908,.T.) ;
#6198=EDGE_CURVE('',#4927,#4926,#4100,.T.) ;
#6199=EDGE_CURVE('',#4926,#4925,#4101,.T.) ;
#6200=EDGE_CURVE('',#4925,#4923,#4102,.T.) ;
#6201=EDGE_CURVE('',#4923,#4924,#4103,.T.) ;
#6202=EDGE_CURVE('',#4924,#4928,#2909,.T.) ;
#6203=EDGE_CURVE('',#4924,#4928,#4104,.T.) ;
#6204=EDGE_CURVE('',#4928,#4927,#2910,.T.) ;
#6205=EDGE_CURVE('',#4928,#4927,#4105,.T.) ;
#6206=EDGE_CURVE('',#4928,#4929,#2911,.T.) ;
#6207=EDGE_CURVE('',#4896,#4927,#2912,.T.) ;
#6208=EDGE_CURVE('',#4893,#4928,#2913,.T.) ;
#7729=ORIENTED_EDGE('',*,*,#5711,.F.) ;
#7730=ORIENTED_EDGE('',*,*,#5712,.T.) ;
#7731=ORIENTED_EDGE('',*,*,#5713,.F.) ;
#7732=ORIENTED_EDGE('',*,*,#5714,.T.) ;
#7733=ORIENTED_EDGE('',*,*,#5715,.F.) ;
#7734=ORIENTED_EDGE('',*,*,#5716,.T.) ;
#7735=ORIENTED_EDGE('',*,*,#5711,.T.) ;
#7736=ORIENTED_EDGE('',*,*,#5717,.T.) ;
#7737=ORIENTED_EDGE('',*,*,#5718,.F.) ;
#7738=ORIENTED_EDGE('',*,*,#5719,.T.) ;
#7739=ORIENTED_EDGE('',*,*,#5715,.T.) ;
#7740=ORIENTED_EDGE('',*,*,#5720,.T.) ;
#7741=ORIENTED_EDGE('',*,*,#5721,.F.) ;
#7742=ORIENTED_EDGE('',*,*,#5722,.T.) ;
#7743=ORIENTED_EDGE('',*,*,#5718,.T.) ;
#7744=ORIENTED_EDGE('',*,*,#5723,.T.) ;
#7745=ORIENTED_EDGE('',*,*,#5724,.F.) ;
#7746=ORIENTED_EDGE('',*,*,#5725,.T.) ;
#7747=ORIENTED_EDGE('',*,*,#5721,.T.) ;
#7748=ORIENTED_EDGE('',*,*,#5726,.T.) ;
#7749=ORIENTED_EDGE('',*,*,#5727,.F.) ;
#7750=ORIENTED_EDGE('',*,*,#5728,.T.) ;
#7751=ORIENTED_EDGE('',*,*,#5724,.T.) ;
#7752=ORIENTED_EDGE('',*,*,#5729,.T.) ;
#7753=ORIENTED_EDGE('',*,*,#5730,.F.) ;
#7754=ORIENTED_EDGE('',*,*,#5731,.T.) ;
#7755=ORIENTED_EDGE('',*,*,#5727,.T.) ;
#7756=ORIENTED_EDGE('',*,*,#5732,.T.) ;
#7757=ORIENTED_EDGE('',*,*,#5733,.F.) ;
#7758=ORIENTED_EDGE('',*,*,#5734,.T.) ;
#7759=ORIENTED_EDGE('',*,*,#5730,.T.) ;
#7760=ORIENTED_EDGE('',*,*,#5735,.T.) ;
#7761=ORIENTED_EDGE('',*,*,#5736,.F.) ;
#7762=ORIENTED_EDGE('',*,*,#5737,.T.) ;
#7763=ORIENTED_EDGE('',*,*,#5733,.T.) ;
#7764=ORIENTED_EDGE('',*,*,#5738,.T.) ;
#7765=ORIENTED_EDGE('',*,*,#5739,.F.) ;
#7766=ORIENTED_EDGE('',*,*,#5740,.T.) ;
#7767=ORIENTED_EDGE('',*,*,#5736,.T.) ;
#7768=ORIENTED_EDGE('',*,*,#5741,.T.) ;
#7769=ORIENTED_EDGE('',*,*,#5742,.F.) ;
#7770=ORIENTED_EDGE('',*,*,#5743,.T.) ;
#7771=ORIENTED_EDGE('',*,*,#5739,.T.) ;
#7772=ORIENTED_EDGE('',*,*,#5744,.T.) ;
#7773=ORIENTED_EDGE('',*,*,#5745,.F.) ;
#7774=ORIENTED_EDGE('',*,*,#5746,.T.) ;
#7775=ORIENTED_EDGE('',*,*,#5742,.T.) ;
#7776=ORIENTED_EDGE('',*,*,#5747,.T.) ;
#7777=ORIENTED_EDGE('',*,*,#5748,.F.) ;
#7778=ORIENTED_EDGE('',*,*,#5749,.T.) ;
#7779=ORIENTED_EDGE('',*,*,#5745,.T.) ;
#7780=ORIENTED_EDGE('',*,*,#5750,.T.) ;
#7781=ORIENTED_EDGE('',*,*,#5751,.F.) ;
#7782=ORIENTED_EDGE('',*,*,#5752,.T.) ;
#7783=ORIENTED_EDGE('',*,*,#5748,.T.) ;
#7784=ORIENTED_EDGE('',*,*,#5753,.T.) ;
#7785=ORIENTED_EDGE('',*,*,#5754,.F.) ;
#7786=ORIENTED_EDGE('',*,*,#5755,.T.) ;
#7787=ORIENTED_EDGE('',*,*,#5756,.F.) ;
#7788=ORIENTED_EDGE('',*,*,#5757,.F.) ;
#7789=ORIENTED_EDGE('',*,*,#5758,.F.) ;
#7790=ORIENTED_EDGE('',*,*,#5759,.T.) ;
#7791=ORIENTED_EDGE('',*,*,#5754,.T.) ;
#7792=ORIENTED_EDGE('',*,*,#5760,.F.) ;
#7793=ORIENTED_EDGE('',*,*,#5761,.F.) ;
#7794=ORIENTED_EDGE('',*,*,#5762,.T.) ;
#7795=ORIENTED_EDGE('',*,*,#5758,.T.) ;
#7796=ORIENTED_EDGE('',*,*,#5763,.F.) ;
#7797=ORIENTED_EDGE('',*,*,#5764,.F.) ;
#7798=ORIENTED_EDGE('',*,*,#5765,.T.) ;
#7799=ORIENTED_EDGE('',*,*,#5761,.T.) ;
#7800=ORIENTED_EDGE('',*,*,#5766,.F.) ;
#7801=ORIENTED_EDGE('',*,*,#5767,.F.) ;
#7802=ORIENTED_EDGE('',*,*,#5768,.T.) ;
#7803=ORIENTED_EDGE('',*,*,#5764,.T.) ;
#7804=ORIENTED_EDGE('',*,*,#5769,.F.) ;
#7805=ORIENTED_EDGE('',*,*,#5770,.F.) ;
#7806=ORIENTED_EDGE('',*,*,#5771,.T.) ;
#7807=ORIENTED_EDGE('',*,*,#5767,.T.) ;
#7808=ORIENTED_EDGE('',*,*,#5772,.F.) ;
#7809=ORIENTED_EDGE('',*,*,#5773,.F.) ;
#7810=ORIENTED_EDGE('',*,*,#5774,.T.) ;
#7811=ORIENTED_EDGE('',*,*,#5770,.T.) ;
#7812=ORIENTED_EDGE('',*,*,#5775,.F.) ;
#7813=ORIENTED_EDGE('',*,*,#5776,.F.) ;
#7814=ORIENTED_EDGE('',*,*,#5777,.T.) ;
#7815=ORIENTED_EDGE('',*,*,#5773,.T.) ;
#7816=ORIENTED_EDGE('',*,*,#5778,.F.) ;
#7817=ORIENTED_EDGE('',*,*,#5779,.F.) ;
#7818=ORIENTED_EDGE('',*,*,#5780,.T.) ;
#7819=ORIENTED_EDGE('',*,*,#5776,.T.) ;
#7820=ORIENTED_EDGE('',*,*,#5781,.F.) ;
#7821=ORIENTED_EDGE('',*,*,#5782,.F.) ;
#7822=ORIENTED_EDGE('',*,*,#5783,.T.) ;
#7823=ORIENTED_EDGE('',*,*,#5779,.T.) ;
#7824=ORIENTED_EDGE('',*,*,#5784,.F.) ;
#7825=ORIENTED_EDGE('',*,*,#5785,.F.) ;
#7826=ORIENTED_EDGE('',*,*,#5786,.T.) ;
#7827=ORIENTED_EDGE('',*,*,#5782,.T.) ;
#7828=ORIENTED_EDGE('',*,*,#5787,.F.) ;
#7829=ORIENTED_EDGE('',*,*,#5788,.F.) ;
#7830=ORIENTED_EDGE('',*,*,#5789,.T.) ;
#7831=ORIENTED_EDGE('',*,*,#5785,.T.) ;
#7832=ORIENTED_EDGE('',*,*,#5790,.F.) ;
#7833=ORIENTED_EDGE('',*,*,#5791,.F.) ;
#7834=ORIENTED_EDGE('',*,*,#5792,.T.) ;
#7835=ORIENTED_EDGE('',*,*,#5788,.T.) ;
#7836=ORIENTED_EDGE('',*,*,#5793,.F.) ;
#7837=ORIENTED_EDGE('',*,*,#5794,.F.) ;
#7838=ORIENTED_EDGE('',*,*,#5795,.T.) ;
#7839=ORIENTED_EDGE('',*,*,#5791,.T.) ;
#7840=ORIENTED_EDGE('',*,*,#5796,.F.) ;
#7841=ORIENTED_EDGE('',*,*,#5756,.T.) ;
#7842=ORIENTED_EDGE('',*,*,#5797,.T.) ;
#7843=ORIENTED_EDGE('',*,*,#5798,.F.) ;
#7844=ORIENTED_EDGE('',*,*,#5799,.F.) ;
#7845=ORIENTED_EDGE('',*,*,#5800,.T.) ;
#7846=ORIENTED_EDGE('',*,*,#5800,.F.) ;
#7847=ORIENTED_EDGE('',*,*,#5801,.F.) ;
#7848=ORIENTED_EDGE('',*,*,#5753,.F.) ;
#7849=ORIENTED_EDGE('',*,*,#5750,.F.) ;
#7850=ORIENTED_EDGE('',*,*,#5747,.F.) ;
#7851=ORIENTED_EDGE('',*,*,#5744,.F.) ;
#7852=ORIENTED_EDGE('',*,*,#5741,.F.) ;
#7853=ORIENTED_EDGE('',*,*,#5738,.F.) ;
#7854=ORIENTED_EDGE('',*,*,#5735,.F.) ;
#7855=ORIENTED_EDGE('',*,*,#5732,.F.) ;
#7856=ORIENTED_EDGE('',*,*,#5729,.F.) ;
#7857=ORIENTED_EDGE('',*,*,#5726,.F.) ;
#7858=ORIENTED_EDGE('',*,*,#5723,.F.) ;
#7859=ORIENTED_EDGE('',*,*,#5720,.F.) ;
#7860=ORIENTED_EDGE('',*,*,#5717,.F.) ;
#7861=ORIENTED_EDGE('',*,*,#5714,.F.) ;
#7862=ORIENTED_EDGE('',*,*,#5802,.F.) ;
#7863=ORIENTED_EDGE('',*,*,#5803,.T.) ;
#7864=ORIENTED_EDGE('',*,*,#5796,.T.) ;
#7865=ORIENTED_EDGE('',*,*,#5793,.T.) ;
#7866=ORIENTED_EDGE('',*,*,#5790,.T.) ;
#7867=ORIENTED_EDGE('',*,*,#5787,.T.) ;
#7868=ORIENTED_EDGE('',*,*,#5784,.T.) ;
#7869=ORIENTED_EDGE('',*,*,#5781,.T.) ;
#7870=ORIENTED_EDGE('',*,*,#5778,.T.) ;
#7871=ORIENTED_EDGE('',*,*,#5775,.T.) ;
#7872=ORIENTED_EDGE('',*,*,#5772,.T.) ;
#7873=ORIENTED_EDGE('',*,*,#5769,.T.) ;
#7874=ORIENTED_EDGE('',*,*,#5766,.T.) ;
#7875=ORIENTED_EDGE('',*,*,#5763,.T.) ;
#7876=ORIENTED_EDGE('',*,*,#5760,.T.) ;
#7877=ORIENTED_EDGE('',*,*,#5757,.T.) ;
#7878=ORIENTED_EDGE('',*,*,#5804,.F.) ;
#7879=ORIENTED_EDGE('',*,*,#5805,.T.) ;
#7880=ORIENTED_EDGE('',*,*,#5806,.T.) ;
#7881=ORIENTED_EDGE('',*,*,#5802,.T.) ;
#7882=ORIENTED_EDGE('',*,*,#5807,.F.) ;
#7883=ORIENTED_EDGE('',*,*,#5794,.T.) ;
#7884=ORIENTED_EDGE('',*,*,#5803,.F.) ;
#7885=ORIENTED_EDGE('',*,*,#5806,.F.) ;
#7886=ORIENTED_EDGE('',*,*,#5808,.T.) ;
#7887=ORIENTED_EDGE('',*,*,#5797,.F.) ;
#7888=ORIENTED_EDGE('',*,*,#5755,.F.) ;
#7889=ORIENTED_EDGE('',*,*,#5759,.F.) ;
#7890=ORIENTED_EDGE('',*,*,#5762,.F.) ;
#7891=ORIENTED_EDGE('',*,*,#5765,.F.) ;
#7892=ORIENTED_EDGE('',*,*,#5768,.F.) ;
#7893=ORIENTED_EDGE('',*,*,#5771,.F.) ;
#7894=ORIENTED_EDGE('',*,*,#5774,.F.) ;
#7895=ORIENTED_EDGE('',*,*,#5777,.F.) ;
#7896=ORIENTED_EDGE('',*,*,#5780,.F.) ;
#7897=ORIENTED_EDGE('',*,*,#5783,.F.) ;
#7898=ORIENTED_EDGE('',*,*,#5786,.F.) ;
#7899=ORIENTED_EDGE('',*,*,#5789,.F.) ;
#7900=ORIENTED_EDGE('',*,*,#5792,.F.) ;
#7901=ORIENTED_EDGE('',*,*,#5795,.F.) ;
#7902=ORIENTED_EDGE('',*,*,#5808,.F.) ;
#7903=ORIENTED_EDGE('',*,*,#5805,.F.) ;
#7904=ORIENTED_EDGE('',*,*,#5712,.F.) ;
#7905=ORIENTED_EDGE('',*,*,#5716,.F.) ;
#7906=ORIENTED_EDGE('',*,*,#5719,.F.) ;
#7907=ORIENTED_EDGE('',*,*,#5722,.F.) ;
#7908=ORIENTED_EDGE('',*,*,#5725,.F.) ;
#7909=ORIENTED_EDGE('',*,*,#5728,.F.) ;
#7910=ORIENTED_EDGE('',*,*,#5731,.F.) ;
#7911=ORIENTED_EDGE('',*,*,#5734,.F.) ;
#7912=ORIENTED_EDGE('',*,*,#5737,.F.) ;
#7913=ORIENTED_EDGE('',*,*,#5740,.F.) ;
#7914=ORIENTED_EDGE('',*,*,#5743,.F.) ;
#7915=ORIENTED_EDGE('',*,*,#5746,.F.) ;
#7916=ORIENTED_EDGE('',*,*,#5749,.F.) ;
#7917=ORIENTED_EDGE('',*,*,#5752,.F.) ;
#7918=ORIENTED_EDGE('',*,*,#5809,.F.) ;
#7919=ORIENTED_EDGE('',*,*,#5804,.T.) ;
#7920=ORIENTED_EDGE('',*,*,#5810,.T.) ;
#7921=ORIENTED_EDGE('',*,*,#5811,.T.) ;
#7922=ORIENTED_EDGE('',*,*,#5810,.F.) ;
#7923=ORIENTED_EDGE('',*,*,#5807,.T.) ;
#7924=ORIENTED_EDGE('',*,*,#5713,.T.) ;
#7925=ORIENTED_EDGE('',*,*,#5751,.T.) ;
#7926=ORIENTED_EDGE('',*,*,#5801,.T.) ;
#7927=ORIENTED_EDGE('',*,*,#5812,.F.) ;
#7928=ORIENTED_EDGE('',*,*,#5809,.T.) ;
#7929=ORIENTED_EDGE('',*,*,#5813,.F.) ;
#7930=ORIENTED_EDGE('',*,*,#5811,.F.) ;
#7931=ORIENTED_EDGE('',*,*,#5799,.T.) ;
#7932=ORIENTED_EDGE('',*,*,#5814,.T.) ;
#7933=ORIENTED_EDGE('',*,*,#5815,.T.) ;
#7934=ORIENTED_EDGE('',*,*,#5814,.F.) ;
#7935=ORIENTED_EDGE('',*,*,#5798,.T.) ;
#7936=ORIENTED_EDGE('',*,*,#5812,.T.) ;
#7937=ORIENTED_EDGE('',*,*,#5815,.F.) ;
#7938=ORIENTED_EDGE('',*,*,#5816,.F.) ;
#7939=ORIENTED_EDGE('',*,*,#5817,.F.) ;
#7940=ORIENTED_EDGE('',*,*,#5818,.F.) ;
#7941=ORIENTED_EDGE('',*,*,#5819,.F.) ;
#7942=ORIENTED_EDGE('',*,*,#5818,.T.) ;
#7943=ORIENTED_EDGE('',*,*,#5820,.F.) ;
#7944=ORIENTED_EDGE('',*,*,#5821,.F.) ;
#7945=ORIENTED_EDGE('',*,*,#5822,.F.) ;
#7946=ORIENTED_EDGE('',*,*,#5823,.F.) ;
#7947=ORIENTED_EDGE('',*,*,#5820,.T.) ;
#7948=ORIENTED_EDGE('',*,*,#5817,.T.) ;
#7949=ORIENTED_EDGE('',*,*,#5822,.T.) ;
#7950=ORIENTED_EDGE('',*,*,#5816,.T.) ;
#7951=ORIENTED_EDGE('',*,*,#5819,.T.) ;
#7952=ORIENTED_EDGE('',*,*,#5824,.F.) ;
#7953=ORIENTED_EDGE('',*,*,#5825,.T.) ;
#7954=ORIENTED_EDGE('',*,*,#5826,.T.) ;
#7955=ORIENTED_EDGE('',*,*,#5827,.T.) ;
#7956=ORIENTED_EDGE('',*,*,#5828,.F.) ;
#7957=ORIENTED_EDGE('',*,*,#5829,.T.) ;
#7958=ORIENTED_EDGE('',*,*,#5830,.T.) ;
#7959=ORIENTED_EDGE('',*,*,#5831,.T.) ;
#7960=ORIENTED_EDGE('',*,*,#5832,.F.) ;
#7961=ORIENTED_EDGE('',*,*,#5833,.T.) ;
#7962=ORIENTED_EDGE('',*,*,#5834,.T.) ;
#7963=ORIENTED_EDGE('',*,*,#5835,.T.) ;
#7964=ORIENTED_EDGE('',*,*,#5836,.F.) ;
#7965=ORIENTED_EDGE('',*,*,#5837,.T.) ;
#7966=ORIENTED_EDGE('',*,*,#5838,.T.) ;
#7967=ORIENTED_EDGE('',*,*,#5839,.T.) ;
#7968=ORIENTED_EDGE('',*,*,#5840,.F.) ;
#7969=ORIENTED_EDGE('',*,*,#5841,.T.) ;
#7970=ORIENTED_EDGE('',*,*,#5842,.T.) ;
#7971=ORIENTED_EDGE('',*,*,#5843,.T.) ;
#7972=ORIENTED_EDGE('',*,*,#5844,.F.) ;
#7973=ORIENTED_EDGE('',*,*,#5845,.T.) ;
#7974=ORIENTED_EDGE('',*,*,#5846,.T.) ;
#7975=ORIENTED_EDGE('',*,*,#5847,.T.) ;
#7976=ORIENTED_EDGE('',*,*,#5848,.F.) ;
#7977=ORIENTED_EDGE('',*,*,#5849,.T.) ;
#7978=ORIENTED_EDGE('',*,*,#5850,.T.) ;
#7979=ORIENTED_EDGE('',*,*,#5851,.T.) ;
#7980=ORIENTED_EDGE('',*,*,#5852,.F.) ;
#7981=ORIENTED_EDGE('',*,*,#5853,.T.) ;
#7982=ORIENTED_EDGE('',*,*,#5854,.T.) ;
#7983=ORIENTED_EDGE('',*,*,#5855,.T.) ;
#7984=ORIENTED_EDGE('',*,*,#5856,.F.) ;
#7985=ORIENTED_EDGE('',*,*,#5857,.T.) ;
#7986=ORIENTED_EDGE('',*,*,#5858,.T.) ;
#7987=ORIENTED_EDGE('',*,*,#5859,.T.) ;
#7988=ORIENTED_EDGE('',*,*,#5860,.F.) ;
#7989=ORIENTED_EDGE('',*,*,#5861,.T.) ;
#7990=ORIENTED_EDGE('',*,*,#5862,.T.) ;
#7991=ORIENTED_EDGE('',*,*,#5863,.T.) ;
#7992=ORIENTED_EDGE('',*,*,#5864,.F.) ;
#7993=ORIENTED_EDGE('',*,*,#5865,.T.) ;
#7994=ORIENTED_EDGE('',*,*,#5866,.T.) ;
#7995=ORIENTED_EDGE('',*,*,#5867,.T.) ;
#7996=ORIENTED_EDGE('',*,*,#5868,.F.) ;
#7997=ORIENTED_EDGE('',*,*,#5869,.T.) ;
#7998=ORIENTED_EDGE('',*,*,#5870,.T.) ;
#7999=ORIENTED_EDGE('',*,*,#5871,.T.) ;
#8000=ORIENTED_EDGE('',*,*,#5872,.F.) ;
#8001=ORIENTED_EDGE('',*,*,#5873,.T.) ;
#8002=ORIENTED_EDGE('',*,*,#5874,.T.) ;
#8003=ORIENTED_EDGE('',*,*,#5875,.T.) ;
#8004=ORIENTED_EDGE('',*,*,#5876,.F.) ;
#8005=ORIENTED_EDGE('',*,*,#5877,.T.) ;
#8006=ORIENTED_EDGE('',*,*,#5878,.T.) ;
#8007=ORIENTED_EDGE('',*,*,#5879,.T.) ;
#8008=ORIENTED_EDGE('',*,*,#5880,.F.) ;
#8009=ORIENTED_EDGE('',*,*,#5881,.T.) ;
#8010=ORIENTED_EDGE('',*,*,#5882,.T.) ;
#8011=ORIENTED_EDGE('',*,*,#5883,.T.) ;
#8012=ORIENTED_EDGE('',*,*,#5884,.F.) ;
#8013=ORIENTED_EDGE('',*,*,#5885,.T.) ;
#8014=ORIENTED_EDGE('',*,*,#5886,.T.) ;
#8015=ORIENTED_EDGE('',*,*,#5887,.T.) ;
#8016=ORIENTED_EDGE('',*,*,#5888,.F.) ;
#8017=ORIENTED_EDGE('',*,*,#5889,.T.) ;
#8018=ORIENTED_EDGE('',*,*,#5890,.T.) ;
#8019=ORIENTED_EDGE('',*,*,#5891,.T.) ;
#8020=ORIENTED_EDGE('',*,*,#5892,.F.) ;
#8021=ORIENTED_EDGE('',*,*,#5893,.T.) ;
#8022=ORIENTED_EDGE('',*,*,#5894,.T.) ;
#8023=ORIENTED_EDGE('',*,*,#5895,.T.) ;
#8024=ORIENTED_EDGE('',*,*,#5896,.F.) ;
#8025=ORIENTED_EDGE('',*,*,#5897,.T.) ;
#8026=ORIENTED_EDGE('',*,*,#5898,.T.) ;
#8027=ORIENTED_EDGE('',*,*,#5899,.T.) ;
#8028=ORIENTED_EDGE('',*,*,#5900,.F.) ;
#8029=ORIENTED_EDGE('',*,*,#5899,.F.) ;
#8030=ORIENTED_EDGE('',*,*,#5901,.T.) ;
#8031=ORIENTED_EDGE('',*,*,#5902,.T.) ;
#8032=ORIENTED_EDGE('',*,*,#5903,.F.) ;
#8033=ORIENTED_EDGE('',*,*,#5904,.T.) ;
#8034=ORIENTED_EDGE('',*,*,#5905,.T.) ;
#8035=ORIENTED_EDGE('',*,*,#5906,.T.) ;
#8036=ORIENTED_EDGE('',*,*,#5907,.F.) ;
#8037=ORIENTED_EDGE('',*,*,#5908,.T.) ;
#8038=ORIENTED_EDGE('',*,*,#5909,.T.) ;
#8039=ORIENTED_EDGE('',*,*,#5910,.T.) ;
#8040=ORIENTED_EDGE('',*,*,#5911,.F.) ;
#8041=ORIENTED_EDGE('',*,*,#5912,.T.) ;
#8042=ORIENTED_EDGE('',*,*,#5913,.T.) ;
#8043=ORIENTED_EDGE('',*,*,#5914,.T.) ;
#8044=ORIENTED_EDGE('',*,*,#5915,.F.) ;
#8045=ORIENTED_EDGE('',*,*,#5916,.T.) ;
#8046=ORIENTED_EDGE('',*,*,#5917,.T.) ;
#8047=ORIENTED_EDGE('',*,*,#5918,.T.) ;
#8048=ORIENTED_EDGE('',*,*,#5919,.F.) ;
#8049=ORIENTED_EDGE('',*,*,#5920,.T.) ;
#8050=ORIENTED_EDGE('',*,*,#5921,.T.) ;
#8051=ORIENTED_EDGE('',*,*,#5922,.T.) ;
#8052=ORIENTED_EDGE('',*,*,#5923,.F.) ;
#8053=ORIENTED_EDGE('',*,*,#5924,.T.) ;
#8054=ORIENTED_EDGE('',*,*,#5925,.T.) ;
#8055=ORIENTED_EDGE('',*,*,#5926,.T.) ;
#8056=ORIENTED_EDGE('',*,*,#5927,.F.) ;
#8057=ORIENTED_EDGE('',*,*,#5928,.T.) ;
#8058=ORIENTED_EDGE('',*,*,#5929,.T.) ;
#8059=ORIENTED_EDGE('',*,*,#5930,.T.) ;
#8060=ORIENTED_EDGE('',*,*,#5931,.F.) ;
#8061=ORIENTED_EDGE('',*,*,#5932,.T.) ;
#8062=ORIENTED_EDGE('',*,*,#5933,.T.) ;
#8063=ORIENTED_EDGE('',*,*,#5934,.T.) ;
#8064=ORIENTED_EDGE('',*,*,#5935,.F.) ;
#8065=ORIENTED_EDGE('',*,*,#5936,.T.) ;
#8066=ORIENTED_EDGE('',*,*,#5937,.T.) ;
#8067=ORIENTED_EDGE('',*,*,#5938,.T.) ;
#8068=ORIENTED_EDGE('',*,*,#5939,.F.) ;
#8069=ORIENTED_EDGE('',*,*,#5940,.T.) ;
#8070=ORIENTED_EDGE('',*,*,#5941,.T.) ;
#8071=ORIENTED_EDGE('',*,*,#5942,.T.) ;
#8072=ORIENTED_EDGE('',*,*,#5943,.F.) ;
#8073=ORIENTED_EDGE('',*,*,#5944,.T.) ;
#8074=ORIENTED_EDGE('',*,*,#5945,.T.) ;
#8075=ORIENTED_EDGE('',*,*,#5946,.T.) ;
#8076=ORIENTED_EDGE('',*,*,#5947,.F.) ;
#8077=ORIENTED_EDGE('',*,*,#5948,.T.) ;
#8078=ORIENTED_EDGE('',*,*,#5949,.T.) ;
#8079=ORIENTED_EDGE('',*,*,#5950,.T.) ;
#8080=ORIENTED_EDGE('',*,*,#5951,.F.) ;
#8081=ORIENTED_EDGE('',*,*,#5952,.T.) ;
#8082=ORIENTED_EDGE('',*,*,#5953,.T.) ;
#8083=ORIENTED_EDGE('',*,*,#5954,.T.) ;
#8084=ORIENTED_EDGE('',*,*,#5955,.F.) ;
#8085=ORIENTED_EDGE('',*,*,#5956,.T.) ;
#8086=ORIENTED_EDGE('',*,*,#5957,.T.) ;
#8087=ORIENTED_EDGE('',*,*,#5958,.T.) ;
#8088=ORIENTED_EDGE('',*,*,#5959,.F.) ;
#8089=ORIENTED_EDGE('',*,*,#5960,.T.) ;
#8090=ORIENTED_EDGE('',*,*,#5961,.T.) ;
#8091=ORIENTED_EDGE('',*,*,#5962,.T.) ;
#8092=ORIENTED_EDGE('',*,*,#5963,.F.) ;
#8093=ORIENTED_EDGE('',*,*,#5964,.T.) ;
#8094=ORIENTED_EDGE('',*,*,#5965,.T.) ;
#8095=ORIENTED_EDGE('',*,*,#5966,.T.) ;
#8096=ORIENTED_EDGE('',*,*,#5967,.F.) ;
#8097=ORIENTED_EDGE('',*,*,#5966,.F.) ;
#8098=ORIENTED_EDGE('',*,*,#5968,.T.) ;
#8099=ORIENTED_EDGE('',*,*,#5969,.F.) ;
#8100=ORIENTED_EDGE('',*,*,#5970,.F.) ;
#8101=ORIENTED_EDGE('',*,*,#5971,.F.) ;
#8102=ORIENTED_EDGE('',*,*,#5969,.T.) ;
#8103=ORIENTED_EDGE('',*,*,#5972,.T.) ;
#8104=ORIENTED_EDGE('',*,*,#5964,.F.) ;
#8105=ORIENTED_EDGE('',*,*,#5965,.F.) ;
#8106=ORIENTED_EDGE('',*,*,#5972,.F.) ;
#8107=ORIENTED_EDGE('',*,*,#5968,.F.) ;
#8108=ORIENTED_EDGE('',*,*,#5973,.T.) ;
#8109=ORIENTED_EDGE('',*,*,#5974,.T.) ;
#8110=ORIENTED_EDGE('',*,*,#5975,.T.) ;
#8111=ORIENTED_EDGE('',*,*,#5896,.T.) ;
#8112=ORIENTED_EDGE('',*,*,#5976,.T.) ;
#8113=ORIENTED_EDGE('',*,*,#5977,.T.) ;
#8114=ORIENTED_EDGE('',*,*,#5892,.T.) ;
#8115=ORIENTED_EDGE('',*,*,#5978,.T.) ;
#8116=ORIENTED_EDGE('',*,*,#5979,.T.) ;
#8117=ORIENTED_EDGE('',*,*,#5888,.T.) ;
#8118=ORIENTED_EDGE('',*,*,#5980,.T.) ;
#8119=ORIENTED_EDGE('',*,*,#5981,.T.) ;
#8120=ORIENTED_EDGE('',*,*,#5884,.T.) ;
#8121=ORIENTED_EDGE('',*,*,#5982,.T.) ;
#8122=ORIENTED_EDGE('',*,*,#5983,.T.) ;
#8123=ORIENTED_EDGE('',*,*,#5880,.T.) ;
#8124=ORIENTED_EDGE('',*,*,#5984,.T.) ;
#8125=ORIENTED_EDGE('',*,*,#5985,.T.) ;
#8126=ORIENTED_EDGE('',*,*,#5876,.T.) ;
#8127=ORIENTED_EDGE('',*,*,#5986,.T.) ;
#8128=ORIENTED_EDGE('',*,*,#5987,.T.) ;
#8129=ORIENTED_EDGE('',*,*,#5872,.T.) ;
#8130=ORIENTED_EDGE('',*,*,#5988,.T.) ;
#8131=ORIENTED_EDGE('',*,*,#5989,.T.) ;
#8132=ORIENTED_EDGE('',*,*,#5868,.T.) ;
#8133=ORIENTED_EDGE('',*,*,#5990,.T.) ;
#8134=ORIENTED_EDGE('',*,*,#5991,.T.) ;
#8135=ORIENTED_EDGE('',*,*,#5864,.T.) ;
#8136=ORIENTED_EDGE('',*,*,#5992,.T.) ;
#8137=ORIENTED_EDGE('',*,*,#5993,.T.) ;
#8138=ORIENTED_EDGE('',*,*,#5860,.T.) ;
#8139=ORIENTED_EDGE('',*,*,#5994,.T.) ;
#8140=ORIENTED_EDGE('',*,*,#5995,.T.) ;
#8141=ORIENTED_EDGE('',*,*,#5856,.T.) ;
#8142=ORIENTED_EDGE('',*,*,#5996,.T.) ;
#8143=ORIENTED_EDGE('',*,*,#5997,.T.) ;
#8144=ORIENTED_EDGE('',*,*,#5852,.T.) ;
#8145=ORIENTED_EDGE('',*,*,#5998,.T.) ;
#8146=ORIENTED_EDGE('',*,*,#5999,.T.) ;
#8147=ORIENTED_EDGE('',*,*,#5848,.T.) ;
#8148=ORIENTED_EDGE('',*,*,#6000,.T.) ;
#8149=ORIENTED_EDGE('',*,*,#6001,.T.) ;
#8150=ORIENTED_EDGE('',*,*,#5844,.T.) ;
#8151=ORIENTED_EDGE('',*,*,#6002,.T.) ;
#8152=ORIENTED_EDGE('',*,*,#6003,.T.) ;
#8153=ORIENTED_EDGE('',*,*,#5840,.T.) ;
#8154=ORIENTED_EDGE('',*,*,#6004,.T.) ;
#8155=ORIENTED_EDGE('',*,*,#6005,.T.) ;
#8156=ORIENTED_EDGE('',*,*,#5836,.T.) ;
#8157=ORIENTED_EDGE('',*,*,#6006,.T.) ;
#8158=ORIENTED_EDGE('',*,*,#6007,.T.) ;
#8159=ORIENTED_EDGE('',*,*,#5832,.T.) ;
#8160=ORIENTED_EDGE('',*,*,#6008,.T.) ;
#8161=ORIENTED_EDGE('',*,*,#6009,.T.) ;
#8162=ORIENTED_EDGE('',*,*,#5828,.T.) ;
#8163=ORIENTED_EDGE('',*,*,#6010,.T.) ;
#8164=ORIENTED_EDGE('',*,*,#6011,.T.) ;
#8165=ORIENTED_EDGE('',*,*,#5824,.T.) ;
#8166=ORIENTED_EDGE('',*,*,#5821,.T.) ;
#8167=ORIENTED_EDGE('',*,*,#5823,.T.) ;
#8168=ORIENTED_EDGE('',*,*,#5967,.T.) ;
#8169=ORIENTED_EDGE('',*,*,#5970,.T.) ;
#8170=ORIENTED_EDGE('',*,*,#5971,.T.) ;
#8171=ORIENTED_EDGE('',*,*,#5963,.T.) ;
#8172=ORIENTED_EDGE('',*,*,#6012,.T.) ;
#8173=ORIENTED_EDGE('',*,*,#6013,.T.) ;
#8174=ORIENTED_EDGE('',*,*,#5959,.T.) ;
#8175=ORIENTED_EDGE('',*,*,#6014,.T.) ;
#8176=ORIENTED_EDGE('',*,*,#6015,.T.) ;
#8177=ORIENTED_EDGE('',*,*,#5955,.T.) ;
#8178=ORIENTED_EDGE('',*,*,#6016,.T.) ;
#8179=ORIENTED_EDGE('',*,*,#6017,.T.) ;
#8180=ORIENTED_EDGE('',*,*,#5951,.T.) ;
#8181=ORIENTED_EDGE('',*,*,#6018,.T.) ;
#8182=ORIENTED_EDGE('',*,*,#6019,.T.) ;
#8183=ORIENTED_EDGE('',*,*,#5947,.T.) ;
#8184=ORIENTED_EDGE('',*,*,#6020,.T.) ;
#8185=ORIENTED_EDGE('',*,*,#6021,.T.) ;
#8186=ORIENTED_EDGE('',*,*,#5943,.T.) ;
#8187=ORIENTED_EDGE('',*,*,#6022,.T.) ;
#8188=ORIENTED_EDGE('',*,*,#6023,.T.) ;
#8189=ORIENTED_EDGE('',*,*,#5939,.T.) ;
#8190=ORIENTED_EDGE('',*,*,#6024,.T.) ;
#8191=ORIENTED_EDGE('',*,*,#6025,.T.) ;
#8192=ORIENTED_EDGE('',*,*,#5935,.T.) ;
#8193=ORIENTED_EDGE('',*,*,#6026,.T.) ;
#8194=ORIENTED_EDGE('',*,*,#6027,.T.) ;
#8195=ORIENTED_EDGE('',*,*,#5931,.T.) ;
#8196=ORIENTED_EDGE('',*,*,#6028,.T.) ;
#8197=ORIENTED_EDGE('',*,*,#6029,.T.) ;
#8198=ORIENTED_EDGE('',*,*,#5927,.T.) ;
#8199=ORIENTED_EDGE('',*,*,#6030,.T.) ;
#8200=ORIENTED_EDGE('',*,*,#6031,.T.) ;
#8201=ORIENTED_EDGE('',*,*,#5923,.T.) ;
#8202=ORIENTED_EDGE('',*,*,#6032,.T.) ;
#8203=ORIENTED_EDGE('',*,*,#6033,.T.) ;
#8204=ORIENTED_EDGE('',*,*,#5919,.T.) ;
#8205=ORIENTED_EDGE('',*,*,#6034,.T.) ;
#8206=ORIENTED_EDGE('',*,*,#6035,.T.) ;
#8207=ORIENTED_EDGE('',*,*,#5915,.T.) ;
#8208=ORIENTED_EDGE('',*,*,#6036,.T.) ;
#8209=ORIENTED_EDGE('',*,*,#6037,.T.) ;
#8210=ORIENTED_EDGE('',*,*,#5911,.T.) ;
#8211=ORIENTED_EDGE('',*,*,#6038,.T.) ;
#8212=ORIENTED_EDGE('',*,*,#6039,.T.) ;
#8213=ORIENTED_EDGE('',*,*,#5907,.T.) ;
#8214=ORIENTED_EDGE('',*,*,#6040,.T.) ;
#8215=ORIENTED_EDGE('',*,*,#6041,.T.) ;
#8216=ORIENTED_EDGE('',*,*,#5903,.T.) ;
#8217=ORIENTED_EDGE('',*,*,#6042,.T.) ;
#8218=ORIENTED_EDGE('',*,*,#5974,.F.) ;
#8219=ORIENTED_EDGE('',*,*,#5961,.F.) ;
#8220=ORIENTED_EDGE('',*,*,#6043,.F.) ;
#8221=ORIENTED_EDGE('',*,*,#6044,.F.) ;
#8222=ORIENTED_EDGE('',*,*,#5962,.F.) ;
#8223=ORIENTED_EDGE('',*,*,#6044,.T.) ;
#8224=ORIENTED_EDGE('',*,*,#6045,.F.) ;
#8225=ORIENTED_EDGE('',*,*,#6012,.F.) ;
#8226=ORIENTED_EDGE('',*,*,#5960,.F.) ;
#8227=ORIENTED_EDGE('',*,*,#6013,.F.) ;
#8228=ORIENTED_EDGE('',*,*,#6045,.T.) ;
#8229=ORIENTED_EDGE('',*,*,#6043,.T.) ;
#8230=ORIENTED_EDGE('',*,*,#5958,.F.) ;
#8231=ORIENTED_EDGE('',*,*,#6046,.T.) ;
#8232=ORIENTED_EDGE('',*,*,#6047,.F.) ;
#8233=ORIENTED_EDGE('',*,*,#6014,.F.) ;
#8234=ORIENTED_EDGE('',*,*,#6015,.F.) ;
#8235=ORIENTED_EDGE('',*,*,#6047,.T.) ;
#8236=ORIENTED_EDGE('',*,*,#6048,.T.) ;
#8237=ORIENTED_EDGE('',*,*,#5956,.F.) ;
#8238=ORIENTED_EDGE('',*,*,#5957,.F.) ;
#8239=ORIENTED_EDGE('',*,*,#6048,.F.) ;
#8240=ORIENTED_EDGE('',*,*,#6046,.F.) ;
#8241=ORIENTED_EDGE('',*,*,#5953,.F.) ;
#8242=ORIENTED_EDGE('',*,*,#6049,.F.) ;
#8243=ORIENTED_EDGE('',*,*,#6050,.F.) ;
#8244=ORIENTED_EDGE('',*,*,#5954,.F.) ;
#8245=ORIENTED_EDGE('',*,*,#6050,.T.) ;
#8246=ORIENTED_EDGE('',*,*,#6051,.F.) ;
#8247=ORIENTED_EDGE('',*,*,#6016,.F.) ;
#8248=ORIENTED_EDGE('',*,*,#5952,.F.) ;
#8249=ORIENTED_EDGE('',*,*,#6017,.F.) ;
#8250=ORIENTED_EDGE('',*,*,#6051,.T.) ;
#8251=ORIENTED_EDGE('',*,*,#6049,.T.) ;
#8252=ORIENTED_EDGE('',*,*,#5950,.F.) ;
#8253=ORIENTED_EDGE('',*,*,#6052,.T.) ;
#8254=ORIENTED_EDGE('',*,*,#6053,.F.) ;
#8255=ORIENTED_EDGE('',*,*,#6018,.F.) ;
#8256=ORIENTED_EDGE('',*,*,#6019,.F.) ;
#8257=ORIENTED_EDGE('',*,*,#6053,.T.) ;
#8258=ORIENTED_EDGE('',*,*,#6054,.T.) ;
#8259=ORIENTED_EDGE('',*,*,#5948,.F.) ;
#8260=ORIENTED_EDGE('',*,*,#5949,.F.) ;
#8261=ORIENTED_EDGE('',*,*,#6054,.F.) ;
#8262=ORIENTED_EDGE('',*,*,#6052,.F.) ;
#8263=ORIENTED_EDGE('',*,*,#5945,.F.) ;
#8264=ORIENTED_EDGE('',*,*,#6055,.F.) ;
#8265=ORIENTED_EDGE('',*,*,#6056,.F.) ;
#8266=ORIENTED_EDGE('',*,*,#5946,.F.) ;
#8267=ORIENTED_EDGE('',*,*,#6056,.T.) ;
#8268=ORIENTED_EDGE('',*,*,#6057,.F.) ;
#8269=ORIENTED_EDGE('',*,*,#6020,.F.) ;
#8270=ORIENTED_EDGE('',*,*,#5944,.F.) ;
#8271=ORIENTED_EDGE('',*,*,#6021,.F.) ;
#8272=ORIENTED_EDGE('',*,*,#6057,.T.) ;
#8273=ORIENTED_EDGE('',*,*,#6055,.T.) ;
#8274=ORIENTED_EDGE('',*,*,#5942,.F.) ;
#8275=ORIENTED_EDGE('',*,*,#6058,.T.) ;
#8276=ORIENTED_EDGE('',*,*,#6059,.F.) ;
#8277=ORIENTED_EDGE('',*,*,#6022,.F.) ;
#8278=ORIENTED_EDGE('',*,*,#6023,.F.) ;
#8279=ORIENTED_EDGE('',*,*,#6059,.T.) ;
#8280=ORIENTED_EDGE('',*,*,#6060,.T.) ;
#8281=ORIENTED_EDGE('',*,*,#5940,.F.) ;
#8282=ORIENTED_EDGE('',*,*,#5941,.F.) ;
#8283=ORIENTED_EDGE('',*,*,#6060,.F.) ;
#8284=ORIENTED_EDGE('',*,*,#6058,.F.) ;
#8285=ORIENTED_EDGE('',*,*,#5937,.F.) ;
#8286=ORIENTED_EDGE('',*,*,#6061,.F.) ;
#8287=ORIENTED_EDGE('',*,*,#6062,.F.) ;
#8288=ORIENTED_EDGE('',*,*,#5938,.F.) ;
#8289=ORIENTED_EDGE('',*,*,#6062,.T.) ;
#8290=ORIENTED_EDGE('',*,*,#6063,.F.) ;
#8291=ORIENTED_EDGE('',*,*,#6024,.F.) ;
#8292=ORIENTED_EDGE('',*,*,#5936,.F.) ;
#8293=ORIENTED_EDGE('',*,*,#6025,.F.) ;
#8294=ORIENTED_EDGE('',*,*,#6063,.T.) ;
#8295=ORIENTED_EDGE('',*,*,#6061,.T.) ;
#8296=ORIENTED_EDGE('',*,*,#5934,.F.) ;
#8297=ORIENTED_EDGE('',*,*,#6064,.T.) ;
#8298=ORIENTED_EDGE('',*,*,#6065,.F.) ;
#8299=ORIENTED_EDGE('',*,*,#6026,.F.) ;
#8300=ORIENTED_EDGE('',*,*,#6027,.F.) ;
#8301=ORIENTED_EDGE('',*,*,#6065,.T.) ;
#8302=ORIENTED_EDGE('',*,*,#6066,.T.) ;
#8303=ORIENTED_EDGE('',*,*,#5932,.F.) ;
#8304=ORIENTED_EDGE('',*,*,#5933,.F.) ;
#8305=ORIENTED_EDGE('',*,*,#6066,.F.) ;
#8306=ORIENTED_EDGE('',*,*,#6064,.F.) ;
#8307=ORIENTED_EDGE('',*,*,#5929,.F.) ;
#8308=ORIENTED_EDGE('',*,*,#6067,.F.) ;
#8309=ORIENTED_EDGE('',*,*,#6068,.F.) ;
#8310=ORIENTED_EDGE('',*,*,#5930,.F.) ;
#8311=ORIENTED_EDGE('',*,*,#6068,.T.) ;
#8312=ORIENTED_EDGE('',*,*,#6069,.F.) ;
#8313=ORIENTED_EDGE('',*,*,#6028,.F.) ;
#8314=ORIENTED_EDGE('',*,*,#5928,.F.) ;
#8315=ORIENTED_EDGE('',*,*,#6029,.F.) ;
#8316=ORIENTED_EDGE('',*,*,#6069,.T.) ;
#8317=ORIENTED_EDGE('',*,*,#6067,.T.) ;
#8318=ORIENTED_EDGE('',*,*,#5926,.F.) ;
#8319=ORIENTED_EDGE('',*,*,#6070,.T.) ;
#8320=ORIENTED_EDGE('',*,*,#6071,.F.) ;
#8321=ORIENTED_EDGE('',*,*,#6030,.F.) ;
#8322=ORIENTED_EDGE('',*,*,#6031,.F.) ;
#8323=ORIENTED_EDGE('',*,*,#6071,.T.) ;
#8324=ORIENTED_EDGE('',*,*,#6072,.T.) ;
#8325=ORIENTED_EDGE('',*,*,#5924,.F.) ;
#8326=ORIENTED_EDGE('',*,*,#5925,.F.) ;
#8327=ORIENTED_EDGE('',*,*,#6072,.F.) ;
#8328=ORIENTED_EDGE('',*,*,#6070,.F.) ;
#8329=ORIENTED_EDGE('',*,*,#5921,.F.) ;
#8330=ORIENTED_EDGE('',*,*,#6073,.F.) ;
#8331=ORIENTED_EDGE('',*,*,#6074,.F.) ;
#8332=ORIENTED_EDGE('',*,*,#5922,.F.) ;
#8333=ORIENTED_EDGE('',*,*,#6074,.T.) ;
#8334=ORIENTED_EDGE('',*,*,#6075,.F.) ;
#8335=ORIENTED_EDGE('',*,*,#6032,.F.) ;
#8336=ORIENTED_EDGE('',*,*,#5920,.F.) ;
#8337=ORIENTED_EDGE('',*,*,#6033,.F.) ;
#8338=ORIENTED_EDGE('',*,*,#6075,.T.) ;
#8339=ORIENTED_EDGE('',*,*,#6073,.T.) ;
#8340=ORIENTED_EDGE('',*,*,#5918,.F.) ;
#8341=ORIENTED_EDGE('',*,*,#6076,.T.) ;
#8342=ORIENTED_EDGE('',*,*,#6077,.F.) ;
#8343=ORIENTED_EDGE('',*,*,#6034,.F.) ;
#8344=ORIENTED_EDGE('',*,*,#6035,.F.) ;
#8345=ORIENTED_EDGE('',*,*,#6077,.T.) ;
#8346=ORIENTED_EDGE('',*,*,#6078,.T.) ;
#8347=ORIENTED_EDGE('',*,*,#5916,.F.) ;
#8348=ORIENTED_EDGE('',*,*,#5917,.F.) ;
#8349=ORIENTED_EDGE('',*,*,#6078,.F.) ;
#8350=ORIENTED_EDGE('',*,*,#6076,.F.) ;
#8351=ORIENTED_EDGE('',*,*,#5913,.F.) ;
#8352=ORIENTED_EDGE('',*,*,#6079,.F.) ;
#8353=ORIENTED_EDGE('',*,*,#6080,.F.) ;
#8354=ORIENTED_EDGE('',*,*,#5914,.F.) ;
#8355=ORIENTED_EDGE('',*,*,#6080,.T.) ;
#8356=ORIENTED_EDGE('',*,*,#6081,.F.) ;
#8357=ORIENTED_EDGE('',*,*,#6036,.F.) ;
#8358=ORIENTED_EDGE('',*,*,#5912,.F.) ;
#8359=ORIENTED_EDGE('',*,*,#6037,.F.) ;
#8360=ORIENTED_EDGE('',*,*,#6081,.T.) ;
#8361=ORIENTED_EDGE('',*,*,#6079,.T.) ;
#8362=ORIENTED_EDGE('',*,*,#5910,.F.) ;
#8363=ORIENTED_EDGE('',*,*,#6082,.T.) ;
#8364=ORIENTED_EDGE('',*,*,#6083,.F.) ;
#8365=ORIENTED_EDGE('',*,*,#6038,.F.) ;
#8366=ORIENTED_EDGE('',*,*,#6039,.F.) ;
#8367=ORIENTED_EDGE('',*,*,#6083,.T.) ;
#8368=ORIENTED_EDGE('',*,*,#6084,.T.) ;
#8369=ORIENTED_EDGE('',*,*,#5908,.F.) ;
#8370=ORIENTED_EDGE('',*,*,#5909,.F.) ;
#8371=ORIENTED_EDGE('',*,*,#6084,.F.) ;
#8372=ORIENTED_EDGE('',*,*,#6082,.F.) ;
#8373=ORIENTED_EDGE('',*,*,#5905,.F.) ;
#8374=ORIENTED_EDGE('',*,*,#6085,.F.) ;
#8375=ORIENTED_EDGE('',*,*,#6086,.F.) ;
#8376=ORIENTED_EDGE('',*,*,#5906,.F.) ;
#8377=ORIENTED_EDGE('',*,*,#6086,.T.) ;
#8378=ORIENTED_EDGE('',*,*,#6087,.F.) ;
#8379=ORIENTED_EDGE('',*,*,#6040,.F.) ;
#8380=ORIENTED_EDGE('',*,*,#5904,.F.) ;
#8381=ORIENTED_EDGE('',*,*,#6041,.F.) ;
#8382=ORIENTED_EDGE('',*,*,#6087,.T.) ;
#8383=ORIENTED_EDGE('',*,*,#6085,.T.) ;
#8384=ORIENTED_EDGE('',*,*,#5902,.F.) ;
#8385=ORIENTED_EDGE('',*,*,#6088,.T.) ;
#8386=ORIENTED_EDGE('',*,*,#6089,.F.) ;
#8387=ORIENTED_EDGE('',*,*,#6042,.F.) ;
#8388=ORIENTED_EDGE('',*,*,#5975,.F.) ;
#8389=ORIENTED_EDGE('',*,*,#6089,.T.) ;
#8390=ORIENTED_EDGE('',*,*,#6090,.T.) ;
#8391=ORIENTED_EDGE('',*,*,#5897,.F.) ;
#8392=ORIENTED_EDGE('',*,*,#5898,.F.) ;
#8393=ORIENTED_EDGE('',*,*,#6090,.F.) ;
#8394=ORIENTED_EDGE('',*,*,#6088,.F.) ;
#8395=ORIENTED_EDGE('',*,*,#5901,.F.) ;
#8396=ORIENTED_EDGE('',*,*,#5894,.F.) ;
#8397=ORIENTED_EDGE('',*,*,#6091,.F.) ;
#8398=ORIENTED_EDGE('',*,*,#6092,.F.) ;
#8399=ORIENTED_EDGE('',*,*,#5895,.F.) ;
#8400=ORIENTED_EDGE('',*,*,#6092,.T.) ;
#8401=ORIENTED_EDGE('',*,*,#6093,.F.) ;
#8402=ORIENTED_EDGE('',*,*,#5976,.F.) ;
#8403=ORIENTED_EDGE('',*,*,#5893,.F.) ;
#8404=ORIENTED_EDGE('',*,*,#5977,.F.) ;
#8405=ORIENTED_EDGE('',*,*,#6093,.T.) ;
#8406=ORIENTED_EDGE('',*,*,#6091,.T.) ;
#8407=ORIENTED_EDGE('',*,*,#5891,.F.) ;
#8408=ORIENTED_EDGE('',*,*,#6094,.T.) ;
#8409=ORIENTED_EDGE('',*,*,#6095,.F.) ;
#8410=ORIENTED_EDGE('',*,*,#5978,.F.) ;
#8411=ORIENTED_EDGE('',*,*,#5979,.F.) ;
#8412=ORIENTED_EDGE('',*,*,#6095,.T.) ;
#8413=ORIENTED_EDGE('',*,*,#6096,.T.) ;
#8414=ORIENTED_EDGE('',*,*,#5889,.F.) ;
#8415=ORIENTED_EDGE('',*,*,#5890,.F.) ;
#8416=ORIENTED_EDGE('',*,*,#6096,.F.) ;
#8417=ORIENTED_EDGE('',*,*,#6094,.F.) ;
#8418=ORIENTED_EDGE('',*,*,#5886,.F.) ;
#8419=ORIENTED_EDGE('',*,*,#6097,.F.) ;
#8420=ORIENTED_EDGE('',*,*,#6098,.F.) ;
#8421=ORIENTED_EDGE('',*,*,#5887,.F.) ;
#8422=ORIENTED_EDGE('',*,*,#6098,.T.) ;
#8423=ORIENTED_EDGE('',*,*,#6099,.F.) ;
#8424=ORIENTED_EDGE('',*,*,#5980,.F.) ;
#8425=ORIENTED_EDGE('',*,*,#5885,.F.) ;
#8426=ORIENTED_EDGE('',*,*,#5981,.F.) ;
#8427=ORIENTED_EDGE('',*,*,#6099,.T.) ;
#8428=ORIENTED_EDGE('',*,*,#6097,.T.) ;
#8429=ORIENTED_EDGE('',*,*,#5883,.F.) ;
#8430=ORIENTED_EDGE('',*,*,#6100,.T.) ;
#8431=ORIENTED_EDGE('',*,*,#6101,.F.) ;
#8432=ORIENTED_EDGE('',*,*,#5982,.F.) ;
#8433=ORIENTED_EDGE('',*,*,#5983,.F.) ;
#8434=ORIENTED_EDGE('',*,*,#6101,.T.) ;
#8435=ORIENTED_EDGE('',*,*,#6102,.T.) ;
#8436=ORIENTED_EDGE('',*,*,#5881,.F.) ;
#8437=ORIENTED_EDGE('',*,*,#5882,.F.) ;
#8438=ORIENTED_EDGE('',*,*,#6102,.F.) ;
#8439=ORIENTED_EDGE('',*,*,#6100,.F.) ;
#8440=ORIENTED_EDGE('',*,*,#5878,.F.) ;
#8441=ORIENTED_EDGE('',*,*,#6103,.F.) ;
#8442=ORIENTED_EDGE('',*,*,#6104,.F.) ;
#8443=ORIENTED_EDGE('',*,*,#5879,.F.) ;
#8444=ORIENTED_EDGE('',*,*,#6104,.T.) ;
#8445=ORIENTED_EDGE('',*,*,#6105,.F.) ;
#8446=ORIENTED_EDGE('',*,*,#5984,.F.) ;
#8447=ORIENTED_EDGE('',*,*,#5877,.F.) ;
#8448=ORIENTED_EDGE('',*,*,#5985,.F.) ;
#8449=ORIENTED_EDGE('',*,*,#6105,.T.) ;
#8450=ORIENTED_EDGE('',*,*,#6103,.T.) ;
#8451=ORIENTED_EDGE('',*,*,#5875,.F.) ;
#8452=ORIENTED_EDGE('',*,*,#6106,.T.) ;
#8453=ORIENTED_EDGE('',*,*,#6107,.F.) ;
#8454=ORIENTED_EDGE('',*,*,#5986,.F.) ;
#8455=ORIENTED_EDGE('',*,*,#5987,.F.) ;
#8456=ORIENTED_EDGE('',*,*,#6107,.T.) ;
#8457=ORIENTED_EDGE('',*,*,#6108,.T.) ;
#8458=ORIENTED_EDGE('',*,*,#5873,.F.) ;
#8459=ORIENTED_EDGE('',*,*,#5874,.F.) ;
#8460=ORIENTED_EDGE('',*,*,#6108,.F.) ;
#8461=ORIENTED_EDGE('',*,*,#6106,.F.) ;
#8462=ORIENTED_EDGE('',*,*,#5870,.F.) ;
#8463=ORIENTED_EDGE('',*,*,#6109,.F.) ;
#8464=ORIENTED_EDGE('',*,*,#6110,.F.) ;
#8465=ORIENTED_EDGE('',*,*,#5871,.F.) ;
#8466=ORIENTED_EDGE('',*,*,#6110,.T.) ;
#8467=ORIENTED_EDGE('',*,*,#6111,.F.) ;
#8468=ORIENTED_EDGE('',*,*,#5988,.F.) ;
#8469=ORIENTED_EDGE('',*,*,#5869,.F.) ;
#8470=ORIENTED_EDGE('',*,*,#5989,.F.) ;
#8471=ORIENTED_EDGE('',*,*,#6111,.T.) ;
#8472=ORIENTED_EDGE('',*,*,#6109,.T.) ;
#8473=ORIENTED_EDGE('',*,*,#5867,.F.) ;
#8474=ORIENTED_EDGE('',*,*,#6112,.T.) ;
#8475=ORIENTED_EDGE('',*,*,#6113,.F.) ;
#8476=ORIENTED_EDGE('',*,*,#5990,.F.) ;
#8477=ORIENTED_EDGE('',*,*,#5991,.F.) ;
#8478=ORIENTED_EDGE('',*,*,#6113,.T.) ;
#8479=ORIENTED_EDGE('',*,*,#6114,.T.) ;
#8480=ORIENTED_EDGE('',*,*,#5865,.F.) ;
#8481=ORIENTED_EDGE('',*,*,#5866,.F.) ;
#8482=ORIENTED_EDGE('',*,*,#6114,.F.) ;
#8483=ORIENTED_EDGE('',*,*,#6112,.F.) ;
#8484=ORIENTED_EDGE('',*,*,#5862,.F.) ;
#8485=ORIENTED_EDGE('',*,*,#6115,.F.) ;
#8486=ORIENTED_EDGE('',*,*,#6116,.F.) ;
#8487=ORIENTED_EDGE('',*,*,#5863,.F.) ;
#8488=ORIENTED_EDGE('',*,*,#6116,.T.) ;
#8489=ORIENTED_EDGE('',*,*,#6117,.F.) ;
#8490=ORIENTED_EDGE('',*,*,#5992,.F.) ;
#8491=ORIENTED_EDGE('',*,*,#5861,.F.) ;
#8492=ORIENTED_EDGE('',*,*,#5993,.F.) ;
#8493=ORIENTED_EDGE('',*,*,#6117,.T.) ;
#8494=ORIENTED_EDGE('',*,*,#6115,.T.) ;
#8495=ORIENTED_EDGE('',*,*,#5859,.F.) ;
#8496=ORIENTED_EDGE('',*,*,#6118,.T.) ;
#8497=ORIENTED_EDGE('',*,*,#6119,.F.) ;
#8498=ORIENTED_EDGE('',*,*,#5994,.F.) ;
#8499=ORIENTED_EDGE('',*,*,#5995,.F.) ;
#8500=ORIENTED_EDGE('',*,*,#6119,.T.) ;
#8501=ORIENTED_EDGE('',*,*,#6120,.T.) ;
#8502=ORIENTED_EDGE('',*,*,#5857,.F.) ;
#8503=ORIENTED_EDGE('',*,*,#5858,.F.) ;
#8504=ORIENTED_EDGE('',*,*,#6120,.F.) ;
#8505=ORIENTED_EDGE('',*,*,#6118,.F.) ;
#8506=ORIENTED_EDGE('',*,*,#5854,.F.) ;
#8507=ORIENTED_EDGE('',*,*,#6121,.F.) ;
#8508=ORIENTED_EDGE('',*,*,#6122,.F.) ;
#8509=ORIENTED_EDGE('',*,*,#5855,.F.) ;
#8510=ORIENTED_EDGE('',*,*,#6122,.T.) ;
#8511=ORIENTED_EDGE('',*,*,#6123,.F.) ;
#8512=ORIENTED_EDGE('',*,*,#5996,.F.) ;
#8513=ORIENTED_EDGE('',*,*,#5853,.F.) ;
#8514=ORIENTED_EDGE('',*,*,#5997,.F.) ;
#8515=ORIENTED_EDGE('',*,*,#6123,.T.) ;
#8516=ORIENTED_EDGE('',*,*,#6121,.T.) ;
#8517=ORIENTED_EDGE('',*,*,#5851,.F.) ;
#8518=ORIENTED_EDGE('',*,*,#6124,.T.) ;
#8519=ORIENTED_EDGE('',*,*,#6125,.F.) ;
#8520=ORIENTED_EDGE('',*,*,#5998,.F.) ;
#8521=ORIENTED_EDGE('',*,*,#5999,.F.) ;
#8522=ORIENTED_EDGE('',*,*,#6125,.T.) ;
#8523=ORIENTED_EDGE('',*,*,#6126,.T.) ;
#8524=ORIENTED_EDGE('',*,*,#5849,.F.) ;
#8525=ORIENTED_EDGE('',*,*,#5850,.F.) ;
#8526=ORIENTED_EDGE('',*,*,#6126,.F.) ;
#8527=ORIENTED_EDGE('',*,*,#6124,.F.) ;
#8528=ORIENTED_EDGE('',*,*,#5846,.F.) ;
#8529=ORIENTED_EDGE('',*,*,#6127,.F.) ;
#8530=ORIENTED_EDGE('',*,*,#6128,.F.) ;
#8531=ORIENTED_EDGE('',*,*,#5847,.F.) ;
#8532=ORIENTED_EDGE('',*,*,#6128,.T.) ;
#8533=ORIENTED_EDGE('',*,*,#6129,.F.) ;
#8534=ORIENTED_EDGE('',*,*,#6000,.F.) ;
#8535=ORIENTED_EDGE('',*,*,#5845,.F.) ;
#8536=ORIENTED_EDGE('',*,*,#6001,.F.) ;
#8537=ORIENTED_EDGE('',*,*,#6129,.T.) ;
#8538=ORIENTED_EDGE('',*,*,#6127,.T.) ;
#8539=ORIENTED_EDGE('',*,*,#5843,.F.) ;
#8540=ORIENTED_EDGE('',*,*,#6130,.T.) ;
#8541=ORIENTED_EDGE('',*,*,#6131,.F.) ;
#8542=ORIENTED_EDGE('',*,*,#6002,.F.) ;
#8543=ORIENTED_EDGE('',*,*,#6003,.F.) ;
#8544=ORIENTED_EDGE('',*,*,#6131,.T.) ;
#8545=ORIENTED_EDGE('',*,*,#6132,.T.) ;
#8546=ORIENTED_EDGE('',*,*,#5841,.F.) ;
#8547=ORIENTED_EDGE('',*,*,#5842,.F.) ;
#8548=ORIENTED_EDGE('',*,*,#6132,.F.) ;
#8549=ORIENTED_EDGE('',*,*,#6130,.F.) ;
#8550=ORIENTED_EDGE('',*,*,#5838,.F.) ;
#8551=ORIENTED_EDGE('',*,*,#6133,.F.) ;
#8552=ORIENTED_EDGE('',*,*,#6134,.F.) ;
#8553=ORIENTED_EDGE('',*,*,#5839,.F.) ;
#8554=ORIENTED_EDGE('',*,*,#6134,.T.) ;
#8555=ORIENTED_EDGE('',*,*,#6135,.F.) ;
#8556=ORIENTED_EDGE('',*,*,#6004,.F.) ;
#8557=ORIENTED_EDGE('',*,*,#5837,.F.) ;
#8558=ORIENTED_EDGE('',*,*,#6005,.F.) ;
#8559=ORIENTED_EDGE('',*,*,#6135,.T.) ;
#8560=ORIENTED_EDGE('',*,*,#6133,.T.) ;
#8561=ORIENTED_EDGE('',*,*,#5835,.F.) ;
#8562=ORIENTED_EDGE('',*,*,#6136,.T.) ;
#8563=ORIENTED_EDGE('',*,*,#6137,.F.) ;
#8564=ORIENTED_EDGE('',*,*,#6006,.F.) ;
#8565=ORIENTED_EDGE('',*,*,#6007,.F.) ;
#8566=ORIENTED_EDGE('',*,*,#6137,.T.) ;
#8567=ORIENTED_EDGE('',*,*,#6138,.T.) ;
#8568=ORIENTED_EDGE('',*,*,#5833,.F.) ;
#8569=ORIENTED_EDGE('',*,*,#5834,.F.) ;
#8570=ORIENTED_EDGE('',*,*,#6138,.F.) ;
#8571=ORIENTED_EDGE('',*,*,#6136,.F.) ;
#8572=ORIENTED_EDGE('',*,*,#5830,.F.) ;
#8573=ORIENTED_EDGE('',*,*,#6139,.F.) ;
#8574=ORIENTED_EDGE('',*,*,#6140,.F.) ;
#8575=ORIENTED_EDGE('',*,*,#5831,.F.) ;
#8576=ORIENTED_EDGE('',*,*,#6140,.T.) ;
#8577=ORIENTED_EDGE('',*,*,#6141,.F.) ;
#8578=ORIENTED_EDGE('',*,*,#6008,.F.) ;
#8579=ORIENTED_EDGE('',*,*,#5829,.F.) ;
#8580=ORIENTED_EDGE('',*,*,#6009,.F.) ;
#8581=ORIENTED_EDGE('',*,*,#6141,.T.) ;
#8582=ORIENTED_EDGE('',*,*,#6139,.T.) ;
#8583=ORIENTED_EDGE('',*,*,#5827,.F.) ;
#8584=ORIENTED_EDGE('',*,*,#6142,.T.) ;
#8585=ORIENTED_EDGE('',*,*,#6143,.F.) ;
#8586=ORIENTED_EDGE('',*,*,#6010,.F.) ;
#8587=ORIENTED_EDGE('',*,*,#6011,.F.) ;
#8588=ORIENTED_EDGE('',*,*,#6143,.T.) ;
#8589=ORIENTED_EDGE('',*,*,#6144,.T.) ;
#8590=ORIENTED_EDGE('',*,*,#5825,.F.) ;
#8591=ORIENTED_EDGE('',*,*,#5826,.F.) ;
#8592=ORIENTED_EDGE('',*,*,#6144,.F.) ;
#8593=ORIENTED_EDGE('',*,*,#6142,.F.) ;
#8594=ORIENTED_EDGE('',*,*,#5813,.T.) ;
#8595=ORIENTED_EDGE('',*,*,#6145,.T.) ;
#8596=ORIENTED_EDGE('',*,*,#5900,.T.) ;
#8597=ORIENTED_EDGE('',*,*,#6145,.F.) ;
#8598=ORIENTED_EDGE('',*,*,#5973,.F.) ;
#8599=ORIENTED_EDGE('',*,*,#6146,.T.) ;
#8600=ORIENTED_EDGE('',*,*,#6146,.F.) ;
#8601=ORIENTED_EDGE('',*,*,#6147,.T.) ;
#8602=ORIENTED_EDGE('',*,*,#6148,.F.) ;
#8603=ORIENTED_EDGE('',*,*,#6149,.T.) ;
#8604=ORIENTED_EDGE('',*,*,#6150,.F.) ;
#8605=ORIENTED_EDGE('',*,*,#6151,.F.) ;
#8606=ORIENTED_EDGE('',*,*,#6152,.T.) ;
#8607=ORIENTED_EDGE('',*,*,#6153,.F.) ;
#8608=ORIENTED_EDGE('',*,*,#6154,.F.) ;
#8609=ORIENTED_EDGE('',*,*,#6155,.T.) ;
#8610=ORIENTED_EDGE('',*,*,#6156,.F.) ;
#8611=ORIENTED_EDGE('',*,*,#6157,.F.) ;
#8612=ORIENTED_EDGE('',*,*,#6158,.T.) ;
#8613=ORIENTED_EDGE('',*,*,#6159,.F.) ;
#8614=ORIENTED_EDGE('',*,*,#6160,.F.) ;
#8615=ORIENTED_EDGE('',*,*,#6161,.T.) ;
#8616=ORIENTED_EDGE('',*,*,#6162,.F.) ;
#8617=ORIENTED_EDGE('',*,*,#6163,.F.) ;
#8618=ORIENTED_EDGE('',*,*,#6164,.T.) ;
#8619=ORIENTED_EDGE('',*,*,#6165,.F.) ;
#8620=ORIENTED_EDGE('',*,*,#6147,.F.) ;
#8621=ORIENTED_EDGE('',*,*,#6166,.F.) ;
#8622=ORIENTED_EDGE('',*,*,#6155,.F.) ;
#8623=ORIENTED_EDGE('',*,*,#6167,.F.) ;
#8624=ORIENTED_EDGE('',*,*,#6168,.F.) ;
#8625=ORIENTED_EDGE('',*,*,#6169,.F.) ;
#8626=ORIENTED_EDGE('',*,*,#6158,.F.) ;
#8627=ORIENTED_EDGE('',*,*,#6170,.F.) ;
#8628=ORIENTED_EDGE('',*,*,#6171,.F.) ;
#8629=ORIENTED_EDGE('',*,*,#6172,.F.) ;
#8630=ORIENTED_EDGE('',*,*,#6173,.F.) ;
#8631=ORIENTED_EDGE('',*,*,#6174,.F.) ;
#8632=ORIENTED_EDGE('',*,*,#6152,.F.) ;
#8633=ORIENTED_EDGE('',*,*,#6175,.F.) ;
#8634=ORIENTED_EDGE('',*,*,#6161,.F.) ;
#8635=ORIENTED_EDGE('',*,*,#6176,.F.) ;
#8636=ORIENTED_EDGE('',*,*,#6177,.F.) ;
#8637=ORIENTED_EDGE('',*,*,#6178,.F.) ;
#8638=ORIENTED_EDGE('',*,*,#6179,.F.) ;
#8639=ORIENTED_EDGE('',*,*,#6180,.F.) ;
#8640=ORIENTED_EDGE('',*,*,#6149,.F.) ;
#8641=ORIENTED_EDGE('',*,*,#6181,.F.) ;
#8642=ORIENTED_EDGE('',*,*,#6182,.F.) ;
#8643=ORIENTED_EDGE('',*,*,#6183,.F.) ;
#8644=ORIENTED_EDGE('',*,*,#6164,.F.) ;
#8645=ORIENTED_EDGE('',*,*,#6162,.T.) ;
#8646=ORIENTED_EDGE('',*,*,#6175,.T.) ;
#8647=ORIENTED_EDGE('',*,*,#6184,.F.) ;
#8648=ORIENTED_EDGE('',*,*,#6176,.T.) ;
#8649=ORIENTED_EDGE('',*,*,#6160,.T.) ;
#8650=ORIENTED_EDGE('',*,*,#6185,.T.) ;
#8651=ORIENTED_EDGE('',*,*,#6186,.T.) ;
#8652=ORIENTED_EDGE('',*,*,#6187,.F.) ;
#8653=ORIENTED_EDGE('',*,*,#6159,.T.) ;
#8654=ORIENTED_EDGE('',*,*,#6169,.T.) ;
#8655=ORIENTED_EDGE('',*,*,#6188,.F.) ;
#8656=ORIENTED_EDGE('',*,*,#6170,.T.) ;
#8657=ORIENTED_EDGE('',*,*,#6157,.T.) ;
#8658=ORIENTED_EDGE('',*,*,#6189,.T.) ;
#8659=ORIENTED_EDGE('',*,*,#6190,.T.) ;
#8660=ORIENTED_EDGE('',*,*,#6185,.F.) ;
#8661=ORIENTED_EDGE('',*,*,#6156,.T.) ;
#8662=ORIENTED_EDGE('',*,*,#6166,.T.) ;
#8663=ORIENTED_EDGE('',*,*,#6191,.F.) ;
#8664=ORIENTED_EDGE('',*,*,#6167,.T.) ;
#8665=ORIENTED_EDGE('',*,*,#6154,.T.) ;
#8666=ORIENTED_EDGE('',*,*,#6192,.T.) ;
#8667=ORIENTED_EDGE('',*,*,#6193,.T.) ;
#8668=ORIENTED_EDGE('',*,*,#6189,.F.) ;
#8669=ORIENTED_EDGE('',*,*,#6168,.T.) ;
#8670=ORIENTED_EDGE('',*,*,#6191,.T.) ;
#8671=ORIENTED_EDGE('',*,*,#6171,.T.) ;
#8672=ORIENTED_EDGE('',*,*,#6188,.T.) ;
#8673=ORIENTED_EDGE('',*,*,#6173,.T.) ;
#8674=ORIENTED_EDGE('',*,*,#6194,.T.) ;
#8675=ORIENTED_EDGE('',*,*,#6177,.T.) ;
#8676=ORIENTED_EDGE('',*,*,#6184,.T.) ;
#8677=ORIENTED_EDGE('',*,*,#6179,.T.) ;
#8678=ORIENTED_EDGE('',*,*,#6195,.T.) ;
#8679=ORIENTED_EDGE('',*,*,#6182,.T.) ;
#8680=ORIENTED_EDGE('',*,*,#6196,.T.) ;
#8681=ORIENTED_EDGE('',*,*,#6197,.F.) ;
#8682=ORIENTED_EDGE('',*,*,#6198,.T.) ;
#8683=ORIENTED_EDGE('',*,*,#6193,.F.) ;
#8684=ORIENTED_EDGE('',*,*,#6199,.T.) ;
#8685=ORIENTED_EDGE('',*,*,#6190,.F.) ;
#8686=ORIENTED_EDGE('',*,*,#6200,.T.) ;
#8687=ORIENTED_EDGE('',*,*,#6186,.F.) ;
#8688=ORIENTED_EDGE('',*,*,#6201,.T.) ;
#8689=ORIENTED_EDGE('',*,*,#6202,.F.) ;
#8690=ORIENTED_EDGE('',*,*,#6203,.T.) ;
#8691=ORIENTED_EDGE('',*,*,#6204,.F.) ;
#8692=ORIENTED_EDGE('',*,*,#6205,.T.) ;
#8693=ORIENTED_EDGE('',*,*,#6200,.F.) ;
#8694=ORIENTED_EDGE('',*,*,#6199,.F.) ;
#8695=ORIENTED_EDGE('',*,*,#6198,.F.) ;
#8696=ORIENTED_EDGE('',*,*,#6205,.F.) ;
#8697=ORIENTED_EDGE('',*,*,#6206,.T.) ;
#8698=ORIENTED_EDGE('',*,*,#6206,.F.) ;
#8699=ORIENTED_EDGE('',*,*,#6203,.F.) ;
#8700=ORIENTED_EDGE('',*,*,#6201,.F.) ;
#8701=ORIENTED_EDGE('',*,*,#6151,.T.) ;
#8702=ORIENTED_EDGE('',*,*,#6207,.T.) ;
#8703=ORIENTED_EDGE('',*,*,#6197,.T.) ;
#8704=ORIENTED_EDGE('',*,*,#6192,.F.) ;
#8705=ORIENTED_EDGE('',*,*,#6153,.T.) ;
#8706=ORIENTED_EDGE('',*,*,#6174,.T.) ;
#8707=ORIENTED_EDGE('',*,*,#6194,.F.) ;
#8708=ORIENTED_EDGE('',*,*,#6172,.T.) ;
#8709=ORIENTED_EDGE('',*,*,#6148,.T.) ;
#8710=ORIENTED_EDGE('',*,*,#6208,.T.) ;
#8711=ORIENTED_EDGE('',*,*,#6204,.T.) ;
#8712=ORIENTED_EDGE('',*,*,#6207,.F.) ;
#8713=ORIENTED_EDGE('',*,*,#6150,.T.) ;
#8714=ORIENTED_EDGE('',*,*,#6180,.T.) ;
#8715=ORIENTED_EDGE('',*,*,#6195,.F.) ;
#8716=ORIENTED_EDGE('',*,*,#6178,.T.) ;
#8717=ORIENTED_EDGE('',*,*,#6163,.T.) ;
#8718=ORIENTED_EDGE('',*,*,#6187,.T.) ;
#8719=ORIENTED_EDGE('',*,*,#6202,.T.) ;
#8720=ORIENTED_EDGE('',*,*,#6208,.F.) ;
#8721=ORIENTED_EDGE('',*,*,#6165,.T.) ;
#8722=ORIENTED_EDGE('',*,*,#6183,.T.) ;
#8723=ORIENTED_EDGE('',*,*,#6196,.F.) ;
#8724=ORIENTED_EDGE('',*,*,#6181,.T.) ;
#9015=CONICAL_SURFACE('',#10316,0.791749999999999,0.785398163397448) ;
#9016=CONICAL_SURFACE('',#10400,1.75,0.785398163397441) ;
#9017=CONICAL_SURFACE('',#10508,0.916025403784442,0.785398163397437) ;
#9018=CONICAL_SURFACE('',#10548,0.866025403784434,1.02974425867665) ;
#9308=ADVANCED_FACE('',(#1372),#596,.T.) ;
#9309=ADVANCED_FACE('',(#1373),#597,.T.) ;
#9310=ADVANCED_FACE('',(#1374),#598,.T.) ;
#9311=ADVANCED_FACE('',(#1375),#599,.T.) ;
#9312=ADVANCED_FACE('',(#1376),#600,.T.) ;
#9313=ADVANCED_FACE('',(#1377),#601,.T.) ;
#9314=ADVANCED_FACE('',(#1378),#602,.T.) ;
#9315=ADVANCED_FACE('',(#1379),#603,.T.) ;
#9316=ADVANCED_FACE('',(#1380),#604,.T.) ;
#9317=ADVANCED_FACE('',(#1381),#605,.T.) ;
#9318=ADVANCED_FACE('',(#1382),#606,.T.) ;
#9319=ADVANCED_FACE('',(#1383),#607,.T.) ;
#9320=ADVANCED_FACE('',(#1384),#608,.T.) ;
#9321=ADVANCED_FACE('',(#1385),#609,.T.) ;
#9322=ADVANCED_FACE('',(#1386),#610,.T.) ;
#9323=ADVANCED_FACE('',(#1387),#611,.T.) ;
#9324=ADVANCED_FACE('',(#1388),#612,.T.) ;
#9325=ADVANCED_FACE('',(#1389),#613,.T.) ;
#9326=ADVANCED_FACE('',(#1390),#614,.T.) ;
#9327=ADVANCED_FACE('',(#1391),#615,.T.) ;
#9328=ADVANCED_FACE('',(#1392),#616,.T.) ;
#9329=ADVANCED_FACE('',(#1393),#617,.T.) ;
#9330=ADVANCED_FACE('',(#1394),#618,.T.) ;
#9331=ADVANCED_FACE('',(#1395),#619,.T.) ;
#9332=ADVANCED_FACE('',(#1396),#620,.T.) ;
#9333=ADVANCED_FACE('',(#1397),#621,.T.) ;
#9334=ADVANCED_FACE('',(#1398),#622,.T.) ;
#9335=ADVANCED_FACE('',(#1399),#623,.T.) ;
#9336=ADVANCED_FACE('',(#1400),#920,.F.) ;
#9337=ADVANCED_FACE('',(#1401),#243,.F.) ;
#9338=ADVANCED_FACE('',(#1402),#921,.T.) ;
#9339=ADVANCED_FACE('',(#1403),#624,.T.) ;
#9340=ADVANCED_FACE('',(#1404),#244,.F.) ;
#9341=ADVANCED_FACE('',(#1405),#337,.F.) ;
#9342=ADVANCED_FACE('',(#1406),#625,.T.) ;
#9343=ADVANCED_FACE('',(#1407,#733),#922,.T.) ;
#9344=ADVANCED_FACE('',(#1408),#9015,.T.) ;
#9345=ADVANCED_FACE('',(#1409),#923,.T.) ;
#9346=ADVANCED_FACE('',(#1410),#924,.F.) ;
#9347=ADVANCED_FACE('',(#1411),#925,.F.) ;
#9348=ADVANCED_FACE('',(#1412),#926,.F.) ;
#9349=ADVANCED_FACE('',(#1413),#626,.T.) ;
#9350=ADVANCED_FACE('',(#1414),#927,.F.) ;
#9351=ADVANCED_FACE('',(#1415),#928,.F.) ;
#9352=ADVANCED_FACE('',(#1416),#929,.F.) ;
#9353=ADVANCED_FACE('',(#1417),#9016,.T.) ;
#9354=ADVANCED_FACE('',(#1418),#930,.F.) ;
#9355=ADVANCED_FACE('',(#1419),#931,.F.) ;
#9356=ADVANCED_FACE('',(#1420),#932,.F.) ;
#9357=ADVANCED_FACE('',(#1421),#933,.F.) ;
#9358=ADVANCED_FACE('',(#1422),#934,.F.) ;
#9359=ADVANCED_FACE('',(#1423),#935,.F.) ;
#9360=ADVANCED_FACE('',(#1424),#936,.F.) ;
#9361=ADVANCED_FACE('',(#1425),#937,.F.) ;
#9362=ADVANCED_FACE('',(#1426),#938,.F.) ;
#9363=ADVANCED_FACE('',(#1427),#939,.F.) ;
#9364=ADVANCED_FACE('',(#1428),#940,.F.) ;
#9365=ADVANCED_FACE('',(#1429),#941,.F.) ;
#9366=ADVANCED_FACE('',(#1430),#942,.F.) ;
#9367=ADVANCED_FACE('',(#1431),#943,.F.) ;
#9368=ADVANCED_FACE('',(#1432),#944,.F.) ;
#9369=ADVANCED_FACE('',(#1433),#945,.F.) ;
#9370=ADVANCED_FACE('',(#1434),#946,.F.) ;
#9371=ADVANCED_FACE('',(#1435),#947,.F.) ;
#9372=ADVANCED_FACE('',(#1436),#948,.F.) ;
#9373=ADVANCED_FACE('',(#1437),#949,.F.) ;
#9374=ADVANCED_FACE('',(#1438),#950,.F.) ;
#9375=ADVANCED_FACE('',(#1439),#951,.F.) ;
#9376=ADVANCED_FACE('',(#1440),#952,.F.) ;
#9377=ADVANCED_FACE('',(#1441),#953,.F.) ;
#9378=ADVANCED_FACE('',(#1442),#954,.F.) ;
#9379=ADVANCED_FACE('',(#1443),#955,.F.) ;
#9380=ADVANCED_FACE('',(#1444),#956,.F.) ;
#9381=ADVANCED_FACE('',(#1445),#957,.F.) ;
#9382=ADVANCED_FACE('',(#1446),#958,.F.) ;
#9383=ADVANCED_FACE('',(#1447),#959,.F.) ;
#9384=ADVANCED_FACE('',(#1448),#960,.F.) ;
#9385=ADVANCED_FACE('',(#1449),#961,.F.) ;
#9386=ADVANCED_FACE('',(#1450),#962,.F.) ;
#9387=ADVANCED_FACE('',(#1451),#963,.F.) ;
#9388=ADVANCED_FACE('',(#1452),#964,.F.) ;
#9389=ADVANCED_FACE('',(#1453),#965,.F.) ;
#9390=ADVANCED_FACE('',(#1454),#966,.F.) ;
#9391=ADVANCED_FACE('',(#1455),#967,.F.) ;
#9392=ADVANCED_FACE('',(#1456),#968,.F.) ;
#9393=ADVANCED_FACE('',(#1457),#969,.F.) ;
#9394=ADVANCED_FACE('',(#1458),#970,.F.) ;
#9395=ADVANCED_FACE('',(#1459),#971,.F.) ;
#9396=ADVANCED_FACE('',(#1460),#972,.F.) ;
#9397=ADVANCED_FACE('',(#1461),#973,.F.) ;
#9398=ADVANCED_FACE('',(#1462),#974,.F.) ;
#9399=ADVANCED_FACE('',(#1463),#975,.F.) ;
#9400=ADVANCED_FACE('',(#1464),#976,.F.) ;
#9401=ADVANCED_FACE('',(#1465),#977,.F.) ;
#9402=ADVANCED_FACE('',(#1466),#978,.F.) ;
#9403=ADVANCED_FACE('',(#1467),#979,.F.) ;
#9404=ADVANCED_FACE('',(#1468),#980,.F.) ;
#9405=ADVANCED_FACE('',(#1469),#981,.F.) ;
#9406=ADVANCED_FACE('',(#1470),#982,.F.) ;
#9407=ADVANCED_FACE('',(#1471),#983,.F.) ;
#9408=ADVANCED_FACE('',(#1472),#984,.F.) ;
#9409=ADVANCED_FACE('',(#1473),#985,.F.) ;
#9410=ADVANCED_FACE('',(#1474),#986,.F.) ;
#9411=ADVANCED_FACE('',(#1475),#987,.F.) ;
#9412=ADVANCED_FACE('',(#1476),#988,.F.) ;
#9413=ADVANCED_FACE('',(#1477),#989,.F.) ;
#9414=ADVANCED_FACE('',(#1478),#990,.F.) ;
#9415=ADVANCED_FACE('',(#1479),#991,.F.) ;
#9416=ADVANCED_FACE('',(#1480),#992,.F.) ;
#9417=ADVANCED_FACE('',(#1481),#993,.F.) ;
#9418=ADVANCED_FACE('',(#1482),#994,.F.) ;
#9419=ADVANCED_FACE('',(#1483),#995,.F.) ;
#9420=ADVANCED_FACE('',(#1484),#996,.F.) ;
#9421=ADVANCED_FACE('',(#1485),#997,.F.) ;
#9422=ADVANCED_FACE('',(#1486),#998,.F.) ;
#9423=ADVANCED_FACE('',(#1487),#999,.F.) ;
#9424=ADVANCED_FACE('',(#1488),#1000,.F.) ;
#9425=ADVANCED_FACE('',(#1489),#1001,.F.) ;
#9426=ADVANCED_FACE('',(#1490),#1002,.F.) ;
#9427=ADVANCED_FACE('',(#1491),#1003,.F.) ;
#9428=ADVANCED_FACE('',(#1492),#1004,.F.) ;
#9429=ADVANCED_FACE('',(#1493),#1005,.F.) ;
#9430=ADVANCED_FACE('',(#1494),#1006,.F.) ;
#9431=ADVANCED_FACE('',(#1495),#1007,.F.) ;
#9432=ADVANCED_FACE('',(#1496),#1008,.F.) ;
#9433=ADVANCED_FACE('',(#1497),#1009,.F.) ;
#9434=ADVANCED_FACE('',(#1498),#1010,.F.) ;
#9435=ADVANCED_FACE('',(#1499),#1011,.F.) ;
#9436=ADVANCED_FACE('',(#1500),#1012,.F.) ;
#9437=ADVANCED_FACE('',(#1501),#1013,.F.) ;
#9438=ADVANCED_FACE('',(#1502),#1014,.F.) ;
#9439=ADVANCED_FACE('',(#1503),#1015,.F.) ;
#9440=ADVANCED_FACE('',(#1504),#1016,.F.) ;
#9441=ADVANCED_FACE('',(#1505),#1017,.F.) ;
#9442=ADVANCED_FACE('',(#1506),#1018,.F.) ;
#9443=ADVANCED_FACE('',(#1507),#1019,.F.) ;
#9444=ADVANCED_FACE('',(#1508),#1020,.F.) ;
#9445=ADVANCED_FACE('',(#1509),#1021,.F.) ;
#9446=ADVANCED_FACE('',(#1510),#1022,.F.) ;
#9447=ADVANCED_FACE('',(#1511),#1023,.F.) ;
#9448=ADVANCED_FACE('',(#1512),#1024,.F.) ;
#9449=ADVANCED_FACE('',(#1513),#1025,.F.) ;
#9450=ADVANCED_FACE('',(#1514),#1026,.F.) ;
#9451=ADVANCED_FACE('',(#1515),#1027,.F.) ;
#9452=ADVANCED_FACE('',(#1516),#1028,.F.) ;
#9453=ADVANCED_FACE('',(#1517),#1029,.F.) ;
#9454=ADVANCED_FACE('',(#1518),#1030,.F.) ;
#9455=ADVANCED_FACE('',(#1519),#1031,.F.) ;
#9456=ADVANCED_FACE('',(#1520),#338,.T.) ;
#9457=ADVANCED_FACE('',(#1521,#734),#1032,.F.) ;
#9458=ADVANCED_FACE('',(#1522),#9017,.F.) ;
#9459=ADVANCED_FACE('',(#1523),#627,.T.) ;
#9460=ADVANCED_FACE('',(#1524),#628,.T.) ;
#9461=ADVANCED_FACE('',(#1525),#629,.T.) ;
#9462=ADVANCED_FACE('',(#1526),#630,.T.) ;
#9463=ADVANCED_FACE('',(#1527),#631,.T.) ;
#9464=ADVANCED_FACE('',(#1528),#632,.T.) ;
#9465=ADVANCED_FACE('',(#1529),#1033,.F.) ;
#9466=ADVANCED_FACE('',(#1530),#1034,.F.) ;
#9467=ADVANCED_FACE('',(#1531),#1035,.F.) ;
#9468=ADVANCED_FACE('',(#1532),#1036,.F.) ;
#9469=ADVANCED_FACE('',(#1533),#1037,.F.) ;
#9470=ADVANCED_FACE('',(#1534),#1038,.F.) ;
#9471=ADVANCED_FACE('',(#1535),#1039,.F.) ;
#9472=ADVANCED_FACE('',(#1536),#1040,.F.) ;
#9473=ADVANCED_FACE('',(#1537),#1041,.F.) ;
#9474=ADVANCED_FACE('',(#1538),#1042,.F.) ;
#9475=ADVANCED_FACE('',(#1539),#1043,.F.) ;
#9476=ADVANCED_FACE('',(#1540),#1044,.F.) ;
#9477=ADVANCED_FACE('',(#1541),#1045,.F.) ;
#9478=ADVANCED_FACE('',(#1542),#1046,.F.) ;
#9479=ADVANCED_FACE('',(#1543),#1047,.F.) ;
#9480=ADVANCED_FACE('',(#1544),#9018,.F.) ;
#9481=ADVANCED_FACE('',(#1545),#1048,.F.) ;
#9482=ADVANCED_FACE('',(#1546),#1049,.F.) ;
#9483=ADVANCED_FACE('',(#1547),#1050,.F.) ;
#9555=CLOSED_SHELL('',(#9308,#9309,#9310,#9311,#9312,#9313,#9314,#9315,
#9316,#9317,#9318,#9319,#9320,#9321,#9322,#9323,#9324,#9325,#9326,#9327,
#9328,#9329,#9330,#9331,#9332,#9333,#9334,#9335,#9336,#9337,#9338,#9339,
#9340,#9341,#9342,#9343,#9344,#9345,#9346,#9347,#9348,#9349,#9350,#9351,
#9352,#9353,#9354,#9355,#9356,#9357,#9358,#9359,#9360,#9361,#9362,#9363,
#9364,#9365,#9366,#9367,#9368,#9369,#9370,#9371,#9372,#9373,#9374,#9375,
#9376,#9377,#9378,#9379,#9380,#9381,#9382,#9383,#9384,#9385,#9386,#9387,
#9388,#9389,#9390,#9391,#9392,#9393,#9394,#9395,#9396,#9397,#9398,#9399,
#9400,#9401,#9402,#9403,#9404,#9405,#9406,#9407,#9408,#9409,#9410,#9411,
#9412,#9413,#9414,#9415,#9416,#9417,#9418,#9419,#9420,#9421,#9422,#9423,
#9424,#9425,#9426,#9427,#9428,#9429,#9430,#9431,#9432,#9433,#9434,#9435,
#9436,#9437,#9438,#9439,#9440,#9441,#9442,#9443,#9444,#9445,#9446,#9447,
#9448,#9449,#9450,#9451,#9452,#9453,#9454,#9455,#9456,#9457,#9458,#9459,
#9460,#9461,#9462,#9463,#9464,#9465,#9466,#9467,#9468,#9469,#9470,#9471,
#9472,#9473,#9474,#9475,#9476,#9477,#9478,#9479,#9480,#9481,#9482,#9483)) ;
#10270=AXIS2_PLACEMENT_3D('',#15298,#12199,#12200) ;
#10271=AXIS2_PLACEMENT_3D('',#15299,#12201,#12202) ;
#10272=AXIS2_PLACEMENT_3D('',#15315,#12204,#12205) ;
#10273=AXIS2_PLACEMENT_3D('',#15323,#12206,#12207) ;
#10274=AXIS2_PLACEMENT_3D('',#15371,#12209,#12210) ;
#10275=AXIS2_PLACEMENT_3D('',#15419,#12212,#12213) ;
#10276=AXIS2_PLACEMENT_3D('',#15473,#12215,#12216) ;
#10277=AXIS2_PLACEMENT_3D('',#15521,#12218,#12219) ;
#10278=AXIS2_PLACEMENT_3D('',#15569,#12221,#12222) ;
#10279=AXIS2_PLACEMENT_3D('',#15623,#12224,#12225) ;
#10280=AXIS2_PLACEMENT_3D('',#15671,#12227,#12228) ;
#10281=AXIS2_PLACEMENT_3D('',#15719,#12230,#12231) ;
#10282=AXIS2_PLACEMENT_3D('',#15773,#12233,#12234) ;
#10283=AXIS2_PLACEMENT_3D('',#15821,#12236,#12237) ;
#10284=AXIS2_PLACEMENT_3D('',#15869,#12239,#12240) ;
#10285=AXIS2_PLACEMENT_3D('',#15923,#12242,#12243) ;
#10286=AXIS2_PLACEMENT_3D('',#15971,#12245,#12246) ;
#10287=AXIS2_PLACEMENT_3D('',#15982,#12248,#12249) ;
#10288=AXIS2_PLACEMENT_3D('',#15987,#12250,#12251) ;
#10289=AXIS2_PLACEMENT_3D('',#16011,#12253,#12254) ;
#10290=AXIS2_PLACEMENT_3D('',#16036,#12256,#12257) ;
#10291=AXIS2_PLACEMENT_3D('',#16061,#12259,#12260) ;
#10292=AXIS2_PLACEMENT_3D('',#16085,#12262,#12263) ;
#10293=AXIS2_PLACEMENT_3D('',#16110,#12265,#12266) ;
#10294=AXIS2_PLACEMENT_3D('',#16135,#12268,#12269) ;
#10295=AXIS2_PLACEMENT_3D('',#16159,#12271,#12272) ;
#10296=AXIS2_PLACEMENT_3D('',#16184,#12274,#12275) ;
#10297=AXIS2_PLACEMENT_3D('',#16209,#12277,#12278) ;
#10298=AXIS2_PLACEMENT_3D('',#16233,#12280,#12281) ;
#10299=AXIS2_PLACEMENT_3D('',#16258,#12283,#12284) ;
#10300=AXIS2_PLACEMENT_3D('',#16283,#12286,#12287) ;
#10301=AXIS2_PLACEMENT_3D('',#16307,#12289,#12290) ;
#10302=AXIS2_PLACEMENT_3D('',#16383,#12291,#12292) ;
#10303=AXIS2_PLACEMENT_3D('',#16385,#12293,#12294) ;
#10304=AXIS2_PLACEMENT_3D('',#16933,#12295,#12296) ;
#10305=AXIS2_PLACEMENT_3D('',#16935,#12297,#12298) ;
#10306=AXIS2_PLACEMENT_3D('',#17013,#12299,#12300) ;
#10307=AXIS2_PLACEMENT_3D('',#17014,#12301,#12302) ;
#10308=AXIS2_PLACEMENT_3D('',#17015,#12303,#12304) ;
#10309=AXIS2_PLACEMENT_3D('',#17409,#12305,#12306) ;
#10310=AXIS2_PLACEMENT_3D('',#17411,#12307,#12308) ;
#10311=AXIS2_PLACEMENT_3D('',#17412,#12309,#12310) ;
#10312=AXIS2_PLACEMENT_3D('',#17413,#12311,#12312) ;
#10313=AXIS2_PLACEMENT_3D('',#17414,#12313,#12314) ;
#10314=AXIS2_PLACEMENT_3D('',#17415,#12315,#12316) ;
#10315=AXIS2_PLACEMENT_3D('',#17417,#12317,#12318) ;
#10316=AXIS2_PLACEMENT_3D('',#17418,#12319,#12320) ;
#10317=AXIS2_PLACEMENT_3D('',#17421,#12322,#12323) ;
#10318=AXIS2_PLACEMENT_3D('',#17422,#12324,#12325) ;
#10319=AXIS2_PLACEMENT_3D('',#17423,#12326,#12327) ;
#10320=AXIS2_PLACEMENT_3D('',#17426,#12328,#12329) ;
#10321=AXIS2_PLACEMENT_3D('',#17430,#12332,#12333) ;
#10322=AXIS2_PLACEMENT_3D('',#17438,#12336,#12337) ;
#10323=AXIS2_PLACEMENT_3D('',#17444,#12339,#12340) ;
#10324=AXIS2_PLACEMENT_3D('',#17446,#12341,#12342) ;
#10325=AXIS2_PLACEMENT_3D('',#17450,#12344,#12345) ;
#10326=AXIS2_PLACEMENT_3D('',#17454,#12347,#12348) ;
#10327=AXIS2_PLACEMENT_3D('',#17458,#12350,#12351) ;
#10328=AXIS2_PLACEMENT_3D('',#17462,#12353,#12354) ;
#10329=AXIS2_PLACEMENT_3D('',#17466,#12356,#12357) ;
#10330=AXIS2_PLACEMENT_3D('',#17470,#12359,#12360) ;
#10331=AXIS2_PLACEMENT_3D('',#17474,#12362,#12363) ;
#10332=AXIS2_PLACEMENT_3D('',#17478,#12365,#12366) ;
#10333=AXIS2_PLACEMENT_3D('',#17482,#12368,#12369) ;
#10334=AXIS2_PLACEMENT_3D('',#17486,#12371,#12372) ;
#10335=AXIS2_PLACEMENT_3D('',#17490,#12374,#12375) ;
#10336=AXIS2_PLACEMENT_3D('',#17494,#12377,#12378) ;
#10337=AXIS2_PLACEMENT_3D('',#17498,#12380,#12381) ;
#10338=AXIS2_PLACEMENT_3D('',#17502,#12383,#12384) ;
#10339=AXIS2_PLACEMENT_3D('',#17506,#12386,#12387) ;
#10340=AXIS2_PLACEMENT_3D('',#17510,#12389,#12390) ;
#10341=AXIS2_PLACEMENT_3D('',#17514,#12392,#12393) ;
#10342=AXIS2_PLACEMENT_3D('',#17518,#12395,#12396) ;
#10343=AXIS2_PLACEMENT_3D('',#17522,#12398,#12399) ;
#10344=AXIS2_PLACEMENT_3D('',#17526,#12401,#12402) ;
#10345=AXIS2_PLACEMENT_3D('',#17530,#12404,#12405) ;
#10346=AXIS2_PLACEMENT_3D('',#17534,#12407,#12408) ;
#10347=AXIS2_PLACEMENT_3D('',#17538,#12410,#12411) ;
#10348=AXIS2_PLACEMENT_3D('',#17542,#12413,#12414) ;
#10349=AXIS2_PLACEMENT_3D('',#17546,#12416,#12417) ;
#10350=AXIS2_PLACEMENT_3D('',#17550,#12419,#12420) ;
#10351=AXIS2_PLACEMENT_3D('',#17554,#12422,#12423) ;
#10352=AXIS2_PLACEMENT_3D('',#17558,#12425,#12426) ;
#10353=AXIS2_PLACEMENT_3D('',#17562,#12428,#12429) ;
#10354=AXIS2_PLACEMENT_3D('',#17566,#12431,#12432) ;
#10355=AXIS2_PLACEMENT_3D('',#17570,#12434,#12435) ;
#10356=AXIS2_PLACEMENT_3D('',#17574,#12437,#12438) ;
#10357=AXIS2_PLACEMENT_3D('',#17578,#12440,#12441) ;
#10358=AXIS2_PLACEMENT_3D('',#17582,#12443,#12444) ;
#10359=AXIS2_PLACEMENT_3D('',#17586,#12446,#12447) ;
#10360=AXIS2_PLACEMENT_3D('',#17590,#12449,#12450) ;
#10361=AXIS2_PLACEMENT_3D('',#17594,#12452,#12453) ;
#10362=AXIS2_PLACEMENT_3D('',#17597,#12455,#12456) ;
#10363=AXIS2_PLACEMENT_3D('',#17599,#12457,#12458) ;
#10364=AXIS2_PLACEMENT_3D('',#17603,#12460,#12461) ;
#10365=AXIS2_PLACEMENT_3D('',#17607,#12463,#12464) ;
#10366=AXIS2_PLACEMENT_3D('',#17611,#12466,#12467) ;
#10367=AXIS2_PLACEMENT_3D('',#17615,#12469,#12470) ;
#10368=AXIS2_PLACEMENT_3D('',#17619,#12472,#12473) ;
#10369=AXIS2_PLACEMENT_3D('',#17623,#12475,#12476) ;
#10370=AXIS2_PLACEMENT_3D('',#17627,#12478,#12479) ;
#10371=AXIS2_PLACEMENT_3D('',#17631,#12481,#12482) ;
#10372=AXIS2_PLACEMENT_3D('',#17635,#12484,#12485) ;
#10373=AXIS2_PLACEMENT_3D('',#17639,#12487,#12488) ;
#10374=AXIS2_PLACEMENT_3D('',#17643,#12490,#12491) ;
#10375=AXIS2_PLACEMENT_3D('',#17647,#12493,#12494) ;
#10376=AXIS2_PLACEMENT_3D('',#17651,#12496,#12497) ;
#10377=AXIS2_PLACEMENT_3D('',#17655,#12499,#12500) ;
#10378=AXIS2_PLACEMENT_3D('',#17659,#12502,#12503) ;
#10379=AXIS2_PLACEMENT_3D('',#17663,#12505,#12506) ;
#10380=AXIS2_PLACEMENT_3D('',#17667,#12508,#12509) ;
#10381=AXIS2_PLACEMENT_3D('',#17671,#12511,#12512) ;
#10382=AXIS2_PLACEMENT_3D('',#17675,#12514,#12515) ;
#10383=AXIS2_PLACEMENT_3D('',#17679,#12517,#12518) ;
#10384=AXIS2_PLACEMENT_3D('',#17683,#12520,#12521) ;
#10385=AXIS2_PLACEMENT_3D('',#17687,#12523,#12524) ;
#10386=AXIS2_PLACEMENT_3D('',#17691,#12526,#12527) ;
#10387=AXIS2_PLACEMENT_3D('',#17695,#12529,#12530) ;
#10388=AXIS2_PLACEMENT_3D('',#17699,#12532,#12533) ;
#10389=AXIS2_PLACEMENT_3D('',#17703,#12535,#12536) ;
#10390=AXIS2_PLACEMENT_3D('',#17707,#12538,#12539) ;
#10391=AXIS2_PLACEMENT_3D('',#17711,#12541,#12542) ;
#10392=AXIS2_PLACEMENT_3D('',#17715,#12544,#12545) ;
#10393=AXIS2_PLACEMENT_3D('',#17719,#12547,#12548) ;
#10394=AXIS2_PLACEMENT_3D('',#17723,#12550,#12551) ;
#10395=AXIS2_PLACEMENT_3D('',#17727,#12553,#12554) ;
#10396=AXIS2_PLACEMENT_3D('',#17730,#12556,#12557) ;
#10397=AXIS2_PLACEMENT_3D('',#17731,#12558,#12559) ;
#10398=AXIS2_PLACEMENT_3D('',#17739,#12562,#12563) ;
#10399=AXIS2_PLACEMENT_3D('',#17744,#12565,#12566) ;
#10400=AXIS2_PLACEMENT_3D('',#17745,#12567,#12568) ;
#10401=AXIS2_PLACEMENT_3D('',#17747,#12569,#12570) ;
#10402=AXIS2_PLACEMENT_3D('',#17987,#12572,#12573) ;
#10403=AXIS2_PLACEMENT_3D('',#17991,#12576,#12577) ;
#10404=AXIS2_PLACEMENT_3D('',#17993,#12579,#12580) ;
#10405=AXIS2_PLACEMENT_3D('',#17994,#12581,#12582) ;
#10406=AXIS2_PLACEMENT_3D('',#17998,#12585,#12586) ;
#10407=AXIS2_PLACEMENT_3D('',#18000,#12588,#12589) ;
#10408=AXIS2_PLACEMENT_3D('',#18001,#12590,#12591) ;
#10409=AXIS2_PLACEMENT_3D('',#18005,#12594,#12595) ;
#10410=AXIS2_PLACEMENT_3D('',#18007,#12597,#12598) ;
#10411=AXIS2_PLACEMENT_3D('',#18008,#12599,#12600) ;
#10412=AXIS2_PLACEMENT_3D('',#18012,#12603,#12604) ;
#10413=AXIS2_PLACEMENT_3D('',#18014,#12606,#12607) ;
#10414=AXIS2_PLACEMENT_3D('',#18015,#12608,#12609) ;
#10415=AXIS2_PLACEMENT_3D('',#18019,#12612,#12613) ;
#10416=AXIS2_PLACEMENT_3D('',#18021,#12615,#12616) ;
#10417=AXIS2_PLACEMENT_3D('',#18022,#12617,#12618) ;
#10418=AXIS2_PLACEMENT_3D('',#18026,#12621,#12622) ;
#10419=AXIS2_PLACEMENT_3D('',#18028,#12624,#12625) ;
#10420=AXIS2_PLACEMENT_3D('',#18029,#12626,#12627) ;
#10421=AXIS2_PLACEMENT_3D('',#18033,#12630,#12631) ;
#10422=AXIS2_PLACEMENT_3D('',#18035,#12633,#12634) ;
#10423=AXIS2_PLACEMENT_3D('',#18036,#12635,#12636) ;
#10424=AXIS2_PLACEMENT_3D('',#18040,#12639,#12640) ;
#10425=AXIS2_PLACEMENT_3D('',#18042,#12642,#12643) ;
#10426=AXIS2_PLACEMENT_3D('',#18043,#12644,#12645) ;
#10427=AXIS2_PLACEMENT_3D('',#18047,#12648,#12649) ;
#10428=AXIS2_PLACEMENT_3D('',#18049,#12651,#12652) ;
#10429=AXIS2_PLACEMENT_3D('',#18050,#12653,#12654) ;
#10430=AXIS2_PLACEMENT_3D('',#18054,#12657,#12658) ;
#10431=AXIS2_PLACEMENT_3D('',#18056,#12660,#12661) ;
#10432=AXIS2_PLACEMENT_3D('',#18057,#12662,#12663) ;
#10433=AXIS2_PLACEMENT_3D('',#18061,#12666,#12667) ;
#10434=AXIS2_PLACEMENT_3D('',#18063,#12669,#12670) ;
#10435=AXIS2_PLACEMENT_3D('',#18064,#12671,#12672) ;
#10436=AXIS2_PLACEMENT_3D('',#18068,#12675,#12676) ;
#10437=AXIS2_PLACEMENT_3D('',#18070,#12678,#12679) ;
#10438=AXIS2_PLACEMENT_3D('',#18071,#12680,#12681) ;
#10439=AXIS2_PLACEMENT_3D('',#18075,#12684,#12685) ;
#10440=AXIS2_PLACEMENT_3D('',#18077,#12687,#12688) ;
#10441=AXIS2_PLACEMENT_3D('',#18078,#12689,#12690) ;
#10442=AXIS2_PLACEMENT_3D('',#18082,#12693,#12694) ;
#10443=AXIS2_PLACEMENT_3D('',#18084,#12696,#12697) ;
#10444=AXIS2_PLACEMENT_3D('',#18085,#12698,#12699) ;
#10445=AXIS2_PLACEMENT_3D('',#18089,#12702,#12703) ;
#10446=AXIS2_PLACEMENT_3D('',#18091,#12705,#12706) ;
#10447=AXIS2_PLACEMENT_3D('',#18092,#12707,#12708) ;
#10448=AXIS2_PLACEMENT_3D('',#18096,#12711,#12712) ;
#10449=AXIS2_PLACEMENT_3D('',#18098,#12714,#12715) ;
#10450=AXIS2_PLACEMENT_3D('',#18099,#12716,#12717) ;
#10451=AXIS2_PLACEMENT_3D('',#18103,#12720,#12721) ;
#10452=AXIS2_PLACEMENT_3D('',#18105,#12723,#12724) ;
#10453=AXIS2_PLACEMENT_3D('',#18106,#12725,#12726) ;
#10454=AXIS2_PLACEMENT_3D('',#18110,#12729,#12730) ;
#10455=AXIS2_PLACEMENT_3D('',#18112,#12732,#12733) ;
#10456=AXIS2_PLACEMENT_3D('',#18113,#12734,#12735) ;
#10457=AXIS2_PLACEMENT_3D('',#18117,#12738,#12739) ;
#10458=AXIS2_PLACEMENT_3D('',#18119,#12741,#12742) ;
#10459=AXIS2_PLACEMENT_3D('',#18120,#12743,#12744) ;
#10460=AXIS2_PLACEMENT_3D('',#18124,#12747,#12748) ;
#10461=AXIS2_PLACEMENT_3D('',#18126,#12750,#12751) ;
#10462=AXIS2_PLACEMENT_3D('',#18127,#12752,#12753) ;
#10463=AXIS2_PLACEMENT_3D('',#18131,#12756,#12757) ;
#10464=AXIS2_PLACEMENT_3D('',#18133,#12759,#12760) ;
#10465=AXIS2_PLACEMENT_3D('',#18134,#12761,#12762) ;
#10466=AXIS2_PLACEMENT_3D('',#18138,#12765,#12766) ;
#10467=AXIS2_PLACEMENT_3D('',#18140,#12768,#12769) ;
#10468=AXIS2_PLACEMENT_3D('',#18141,#12770,#12771) ;
#10469=AXIS2_PLACEMENT_3D('',#18145,#12774,#12775) ;
#10470=AXIS2_PLACEMENT_3D('',#18147,#12777,#12778) ;
#10471=AXIS2_PLACEMENT_3D('',#18148,#12779,#12780) ;
#10472=AXIS2_PLACEMENT_3D('',#18152,#12783,#12784) ;
#10473=AXIS2_PLACEMENT_3D('',#18154,#12786,#12787) ;
#10474=AXIS2_PLACEMENT_3D('',#18155,#12788,#12789) ;
#10475=AXIS2_PLACEMENT_3D('',#18159,#12792,#12793) ;
#10476=AXIS2_PLACEMENT_3D('',#18161,#12795,#12796) ;
#10477=AXIS2_PLACEMENT_3D('',#18162,#12797,#12798) ;
#10478=AXIS2_PLACEMENT_3D('',#18166,#12801,#12802) ;
#10479=AXIS2_PLACEMENT_3D('',#18168,#12804,#12805) ;
#10480=AXIS2_PLACEMENT_3D('',#18169,#12806,#12807) ;
#10481=AXIS2_PLACEMENT_3D('',#18173,#12810,#12811) ;
#10482=AXIS2_PLACEMENT_3D('',#18175,#12813,#12814) ;
#10483=AXIS2_PLACEMENT_3D('',#18176,#12815,#12816) ;
#10484=AXIS2_PLACEMENT_3D('',#18180,#12819,#12820) ;
#10485=AXIS2_PLACEMENT_3D('',#18182,#12822,#12823) ;
#10486=AXIS2_PLACEMENT_3D('',#18183,#12824,#12825) ;
#10487=AXIS2_PLACEMENT_3D('',#18187,#12828,#12829) ;
#10488=AXIS2_PLACEMENT_3D('',#18189,#12831,#12832) ;
#10489=AXIS2_PLACEMENT_3D('',#18190,#12833,#12834) ;
#10490=AXIS2_PLACEMENT_3D('',#18194,#12837,#12838) ;
#10491=AXIS2_PLACEMENT_3D('',#18196,#12840,#12841) ;
#10492=AXIS2_PLACEMENT_3D('',#18197,#12842,#12843) ;
#10493=AXIS2_PLACEMENT_3D('',#18201,#12846,#12847) ;
#10494=AXIS2_PLACEMENT_3D('',#18203,#12849,#12850) ;
#10495=AXIS2_PLACEMENT_3D('',#18204,#12851,#12852) ;
#10496=AXIS2_PLACEMENT_3D('',#18208,#12855,#12856) ;
#10497=AXIS2_PLACEMENT_3D('',#18210,#12858,#12859) ;
#10498=AXIS2_PLACEMENT_3D('',#18211,#12860,#12861) ;
#10499=AXIS2_PLACEMENT_3D('',#18215,#12864,#12865) ;
#10500=AXIS2_PLACEMENT_3D('',#18217,#12867,#12868) ;
#10501=AXIS2_PLACEMENT_3D('',#18218,#12869,#12870) ;
#10502=AXIS2_PLACEMENT_3D('',#18222,#12873,#12874) ;
#10503=AXIS2_PLACEMENT_3D('',#18224,#12876,#12877) ;
#10504=AXIS2_PLACEMENT_3D('',#18225,#12878,#12879) ;
#10505=AXIS2_PLACEMENT_3D('',#18226,#12880,#12881) ;
#10506=AXIS2_PLACEMENT_3D('',#18227,#12882,#12883) ;
#10507=AXIS2_PLACEMENT_3D('',#18229,#12884,#12885) ;
#10508=AXIS2_PLACEMENT_3D('',#18230,#12886,#12887) ;
#10509=AXIS2_PLACEMENT_3D('',#18238,#12889,#12890) ;
#10510=AXIS2_PLACEMENT_3D('',#18248,#12891,#12892) ;
#10511=AXIS2_PLACEMENT_3D('',#18258,#12893,#12894) ;
#10512=AXIS2_PLACEMENT_3D('',#18268,#12895,#12896) ;
#10513=AXIS2_PLACEMENT_3D('',#18278,#12897,#12898) ;
#10514=AXIS2_PLACEMENT_3D('',#18288,#12899,#12900) ;
#10515=AXIS2_PLACEMENT_3D('',#18292,#12901,#12902) ;
#10516=AXIS2_PLACEMENT_3D('',#18297,#12905,#12906) ;
#10517=AXIS2_PLACEMENT_3D('',#18298,#12907,#12908) ;
#10518=AXIS2_PLACEMENT_3D('',#18303,#12911,#12912) ;
#10519=AXIS2_PLACEMENT_3D('',#18304,#12913,#12914) ;
#10520=AXIS2_PLACEMENT_3D('',#18308,#12916,#12917) ;
#10521=AXIS2_PLACEMENT_3D('',#18310,#12919,#12920) ;
#10522=AXIS2_PLACEMENT_3D('',#18315,#12923,#12924) ;
#10523=AXIS2_PLACEMENT_3D('',#18316,#12925,#12926) ;
#10524=AXIS2_PLACEMENT_3D('',#18320,#12928,#12929) ;
#10525=AXIS2_PLACEMENT_3D('',#18322,#12931,#12932) ;
#10526=AXIS2_PLACEMENT_3D('',#18326,#12934,#12935) ;
#10527=AXIS2_PLACEMENT_3D('',#18328,#12937,#12938) ;
#10528=AXIS2_PLACEMENT_3D('',#18335,#12943,#12944) ;
#10529=AXIS2_PLACEMENT_3D('',#18340,#12948,#12949) ;
#10530=AXIS2_PLACEMENT_3D('',#18345,#12953,#12954) ;
#10531=AXIS2_PLACEMENT_3D('',#18346,#12955,#12956) ;
#10532=AXIS2_PLACEMENT_3D('',#18347,#12957,#12958) ;
#10533=AXIS2_PLACEMENT_3D('',#18349,#12960,#12961) ;
#10534=AXIS2_PLACEMENT_3D('',#18350,#12962,#12963) ;
#10535=AXIS2_PLACEMENT_3D('',#18352,#12965,#12966) ;
#10536=AXIS2_PLACEMENT_3D('',#18354,#12968,#12969) ;
#10537=AXIS2_PLACEMENT_3D('',#18357,#12971,#12972) ;
#10538=AXIS2_PLACEMENT_3D('',#18358,#12973,#12974) ;
#10539=AXIS2_PLACEMENT_3D('',#18359,#12975,#12976) ;
#10540=AXIS2_PLACEMENT_3D('',#18360,#12977,#12978) ;
#10541=AXIS2_PLACEMENT_3D('',#18361,#12979,#12980) ;
#10542=AXIS2_PLACEMENT_3D('',#18362,#12981,#12982) ;
#10543=AXIS2_PLACEMENT_3D('',#18363,#12983,#12984) ;
#10544=AXIS2_PLACEMENT_3D('',#18364,#12985,#12986) ;
#10545=AXIS2_PLACEMENT_3D('',#18367,#12988,#12989) ;
#10546=AXIS2_PLACEMENT_3D('',#18368,#12990,#12991) ;
#10547=AXIS2_PLACEMENT_3D('',#18370,#12993,#12994) ;
#10548=AXIS2_PLACEMENT_3D('',#18371,#12995,#12996) ;
#10549=AXIS2_PLACEMENT_3D('',#18374,#12998,#12999) ;
#10550=AXIS2_PLACEMENT_3D('',#18376,#13001,#13002) ;
#10551=AXIS2_PLACEMENT_3D('',#18378,#13004,#13005) ;
#12199=DIRECTION('axis',(0.,0.,1.)) ;
#12200=DIRECTION('refdir',(1.,0.,0.)) ;
#12201=DIRECTION('center_axis',(0.,0.,1.)) ;
#12202=DIRECTION('ref_axis',(1.,0.,0.)) ;
#12203=DIRECTION('',(0.,0.,-1.)) ;
#12204=DIRECTION('center_axis',(0.,0.,-1.)) ;
#12205=DIRECTION('ref_axis',(1.,0.,0.)) ;
#12206=DIRECTION('center_axis',(0.,0.,1.)) ;
#12207=DIRECTION('ref_axis',(1.,0.,0.)) ;
#12208=DIRECTION('',(0.,0.,-1.)) ;
#12209=DIRECTION('center_axis',(0.,0.,1.)) ;
#12210=DIRECTION('ref_axis',(1.,0.,0.)) ;
#12211=DIRECTION('',(0.,0.,-1.)) ;
#12212=DIRECTION('center_axis',(0.,0.,1.)) ;
#12213=DIRECTION('ref_axis',(1.,0.,0.)) ;
#12214=DIRECTION('',(0.,0.,-1.)) ;
#12215=DIRECTION('center_axis',(0.,0.,1.)) ;
#12216=DIRECTION('ref_axis',(1.,0.,0.)) ;
#12217=DIRECTION('',(0.,0.,-1.)) ;
#12218=DIRECTION('center_axis',(0.,0.,1.)) ;
#12219=DIRECTION('ref_axis',(1.,0.,0.)) ;
#12220=DIRECTION('',(0.,0.,-1.)) ;
#12221=DIRECTION('center_axis',(0.,0.,1.)) ;
#12222=DIRECTION('ref_axis',(1.,0.,0.)) ;
#12223=DIRECTION('',(0.,0.,-1.)) ;
#12224=DIRECTION('center_axis',(0.,0.,1.)) ;
#12225=DIRECTION('ref_axis',(1.,0.,0.)) ;
#12226=DIRECTION('',(0.,0.,-1.)) ;
#12227=DIRECTION('center_axis',(0.,0.,1.)) ;
#12228=DIRECTION('ref_axis',(1.,0.,0.)) ;
#12229=DIRECTION('',(0.,0.,-1.)) ;
#12230=DIRECTION('center_axis',(0.,0.,1.)) ;
#12231=DIRECTION('ref_axis',(1.,0.,0.)) ;
#12232=DIRECTION('',(0.,0.,-1.)) ;
#12233=DIRECTION('center_axis',(0.,0.,1.)) ;
#12234=DIRECTION('ref_axis',(1.,0.,0.)) ;
#12235=DIRECTION('',(0.,0.,-1.)) ;
#12236=DIRECTION('center_axis',(0.,0.,1.)) ;
#12237=DIRECTION('ref_axis',(1.,0.,0.)) ;
#12238=DIRECTION('',(0.,0.,-1.)) ;
#12239=DIRECTION('center_axis',(0.,0.,1.)) ;
#12240=DIRECTION('ref_axis',(1.,0.,0.)) ;
#12241=DIRECTION('',(0.,0.,-1.)) ;
#12242=DIRECTION('center_axis',(0.,0.,1.)) ;
#12243=DIRECTION('ref_axis',(1.,0.,0.)) ;
#12244=DIRECTION('',(0.,0.,-1.)) ;
#12245=DIRECTION('center_axis',(0.,0.,1.)) ;
#12246=DIRECTION('ref_axis',(-0.762712670465396,-0.646737491036004,0.)) ;
#12247=DIRECTION('',(0.,0.,1.)) ;
#12248=DIRECTION('center_axis',(0.,0.,1.)) ;
#12249=DIRECTION('ref_axis',(1.,1.08167872493926E-13,0.)) ;
#12250=DIRECTION('center_axis',(0.,0.,1.)) ;
#12251=DIRECTION('ref_axis',(1.,1.08167872493926E-13,0.)) ;
#12252=DIRECTION('',(0.,0.,1.)) ;
#12253=DIRECTION('center_axis',(0.,0.,1.)) ;
#12254=DIRECTION('ref_axis',(1.,1.08167872493926E-13,0.)) ;
#12255=DIRECTION('',(0.,0.,1.)) ;
#12256=DIRECTION('center_axis',(0.,0.,1.)) ;
#12257=DIRECTION('ref_axis',(1.,1.08167872493926E-13,0.)) ;
#12258=DIRECTION('',(0.,0.,1.)) ;
#12259=DIRECTION('center_axis',(0.,0.,1.)) ;
#12260=DIRECTION('ref_axis',(1.,1.08167872493926E-13,0.)) ;
#12261=DIRECTION('',(0.,0.,1.)) ;
#12262=DIRECTION('center_axis',(0.,0.,1.)) ;
#12263=DIRECTION('ref_axis',(1.,1.08167872493926E-13,0.)) ;
#12264=DIRECTION('',(0.,0.,1.)) ;
#12265=DIRECTION('center_axis',(0.,0.,1.)) ;
#12266=DIRECTION('ref_axis',(1.,1.08167872493926E-13,0.)) ;
#12267=DIRECTION('',(0.,0.,1.)) ;
#12268=DIRECTION('center_axis',(0.,0.,1.)) ;
#12269=DIRECTION('ref_axis',(1.,1.08167872493926E-13,0.)) ;
#12270=DIRECTION('',(0.,0.,1.)) ;
#12271=DIRECTION('center_axis',(0.,0.,1.)) ;
#12272=DIRECTION('ref_axis',(1.,1.08167872493926E-13,0.)) ;
#12273=DIRECTION('',(0.,0.,1.)) ;
#12274=DIRECTION('center_axis',(0.,0.,1.)) ;
#12275=DIRECTION('ref_axis',(1.,1.08167872493926E-13,0.)) ;
#12276=DIRECTION('',(0.,0.,1.)) ;
#12277=DIRECTION('center_axis',(0.,0.,1.)) ;
#12278=DIRECTION('ref_axis',(1.,1.08167872493926E-13,0.)) ;
#12279=DIRECTION('',(0.,0.,1.)) ;
#12280=DIRECTION('center_axis',(0.,0.,1.)) ;
#12281=DIRECTION('ref_axis',(1.,1.08167872493926E-13,0.)) ;
#12282=DIRECTION('',(0.,0.,1.)) ;
#12283=DIRECTION('center_axis',(0.,0.,1.)) ;
#12284=DIRECTION('ref_axis',(1.,1.08167872493926E-13,0.)) ;
#12285=DIRECTION('',(0.,0.,1.)) ;
#12286=DIRECTION('center_axis',(0.,0.,1.)) ;
#12287=DIRECTION('ref_axis',(1.,1.08167872493926E-13,0.)) ;
#12288=DIRECTION('',(0.,0.,1.)) ;
#12289=DIRECTION('center_axis',(0.,0.,1.)) ;
#12290=DIRECTION('ref_axis',(1.,0.,0.)) ;
#12291=DIRECTION('center_axis',(0.,0.,1.)) ;
#12292=DIRECTION('ref_axis',(1.,0.,0.)) ;
#12293=DIRECTION('center_axis',(0.,0.,1.)) ;
#12294=DIRECTION('ref_axis',(1.,0.,0.)) ;
#12295=DIRECTION('center_axis',(0.,0.,1.)) ;
#12296=DIRECTION('ref_axis',(1.,0.,0.)) ;
#12297=DIRECTION('center_axis',(0.,0.,-1.)) ;
#12298=DIRECTION('ref_axis',(1.,0.,0.)) ;
#12299=DIRECTION('center_axis',(0.,0.,-1.)) ;
#12300=DIRECTION('ref_axis',(1.,1.08167872493926E-13,0.)) ;
#12301=DIRECTION('center_axis',(0.,0.,-1.)) ;
#12302=DIRECTION('ref_axis',(1.,0.,0.)) ;
#12303=DIRECTION('center_axis',(0.,0.,1.)) ;
#12304=DIRECTION('ref_axis',(1.,1.08167872493926E-13,0.)) ;
#12305=DIRECTION('center_axis',(0.,0.,-1.)) ;
#12306=DIRECTION('ref_axis',(-1.,0.,0.)) ;
#12307=DIRECTION('center_axis',(0.,-1.,0.)) ;
#12308=DIRECTION('ref_axis',(1.,0.,0.)) ;
#12309=DIRECTION('center_axis',(0.,0.,1.)) ;
#12310=DIRECTION('ref_axis',(1.,0.,0.)) ;
#12311=DIRECTION('center_axis',(0.,0.,1.)) ;
#12312=DIRECTION('ref_axis',(0.581478264894299,-0.813561938303111,0.)) ;
#12313=DIRECTION('center_axis',(0.,0.,1.)) ;
#12314=DIRECTION('ref_axis',(1.,0.,0.)) ;
#12315=DIRECTION('center_axis',(0.,0.,1.)) ;
#12316=DIRECTION('ref_axis',(1.,0.,0.)) ;
#12317=DIRECTION('center_axis',(0.,0.,-1.)) ;
#12318=DIRECTION('ref_axis',(1.,0.,0.)) ;
#12319=DIRECTION('center_axis',(0.,0.,-1.)) ;
#12320=DIRECTION('ref_axis',(1.,0.,0.)) ;
#12321=DIRECTION('',(0.707106781186547,-8.65956056235493E-17,0.707106781186547)) ;
#12322=DIRECTION('center_axis',(0.,0.,-1.)) ;
#12323=DIRECTION('ref_axis',(1.,0.,0.)) ;
#12324=DIRECTION('center_axis',(0.,0.,1.)) ;
#12325=DIRECTION('ref_axis',(1.,0.,0.)) ;
#12326=DIRECTION('center_axis',(0.,0.,1.)) ;
#12327=DIRECTION('ref_axis',(0.984807753012208,-0.17364817766693,0.)) ;
#12328=DIRECTION('center_axis',(0.,0.,1.)) ;
#12329=DIRECTION('ref_axis',(1.,0.,0.)) ;
#12330=DIRECTION('',(0.869726513699841,-0.493533981978465,0.)) ;
#12331=DIRECTION('',(-0.986074150277955,-0.166306254102512,0.)) ;
#12332=DIRECTION('center_axis',(-0.166306254102512,0.986074150277955,0.)) ;
#12333=DIRECTION('ref_axis',(-0.986074150277955,-0.166306254102512,0.)) ;
#12334=DIRECTION('',(0.,0.,-1.)) ;
#12335=DIRECTION('',(0.,0.,1.)) ;
#12336=DIRECTION('center_axis',(-0.493533981978465,-0.869726513699841,0.)) ;
#12337=DIRECTION('ref_axis',(0.869726513699841,-0.493533981978465,0.)) ;
#12338=DIRECTION('',(0.,0.,1.)) ;
#12339=DIRECTION('center_axis',(0.,0.,-1.)) ;
#12340=DIRECTION('ref_axis',(1.,0.,0.)) ;
#12341=DIRECTION('center_axis',(0.,0.,-1.)) ;
#12342=DIRECTION('ref_axis',(1.,0.,0.)) ;
#12343=DIRECTION('',(0.,0.,1.)) ;
#12344=DIRECTION('center_axis',(0.,0.,1.)) ;
#12345=DIRECTION('ref_axis',(1.,0.,0.)) ;
#12346=DIRECTION('',(0.,0.,-1.)) ;
#12347=DIRECTION('center_axis',(0.,0.,-1.)) ;
#12348=DIRECTION('ref_axis',(1.,0.,0.)) ;
#12349=DIRECTION('',(0.,0.,1.)) ;
#12350=DIRECTION('center_axis',(0.,0.,1.)) ;
#12351=DIRECTION('ref_axis',(1.,0.,0.)) ;
#12352=DIRECTION('',(0.,0.,-1.)) ;
#12353=DIRECTION('center_axis',(0.,0.,-1.)) ;
#12354=DIRECTION('ref_axis',(1.,0.,0.)) ;
#12355=DIRECTION('',(0.,0.,1.)) ;
#12356=DIRECTION('center_axis',(0.,0.,1.)) ;
#12357=DIRECTION('ref_axis',(1.,0.,0.)) ;
#12358=DIRECTION('',(0.,0.,-1.)) ;
#12359=DIRECTION('center_axis',(0.,0.,-1.)) ;
#12360=DIRECTION('ref_axis',(1.,0.,0.)) ;
#12361=DIRECTION('',(0.,0.,1.)) ;
#12362=DIRECTION('center_axis',(0.,0.,1.)) ;
#12363=DIRECTION('ref_axis',(1.,0.,0.)) ;
#12364=DIRECTION('',(0.,0.,-1.)) ;
#12365=DIRECTION('center_axis',(0.,0.,-1.)) ;
#12366=DIRECTION('ref_axis',(1.,0.,0.)) ;
#12367=DIRECTION('',(0.,0.,1.)) ;
#12368=DIRECTION('center_axis',(0.,0.,1.)) ;
#12369=DIRECTION('ref_axis',(1.,0.,0.)) ;
#12370=DIRECTION('',(0.,0.,-1.)) ;
#12371=DIRECTION('center_axis',(0.,0.,-1.)) ;
#12372=DIRECTION('ref_axis',(1.,0.,0.)) ;
#12373=DIRECTION('',(0.,0.,1.)) ;
#12374=DIRECTION('center_axis',(0.,0.,1.)) ;
#12375=DIRECTION('ref_axis',(1.,0.,0.)) ;
#12376=DIRECTION('',(0.,0.,-1.)) ;
#12377=DIRECTION('center_axis',(0.,0.,-1.)) ;
#12378=DIRECTION('ref_axis',(1.,0.,0.)) ;
#12379=DIRECTION('',(0.,0.,1.)) ;
#12380=DIRECTION('center_axis',(0.,0.,1.)) ;
#12381=DIRECTION('ref_axis',(1.,0.,0.)) ;
#12382=DIRECTION('',(0.,0.,-1.)) ;
#12383=DIRECTION('center_axis',(0.,0.,-1.)) ;
#12384=DIRECTION('ref_axis',(1.,0.,0.)) ;
#12385=DIRECTION('',(0.,0.,1.)) ;
#12386=DIRECTION('center_axis',(0.,0.,1.)) ;
#12387=DIRECTION('ref_axis',(1.,0.,0.)) ;
#12388=DIRECTION('',(0.,0.,-1.)) ;
#12389=DIRECTION('center_axis',(0.,0.,-1.)) ;
#12390=DIRECTION('ref_axis',(1.,0.,0.)) ;
#12391=DIRECTION('',(0.,0.,1.)) ;
#12392=DIRECTION('center_axis',(0.,0.,1.)) ;
#12393=DIRECTION('ref_axis',(1.,0.,0.)) ;
#12394=DIRECTION('',(0.,0.,-1.)) ;
#12395=DIRECTION('center_axis',(0.,0.,-1.)) ;
#12396=DIRECTION('ref_axis',(1.,0.,0.)) ;
#12397=DIRECTION('',(0.,0.,1.)) ;
#12398=DIRECTION('center_axis',(0.,0.,1.)) ;
#12399=DIRECTION('ref_axis',(1.,0.,0.)) ;
#12400=DIRECTION('',(0.,0.,-1.)) ;
#12401=DIRECTION('center_axis',(0.,0.,-1.)) ;
#12402=DIRECTION('ref_axis',(1.,0.,0.)) ;
#12403=DIRECTION('',(0.,0.,1.)) ;
#12404=DIRECTION('center_axis',(0.,0.,1.)) ;
#12405=DIRECTION('ref_axis',(1.,0.,0.)) ;
#12406=DIRECTION('',(0.,0.,-1.)) ;
#12407=DIRECTION('center_axis',(0.,0.,-1.)) ;
#12408=DIRECTION('ref_axis',(1.,0.,0.)) ;
#12409=DIRECTION('',(0.,0.,1.)) ;
#12410=DIRECTION('center_axis',(0.,0.,1.)) ;
#12411=DIRECTION('ref_axis',(1.,0.,0.)) ;
#12412=DIRECTION('',(0.,0.,-1.)) ;
#12413=DIRECTION('center_axis',(0.,0.,-1.)) ;
#12414=DIRECTION('ref_axis',(1.,0.,0.)) ;
#12415=DIRECTION('',(0.,0.,1.)) ;
#12416=DIRECTION('center_axis',(0.,0.,1.)) ;
#12417=DIRECTION('ref_axis',(1.,0.,0.)) ;
#12418=DIRECTION('',(0.,0.,-1.)) ;
#12419=DIRECTION('center_axis',(0.,0.,-1.)) ;
#12420=DIRECTION('ref_axis',(1.,0.,0.)) ;
#12421=DIRECTION('',(0.,0.,1.)) ;
#12422=DIRECTION('center_axis',(0.,0.,1.)) ;
#12423=DIRECTION('ref_axis',(1.,0.,0.)) ;
#12424=DIRECTION('',(0.,0.,-1.)) ;
#12425=DIRECTION('center_axis',(0.,0.,-1.)) ;
#12426=DIRECTION('ref_axis',(1.,0.,0.)) ;
#12427=DIRECTION('',(0.,0.,1.)) ;
#12428=DIRECTION('center_axis',(0.,0.,1.)) ;
#12429=DIRECTION('ref_axis',(1.,0.,0.)) ;
#12430=DIRECTION('',(0.,0.,-1.)) ;
#12431=DIRECTION('center_axis',(0.,0.,-1.)) ;
#12432=DIRECTION('ref_axis',(1.,0.,0.)) ;
#12433=DIRECTION('',(0.,0.,1.)) ;
#12434=DIRECTION('center_axis',(0.,0.,1.)) ;
#12435=DIRECTION('ref_axis',(1.,0.,0.)) ;
#12436=DIRECTION('',(0.,0.,-1.)) ;
#12437=DIRECTION('center_axis',(0.,0.,-1.)) ;
#12438=DIRECTION('ref_axis',(1.,0.,0.)) ;
#12439=DIRECTION('',(0.,0.,1.)) ;
#12440=DIRECTION('center_axis',(0.,0.,1.)) ;
#12441=DIRECTION('ref_axis',(1.,0.,0.)) ;
#12442=DIRECTION('',(0.,0.,-1.)) ;
#12443=DIRECTION('center_axis',(0.,0.,-1.)) ;
#12444=DIRECTION('ref_axis',(1.,0.,0.)) ;
#12445=DIRECTION('',(0.,0.,1.)) ;
#12446=DIRECTION('center_axis',(0.,0.,1.)) ;
#12447=DIRECTION('ref_axis',(1.,0.,0.)) ;
#12448=DIRECTION('',(0.,0.,-1.)) ;
#12449=DIRECTION('center_axis',(0.,0.,-1.)) ;
#12450=DIRECTION('ref_axis',(1.,0.,0.)) ;
#12451=DIRECTION('',(0.,0.,1.)) ;
#12452=DIRECTION('center_axis',(0.,0.,1.)) ;
#12453=DIRECTION('ref_axis',(1.,0.,0.)) ;
#12454=DIRECTION('',(0.,0.,1.)) ;
#12455=DIRECTION('center_axis',(0.,0.,1.)) ;
#12456=DIRECTION('ref_axis',(1.,0.,0.)) ;
#12457=DIRECTION('center_axis',(0.,0.,1.)) ;
#12458=DIRECTION('ref_axis',(1.,0.,0.)) ;
#12459=DIRECTION('',(0.,0.,-1.)) ;
#12460=DIRECTION('center_axis',(0.,0.,-1.)) ;
#12461=DIRECTION('ref_axis',(1.,0.,0.)) ;
#12462=DIRECTION('',(0.,0.,1.)) ;
#12463=DIRECTION('center_axis',(0.,0.,1.)) ;
#12464=DIRECTION('ref_axis',(1.,0.,0.)) ;
#12465=DIRECTION('',(0.,0.,-1.)) ;
#12466=DIRECTION('center_axis',(0.,0.,-1.)) ;
#12467=DIRECTION('ref_axis',(1.,0.,0.)) ;
#12468=DIRECTION('',(0.,0.,1.)) ;
#12469=DIRECTION('center_axis',(0.,0.,1.)) ;
#12470=DIRECTION('ref_axis',(1.,0.,0.)) ;
#12471=DIRECTION('',(0.,0.,-1.)) ;
#12472=DIRECTION('center_axis',(0.,0.,-1.)) ;
#12473=DIRECTION('ref_axis',(1.,0.,0.)) ;
#12474=DIRECTION('',(0.,0.,1.)) ;
#12475=DIRECTION('center_axis',(0.,0.,1.)) ;
#12476=DIRECTION('ref_axis',(1.,0.,0.)) ;
#12477=DIRECTION('',(0.,0.,-1.)) ;
#12478=DIRECTION('center_axis',(0.,0.,-1.)) ;
#12479=DIRECTION('ref_axis',(1.,0.,0.)) ;
#12480=DIRECTION('',(0.,0.,1.)) ;
#12481=DIRECTION('center_axis',(0.,0.,1.)) ;
#12482=DIRECTION('ref_axis',(1.,0.,0.)) ;
#12483=DIRECTION('',(0.,0.,-1.)) ;
#12484=DIRECTION('center_axis',(0.,0.,-1.)) ;
#12485=DIRECTION('ref_axis',(1.,0.,0.)) ;
#12486=DIRECTION('',(0.,0.,1.)) ;
#12487=DIRECTION('center_axis',(0.,0.,1.)) ;
#12488=DIRECTION('ref_axis',(1.,0.,0.)) ;
#12489=DIRECTION('',(0.,0.,-1.)) ;
#12490=DIRECTION('center_axis',(0.,0.,-1.)) ;
#12491=DIRECTION('ref_axis',(1.,0.,0.)) ;
#12492=DIRECTION('',(0.,0.,1.)) ;
#12493=DIRECTION('center_axis',(0.,0.,1.)) ;
#12494=DIRECTION('ref_axis',(1.,0.,0.)) ;
#12495=DIRECTION('',(0.,0.,-1.)) ;
#12496=DIRECTION('center_axis',(0.,0.,-1.)) ;
#12497=DIRECTION('ref_axis',(1.,0.,0.)) ;
#12498=DIRECTION('',(0.,0.,1.)) ;
#12499=DIRECTION('center_axis',(0.,0.,1.)) ;
#12500=DIRECTION('ref_axis',(1.,0.,0.)) ;
#12501=DIRECTION('',(0.,0.,-1.)) ;
#12502=DIRECTION('center_axis',(0.,0.,-1.)) ;
#12503=DIRECTION('ref_axis',(1.,0.,0.)) ;
#12504=DIRECTION('',(0.,0.,1.)) ;
#12505=DIRECTION('center_axis',(0.,0.,1.)) ;
#12506=DIRECTION('ref_axis',(1.,0.,0.)) ;
#12507=DIRECTION('',(0.,0.,-1.)) ;
#12508=DIRECTION('center_axis',(0.,0.,-1.)) ;
#12509=DIRECTION('ref_axis',(1.,0.,0.)) ;
#12510=DIRECTION('',(0.,0.,1.)) ;
#12511=DIRECTION('center_axis',(0.,0.,1.)) ;
#12512=DIRECTION('ref_axis',(1.,0.,0.)) ;
#12513=DIRECTION('',(0.,0.,-1.)) ;
#12514=DIRECTION('center_axis',(0.,0.,-1.)) ;
#12515=DIRECTION('ref_axis',(1.,0.,0.)) ;
#12516=DIRECTION('',(0.,0.,1.)) ;
#12517=DIRECTION('center_axis',(0.,0.,1.)) ;
#12518=DIRECTION('ref_axis',(1.,0.,0.)) ;
#12519=DIRECTION('',(0.,0.,-1.)) ;
#12520=DIRECTION('center_axis',(0.,0.,-1.)) ;
#12521=DIRECTION('ref_axis',(1.,0.,0.)) ;
#12522=DIRECTION('',(0.,0.,1.)) ;
#12523=DIRECTION('center_axis',(0.,0.,1.)) ;
#12524=DIRECTION('ref_axis',(1.,0.,0.)) ;
#12525=DIRECTION('',(0.,0.,-1.)) ;
#12526=DIRECTION('center_axis',(0.,0.,-1.)) ;
#12527=DIRECTION('ref_axis',(1.,0.,0.)) ;
#12528=DIRECTION('',(0.,0.,1.)) ;
#12529=DIRECTION('center_axis',(0.,0.,1.)) ;
#12530=DIRECTION('ref_axis',(1.,0.,0.)) ;
#12531=DIRECTION('',(0.,0.,-1.)) ;
#12532=DIRECTION('center_axis',(0.,0.,-1.)) ;
#12533=DIRECTION('ref_axis',(1.,0.,0.)) ;
#12534=DIRECTION('',(0.,0.,1.)) ;
#12535=DIRECTION('center_axis',(0.,0.,1.)) ;
#12536=DIRECTION('ref_axis',(1.,0.,0.)) ;
#12537=DIRECTION('',(0.,0.,-1.)) ;
#12538=DIRECTION('center_axis',(0.,0.,-1.)) ;
#12539=DIRECTION('ref_axis',(1.,0.,0.)) ;
#12540=DIRECTION('',(0.,0.,1.)) ;
#12541=DIRECTION('center_axis',(0.,0.,1.)) ;
#12542=DIRECTION('ref_axis',(1.,0.,0.)) ;
#12543=DIRECTION('',(0.,0.,-1.)) ;
#12544=DIRECTION('center_axis',(0.,0.,-1.)) ;
#12545=DIRECTION('ref_axis',(1.,0.,0.)) ;
#12546=DIRECTION('',(0.,0.,1.)) ;
#12547=DIRECTION('center_axis',(0.,0.,1.)) ;
#12548=DIRECTION('ref_axis',(1.,0.,0.)) ;
#12549=DIRECTION('',(0.,0.,-1.)) ;
#12550=DIRECTION('center_axis',(0.,0.,-1.)) ;
#12551=DIRECTION('ref_axis',(1.,0.,0.)) ;
#12552=DIRECTION('',(0.,0.,1.)) ;
#12553=DIRECTION('center_axis',(0.,0.,1.)) ;
#12554=DIRECTION('ref_axis',(1.,0.,0.)) ;
#12555=DIRECTION('',(0.,0.,-1.)) ;
#12556=DIRECTION('center_axis',(0.,0.,-1.)) ;
#12557=DIRECTION('ref_axis',(1.,0.,0.)) ;
#12558=DIRECTION('center_axis',(0.0074502908256619,0.99997224619817,0.)) ;
#12559=DIRECTION('ref_axis',(-0.99997224619817,0.0074502908256619,0.)) ;
#12560=DIRECTION('',(-0.99997224619817,0.0074502908256619,0.)) ;
#12561=DIRECTION('',(0.,0.,1.)) ;
#12562=DIRECTION('center_axis',(-0.63706251599997,-0.770812137104617,0.)) ;
#12563=DIRECTION('ref_axis',(0.770812137104617,-0.63706251599997,0.)) ;
#12564=DIRECTION('',(0.770812137104617,-0.63706251599997,0.)) ;
#12565=DIRECTION('center_axis',(0.,0.,1.)) ;
#12566=DIRECTION('ref_axis',(0.939692620785908,-0.342020143325669,0.)) ;
#12567=DIRECTION('center_axis',(0.,0.,1.)) ;
#12568=DIRECTION('ref_axis',(1.,0.,0.)) ;
#12569=DIRECTION('center_axis',(0.,0.,1.)) ;
#12570=DIRECTION('ref_axis',(1.,0.,0.)) ;
#12571=DIRECTION('',(-0.707106781186542,8.65956056235487E-17,0.707106781186553)) ;
#12572=DIRECTION('center_axis',(0.,0.,1.)) ;
#12573=DIRECTION('ref_axis',(0.866025403784438,-0.5,0.)) ;
#12574=DIRECTION('',(0.648477023773232,-0.761234227842003,0.)) ;
#12575=DIRECTION('',(-0.983486691428025,0.180980462437127,0.)) ;
#12576=DIRECTION('center_axis',(0.180980462437127,0.983486691428025,0.)) ;
#12577=DIRECTION('ref_axis',(-0.983486691428025,0.180980462437127,0.)) ;
#12578=DIRECTION('',(0.,0.,1.)) ;
#12579=DIRECTION('center_axis',(-0.761234227842003,-0.648477023773232,0.)) ;
#12580=DIRECTION('ref_axis',(0.648477023773232,-0.761234227842003,0.)) ;
#12581=DIRECTION('center_axis',(0.349011634277972,0.937118391207119,0.)) ;
#12582=DIRECTION('ref_axis',(-0.937118391207119,0.349011634277972,0.)) ;
#12583=DIRECTION('',(-0.937118391207119,0.349011634277972,0.)) ;
#12584=DIRECTION('',(0.,0.,1.)) ;
#12585=DIRECTION('center_axis',(-0.862276222874163,-0.506438264219704,0.)) ;
#12586=DIRECTION('ref_axis',(0.506438264219704,-0.862276222874163,0.)) ;
#12587=DIRECTION('',(0.506438264219704,-0.862276222874163,0.)) ;
#12588=DIRECTION('center_axis',(0.,0.,1.)) ;
#12589=DIRECTION('ref_axis',(0.766044443118978,-0.64278760968654,0.)) ;
#12590=DIRECTION('center_axis',(0.,0.,1.)) ;
#12591=DIRECTION('ref_axis',(0.642787609686539,-0.766044443118978,0.)) ;
#12592=DIRECTION('',(0.349011634277988,-0.937118391207113,0.)) ;
#12593=DIRECTION('',(-0.862276222874171,0.50643826421969,0.)) ;
#12594=DIRECTION('center_axis',(0.50643826421969,0.862276222874171,0.)) ;
#12595=DIRECTION('ref_axis',(-0.862276222874171,0.50643826421969,0.)) ;
#12596=DIRECTION('',(0.,0.,1.)) ;
#12597=DIRECTION('center_axis',(-0.937118391207113,-0.349011634277988,0.)) ;
#12598=DIRECTION('ref_axis',(0.349011634277988,-0.937118391207113,0.)) ;
#12599=DIRECTION('center_axis',(0.648477023773219,0.761234227842014,0.)) ;
#12600=DIRECTION('ref_axis',(-0.761234227842014,0.648477023773219,0.)) ;
#12601=DIRECTION('',(-0.761234227842014,0.648477023773219,0.)) ;
#12602=DIRECTION('',(0.,0.,1.)) ;
#12603=DIRECTION('center_axis',(-0.983486691428022,-0.180980462437143,0.)) ;
#12604=DIRECTION('ref_axis',(0.180980462437143,-0.983486691428022,0.)) ;
#12605=DIRECTION('',(0.180980462437143,-0.983486691428022,0.)) ;
#12606=DIRECTION('center_axis',(0.,0.,1.)) ;
#12607=DIRECTION('ref_axis',(0.5,-0.866025403784439,0.)) ;
#12608=DIRECTION('center_axis',(0.,0.,1.)) ;
#12609=DIRECTION('ref_axis',(0.342020143325668,-0.939692620785909,0.)) ;
#12610=DIRECTION('',(0.007450290825678,-0.99997224619817,0.)) ;
#12611=DIRECTION('',(-0.637062515999983,0.770812137104607,0.)) ;
#12612=DIRECTION('center_axis',(0.770812137104607,0.637062515999983,0.)) ;
#12613=DIRECTION('ref_axis',(-0.637062515999983,0.770812137104607,0.)) ;
#12614=DIRECTION('',(0.,0.,1.)) ;
#12615=DIRECTION('center_axis',(-0.99997224619817,-0.007450290825678,0.)) ;
#12616=DIRECTION('ref_axis',(0.007450290825678,-0.99997224619817,0.)) ;
#12617=DIRECTION('center_axis',(0.869726513699833,0.49353398197848,0.)) ;
#12618=DIRECTION('ref_axis',(-0.49353398197848,0.869726513699833,0.)) ;
#12619=DIRECTION('',(-0.49353398197848,0.869726513699833,0.)) ;
#12620=DIRECTION('',(0.,0.,1.)) ;
#12621=DIRECTION('center_axis',(-0.986074150277958,0.166306254102496,0.)) ;
#12622=DIRECTION('ref_axis',(-0.166306254102496,-0.986074150277958,0.)) ;
#12623=DIRECTION('',(-0.166306254102496,-0.986074150277958,0.)) ;
#12624=DIRECTION('center_axis',(0.,0.,1.)) ;
#12625=DIRECTION('ref_axis',(0.17364817766693,-0.984807753012208,0.)) ;
#12626=DIRECTION('center_axis',(0.,0.,1.)) ;
#12627=DIRECTION('ref_axis',(-1.83697019872103E-16,-1.,0.)) ;
#12628=DIRECTION('',(-0.33500966765479,-0.942214690279146,0.)) ;
#12629=DIRECTION('',(-0.335009667654806,0.94221469027914,0.)) ;
#12630=DIRECTION('center_axis',(0.94221469027914,0.335009667654806,0.)) ;
#12631=DIRECTION('ref_axis',(-0.335009667654806,0.94221469027914,0.)) ;
#12632=DIRECTION('',(0.,0.,1.)) ;
#12633=DIRECTION('center_axis',(-0.942214690279146,0.33500966765479,0.)) ;
#12634=DIRECTION('ref_axis',(-0.33500966765479,-0.942214690279146,0.)) ;
#12635=DIRECTION('center_axis',(0.986074150277955,0.166306254102512,0.)) ;
#12636=DIRECTION('ref_axis',(-0.166306254102512,0.986074150277955,0.)) ;
#12637=DIRECTION('',(-0.166306254102512,0.986074150277955,0.)) ;
#12638=DIRECTION('',(0.,0.,1.)) ;
#12639=DIRECTION('center_axis',(-0.869726513699841,0.493533981978465,0.)) ;
#12640=DIRECTION('ref_axis',(-0.493533981978465,-0.869726513699841,0.)) ;
#12641=DIRECTION('',(-0.493533981978465,-0.869726513699841,0.)) ;
#12642=DIRECTION('center_axis',(0.,0.,1.)) ;
#12643=DIRECTION('ref_axis',(-0.17364817766693,-0.984807753012208,0.)) ;
#12644=DIRECTION('center_axis',(0.,0.,1.)) ;
#12645=DIRECTION('ref_axis',(-0.342020143325669,-0.939692620785908,0.)) ;
#12646=DIRECTION('',(-0.63706251599997,-0.770812137104617,0.)) ;
#12647=DIRECTION('',(0.00745029082566179,0.99997224619817,0.)) ;
#12648=DIRECTION('center_axis',(0.99997224619817,-0.00745029082566179,0.)) ;
#12649=DIRECTION('ref_axis',(0.00745029082566179,0.99997224619817,0.)) ;
#12650=DIRECTION('',(0.,0.,1.)) ;
#12651=DIRECTION('center_axis',(-0.770812137104617,0.63706251599997,0.)) ;
#12652=DIRECTION('ref_axis',(-0.63706251599997,-0.770812137104617,0.)) ;
#12653=DIRECTION('center_axis',(0.983486691428025,-0.180980462437127,0.)) ;
#12654=DIRECTION('ref_axis',(0.180980462437127,0.983486691428025,0.)) ;
#12655=DIRECTION('',(0.180980462437127,0.983486691428025,0.)) ;
#12656=DIRECTION('',(0.,0.,1.)) ;
#12657=DIRECTION('center_axis',(-0.648477023773232,0.761234227842003,0.)) ;
#12658=DIRECTION('ref_axis',(-0.761234227842003,-0.648477023773232,0.)) ;
#12659=DIRECTION('',(-0.761234227842003,-0.648477023773232,0.)) ;
#12660=DIRECTION('center_axis',(0.,0.,1.)) ;
#12661=DIRECTION('ref_axis',(-0.5,-0.866025403784438,0.)) ;
#12662=DIRECTION('center_axis',(0.,0.,1.)) ;
#12663=DIRECTION('ref_axis',(-0.642787609686539,-0.766044443118978,0.)) ;
#12664=DIRECTION('',(-0.862276222874163,-0.506438264219704,0.)) ;
#12665=DIRECTION('',(0.349011634277972,0.937118391207119,0.)) ;
#12666=DIRECTION('center_axis',(0.937118391207119,-0.349011634277972,0.)) ;
#12667=DIRECTION('ref_axis',(0.349011634277972,0.937118391207119,0.)) ;
#12668=DIRECTION('',(0.,0.,1.)) ;
#12669=DIRECTION('center_axis',(-0.506438264219705,0.862276222874163,0.)) ;
#12670=DIRECTION('ref_axis',(-0.862276222874163,-0.506438264219704,0.)) ;
#12671=DIRECTION('center_axis',(0.862276222874172,-0.50643826421969,0.)) ;
#12672=DIRECTION('ref_axis',(0.50643826421969,0.862276222874171,0.)) ;
#12673=DIRECTION('',(0.50643826421969,0.862276222874171,0.)) ;
#12674=DIRECTION('',(0.,0.,1.)) ;
#12675=DIRECTION('center_axis',(-0.349011634277988,0.937118391207113,0.)) ;
#12676=DIRECTION('ref_axis',(-0.937118391207113,-0.349011634277988,0.)) ;
#12677=DIRECTION('',(-0.937118391207113,-0.349011634277988,0.)) ;
#12678=DIRECTION('center_axis',(0.,0.,1.)) ;
#12679=DIRECTION('ref_axis',(-0.766044443118978,-0.642787609686539,0.)) ;
#12680=DIRECTION('center_axis',(0.,0.,1.)) ;
#12681=DIRECTION('ref_axis',(-0.866025403784439,-0.5,0.)) ;
#12682=DIRECTION('',(-0.983486691428022,-0.180980462437143,0.)) ;
#12683=DIRECTION('',(0.648477023773219,0.761234227842014,0.)) ;
#12684=DIRECTION('center_axis',(0.761234227842014,-0.648477023773219,0.)) ;
#12685=DIRECTION('ref_axis',(0.648477023773219,0.761234227842014,0.)) ;
#12686=DIRECTION('',(0.,0.,1.)) ;
#12687=DIRECTION('center_axis',(-0.180980462437143,0.983486691428022,0.)) ;
#12688=DIRECTION('ref_axis',(-0.983486691428022,-0.180980462437143,0.)) ;
#12689=DIRECTION('center_axis',(0.637062515999983,-0.770812137104607,0.)) ;
#12690=DIRECTION('ref_axis',(0.770812137104607,0.637062515999983,0.)) ;
#12691=DIRECTION('',(0.770812137104607,0.637062515999983,0.)) ;
#12692=DIRECTION('',(0.,0.,1.)) ;
#12693=DIRECTION('center_axis',(-0.00745029082567855,0.99997224619817,0.)) ;
#12694=DIRECTION('ref_axis',(-0.99997224619817,-0.00745029082567855,0.)) ;
#12695=DIRECTION('',(-0.99997224619817,-0.00745029082567855,0.)) ;
#12696=DIRECTION('center_axis',(0.,0.,1.)) ;
#12697=DIRECTION('ref_axis',(-0.939692620785909,-0.342020143325669,0.)) ;
#12698=DIRECTION('center_axis',(0.,0.,1.)) ;
#12699=DIRECTION('ref_axis',(-0.984807753012208,-0.17364817766693,0.)) ;
#12700=DIRECTION('',(-0.986074150277958,0.166306254102495,0.)) ;
#12701=DIRECTION('',(0.869726513699833,0.49353398197848,0.)) ;
#12702=DIRECTION('center_axis',(0.49353398197848,-0.869726513699833,0.)) ;
#12703=DIRECTION('ref_axis',(0.869726513699833,0.49353398197848,0.)) ;
#12704=DIRECTION('',(0.,0.,1.)) ;
#12705=DIRECTION('center_axis',(0.166306254102495,0.986074150277958,0.)) ;
#12706=DIRECTION('ref_axis',(-0.986074150277958,0.166306254102495,0.)) ;
#12707=DIRECTION('center_axis',(0.335009667654806,-0.94221469027914,0.)) ;
#12708=DIRECTION('ref_axis',(0.94221469027914,0.335009667654806,0.)) ;
#12709=DIRECTION('',(0.94221469027914,0.335009667654806,0.)) ;
#12710=DIRECTION('',(0.,0.,1.)) ;
#12711=DIRECTION('center_axis',(0.33500966765479,0.942214690279146,0.)) ;
#12712=DIRECTION('ref_axis',(-0.942214690279146,0.33500966765479,0.)) ;
#12713=DIRECTION('',(-0.942214690279146,0.33500966765479,0.)) ;
#12714=DIRECTION('center_axis',(0.,0.,1.)) ;
#12715=DIRECTION('ref_axis',(-1.,1.22464679914735E-16,0.)) ;
#12716=DIRECTION('center_axis',(0.,0.,1.)) ;
#12717=DIRECTION('ref_axis',(-0.984807753012208,0.173648177666931,0.)) ;
#12718=DIRECTION('',(-0.869726513699841,0.493533981978465,0.)) ;
#12719=DIRECTION('',(0.986074150277955,0.166306254102512,0.)) ;
#12720=DIRECTION('center_axis',(0.166306254102512,-0.986074150277955,0.)) ;
#12721=DIRECTION('ref_axis',(0.986074150277955,0.166306254102512,0.)) ;
#12722=DIRECTION('',(0.,0.,1.)) ;
#12723=DIRECTION('center_axis',(0.493533981978465,0.869726513699841,0.)) ;
#12724=DIRECTION('ref_axis',(-0.869726513699841,0.493533981978465,0.)) ;
#12725=DIRECTION('center_axis',(-0.00745029082566129,-0.99997224619817,
0.)) ;
#12726=DIRECTION('ref_axis',(0.99997224619817,-0.00745029082566129,0.)) ;
#12727=DIRECTION('',(0.99997224619817,-0.00745029082566129,0.)) ;
#12728=DIRECTION('',(0.,0.,1.)) ;
#12729=DIRECTION('center_axis',(0.63706251599997,0.770812137104618,0.)) ;
#12730=DIRECTION('ref_axis',(-0.770812137104618,0.63706251599997,0.)) ;
#12731=DIRECTION('',(-0.770812137104618,0.63706251599997,0.)) ;
#12732=DIRECTION('center_axis',(0.,0.,1.)) ;
#12733=DIRECTION('ref_axis',(-0.939692620785908,0.342020143325669,0.)) ;
#12734=DIRECTION('center_axis',(0.,0.,1.)) ;
#12735=DIRECTION('ref_axis',(-0.866025403784439,0.5,0.)) ;
#12736=DIRECTION('',(-0.648477023773233,0.761234227842003,0.)) ;
#12737=DIRECTION('',(0.983486691428025,-0.180980462437126,0.)) ;
#12738=DIRECTION('center_axis',(-0.180980462437126,-0.983486691428025,0.)) ;
#12739=DIRECTION('ref_axis',(0.983486691428025,-0.180980462437126,0.)) ;
#12740=DIRECTION('',(0.,0.,1.)) ;
#12741=DIRECTION('center_axis',(0.761234227842003,0.648477023773233,0.)) ;
#12742=DIRECTION('ref_axis',(-0.648477023773233,0.761234227842003,0.)) ;
#12743=DIRECTION('center_axis',(-0.349011634277972,-0.937118391207119,0.)) ;
#12744=DIRECTION('ref_axis',(0.937118391207119,-0.349011634277972,0.)) ;
#12745=DIRECTION('',(0.937118391207119,-0.349011634277972,0.)) ;
#12746=DIRECTION('',(0.,0.,1.)) ;
#12747=DIRECTION('center_axis',(0.862276222874163,0.506438264219705,0.)) ;
#12748=DIRECTION('ref_axis',(-0.506438264219704,0.862276222874163,0.)) ;
#12749=DIRECTION('',(-0.506438264219704,0.862276222874163,0.)) ;
#12750=DIRECTION('center_axis',(0.,0.,1.)) ;
#12751=DIRECTION('ref_axis',(-0.766044443118978,0.642787609686539,0.)) ;
#12752=DIRECTION('center_axis',(0.,0.,1.)) ;
#12753=DIRECTION('ref_axis',(-0.642787609686539,0.766044443118978,0.)) ;
#12754=DIRECTION('',(-0.349011634277988,0.937118391207113,0.)) ;
#12755=DIRECTION('',(0.862276222874171,-0.506438264219689,0.)) ;
#12756=DIRECTION('center_axis',(-0.50643826421969,-0.862276222874172,0.)) ;
#12757=DIRECTION('ref_axis',(0.862276222874171,-0.506438264219689,0.)) ;
#12758=DIRECTION('',(0.,0.,1.)) ;
#12759=DIRECTION('center_axis',(0.937118391207113,0.349011634277988,0.)) ;
#12760=DIRECTION('ref_axis',(-0.349011634277988,0.937118391207113,0.)) ;
#12761=DIRECTION('center_axis',(-0.648477023773219,-0.761234227842014,0.)) ;
#12762=DIRECTION('ref_axis',(0.761234227842014,-0.648477023773219,0.)) ;
#12763=DIRECTION('',(0.761234227842014,-0.648477023773219,0.)) ;
#12764=DIRECTION('',(0.,0.,1.)) ;
#12765=DIRECTION('center_axis',(0.983486691428022,0.180980462437143,0.)) ;
#12766=DIRECTION('ref_axis',(-0.180980462437143,0.983486691428022,0.)) ;
#12767=DIRECTION('',(-0.180980462437143,0.983486691428022,0.)) ;
#12768=DIRECTION('center_axis',(0.,0.,1.)) ;
#12769=DIRECTION('ref_axis',(-0.5,0.866025403784439,0.)) ;
#12770=DIRECTION('center_axis',(0.,0.,1.)) ;
#12771=DIRECTION('ref_axis',(-0.342020143325669,0.939692620785908,0.)) ;
#12772=DIRECTION('',(-0.00745029082567861,0.99997224619817,0.)) ;
#12773=DIRECTION('',(0.637062515999983,-0.770812137104607,0.)) ;
#12774=DIRECTION('center_axis',(-0.770812137104607,-0.637062515999983,0.)) ;
#12775=DIRECTION('ref_axis',(0.637062515999983,-0.770812137104607,0.)) ;
#12776=DIRECTION('',(0.,0.,1.)) ;
#12777=DIRECTION('center_axis',(0.99997224619817,0.00745029082567861,0.)) ;
#12778=DIRECTION('ref_axis',(-0.00745029082567861,0.99997224619817,0.)) ;
#12779=DIRECTION('center_axis',(-0.869726513699833,-0.49353398197848,0.)) ;
#12780=DIRECTION('ref_axis',(0.49353398197848,-0.869726513699833,0.)) ;
#12781=DIRECTION('',(0.49353398197848,-0.869726513699833,0.)) ;
#12782=DIRECTION('',(0.,0.,1.)) ;
#12783=DIRECTION('center_axis',(0.986074150277958,-0.166306254102495,0.)) ;
#12784=DIRECTION('ref_axis',(0.166306254102495,0.986074150277958,0.)) ;
#12785=DIRECTION('',(0.166306254102495,0.986074150277958,0.)) ;
#12786=DIRECTION('center_axis',(0.,0.,1.)) ;
#12787=DIRECTION('ref_axis',(-0.17364817766693,0.984807753012208,0.)) ;
#12788=DIRECTION('center_axis',(0.,0.,1.)) ;
#12789=DIRECTION('ref_axis',(6.12323399573677E-17,1.,0.)) ;
#12790=DIRECTION('',(0.33500966765479,0.942214690279146,0.)) ;
#12791=DIRECTION('',(0.335009667654806,-0.94221469027914,0.)) ;
#12792=DIRECTION('center_axis',(-0.94221469027914,-0.335009667654806,0.)) ;
#12793=DIRECTION('ref_axis',(0.335009667654806,-0.94221469027914,0.)) ;
#12794=DIRECTION('',(0.,0.,1.)) ;
#12795=DIRECTION('center_axis',(0.942214690279146,-0.33500966765479,0.)) ;
#12796=DIRECTION('ref_axis',(0.33500966765479,0.942214690279146,0.)) ;
#12797=DIRECTION('center_axis',(-0.986074150277955,-0.166306254102512,0.)) ;
#12798=DIRECTION('ref_axis',(0.166306254102512,-0.986074150277955,0.)) ;
#12799=DIRECTION('',(0.166306254102512,-0.986074150277955,0.)) ;
#12800=DIRECTION('',(0.,0.,1.)) ;
#12801=DIRECTION('center_axis',(0.869726513699841,-0.493533981978465,0.)) ;
#12802=DIRECTION('ref_axis',(0.493533981978465,0.869726513699841,0.)) ;
#12803=DIRECTION('',(0.493533981978465,0.869726513699841,0.)) ;
#12804=DIRECTION('center_axis',(0.,0.,1.)) ;
#12805=DIRECTION('ref_axis',(0.17364817766693,0.984807753012208,0.)) ;
#12806=DIRECTION('center_axis',(0.,0.,1.)) ;
#12807=DIRECTION('ref_axis',(0.342020143325669,0.939692620785908,0.)) ;
#12808=DIRECTION('',(0.63706251599997,0.770812137104618,0.)) ;
#12809=DIRECTION('',(-0.00745029082566129,-0.99997224619817,0.)) ;
#12810=DIRECTION('center_axis',(-0.99997224619817,0.00745029082566129,0.)) ;
#12811=DIRECTION('ref_axis',(-0.00745029082566129,-0.99997224619817,0.)) ;
#12812=DIRECTION('',(0.,0.,1.)) ;
#12813=DIRECTION('center_axis',(0.770812137104618,-0.63706251599997,0.)) ;
#12814=DIRECTION('ref_axis',(0.63706251599997,0.770812137104618,0.)) ;
#12815=DIRECTION('center_axis',(-0.983486691428025,0.180980462437126,0.)) ;
#12816=DIRECTION('ref_axis',(-0.180980462437126,-0.983486691428025,0.)) ;
#12817=DIRECTION('',(-0.180980462437126,-0.983486691428025,0.)) ;
#12818=DIRECTION('',(0.,0.,1.)) ;
#12819=DIRECTION('center_axis',(0.648477023773232,-0.761234227842003,0.)) ;
#12820=DIRECTION('ref_axis',(0.761234227842003,0.648477023773232,0.)) ;
#12821=DIRECTION('',(0.761234227842003,0.648477023773232,0.)) ;
#12822=DIRECTION('center_axis',(0.,0.,1.)) ;
#12823=DIRECTION('ref_axis',(0.5,0.866025403784439,0.)) ;
#12824=DIRECTION('center_axis',(0.,0.,1.)) ;
#12825=DIRECTION('ref_axis',(0.642787609686539,0.766044443118978,0.)) ;
#12826=DIRECTION('',(0.862276222874163,0.506438264219705,0.)) ;
#12827=DIRECTION('',(-0.349011634277972,-0.937118391207119,0.)) ;
#12828=DIRECTION('center_axis',(-0.937118391207119,0.349011634277972,0.)) ;
#12829=DIRECTION('ref_axis',(-0.349011634277972,-0.937118391207119,0.)) ;
#12830=DIRECTION('',(0.,0.,1.)) ;
#12831=DIRECTION('center_axis',(0.506438264219705,-0.862276222874163,0.)) ;
#12832=DIRECTION('ref_axis',(0.862276222874163,0.506438264219705,0.)) ;
#12833=DIRECTION('center_axis',(-0.862276222874172,0.50643826421969,0.)) ;
#12834=DIRECTION('ref_axis',(-0.50643826421969,-0.862276222874171,0.)) ;
#12835=DIRECTION('',(-0.50643826421969,-0.862276222874171,0.)) ;
#12836=DIRECTION('',(0.,0.,1.)) ;
#12837=DIRECTION('center_axis',(0.349011634277988,-0.937118391207113,0.)) ;
#12838=DIRECTION('ref_axis',(0.937118391207113,0.349011634277988,0.)) ;
#12839=DIRECTION('',(0.937118391207113,0.349011634277988,0.)) ;
#12840=DIRECTION('center_axis',(0.,0.,1.)) ;
#12841=DIRECTION('ref_axis',(0.766044443118978,0.642787609686539,0.)) ;
#12842=DIRECTION('center_axis',(0.,0.,1.)) ;
#12843=DIRECTION('ref_axis',(0.866025403784439,0.5,0.)) ;
#12844=DIRECTION('',(0.983486691428022,0.180980462437143,0.)) ;
#12845=DIRECTION('',(-0.648477023773219,-0.761234227842014,0.)) ;
#12846=DIRECTION('center_axis',(-0.761234227842014,0.648477023773219,0.)) ;
#12847=DIRECTION('ref_axis',(-0.648477023773219,-0.761234227842014,0.)) ;
#12848=DIRECTION('',(0.,0.,1.)) ;
#12849=DIRECTION('center_axis',(0.180980462437143,-0.983486691428022,0.)) ;
#12850=DIRECTION('ref_axis',(0.983486691428022,0.180980462437143,0.)) ;
#12851=DIRECTION('center_axis',(-0.637062515999983,0.770812137104607,0.)) ;
#12852=DIRECTION('ref_axis',(-0.770812137104607,-0.637062515999983,0.)) ;
#12853=DIRECTION('',(-0.770812137104607,-0.637062515999983,0.)) ;
#12854=DIRECTION('',(0.,0.,1.)) ;
#12855=DIRECTION('center_axis',(0.00745029082567861,-0.99997224619817,0.)) ;
#12856=DIRECTION('ref_axis',(0.99997224619817,0.00745029082567861,0.)) ;
#12857=DIRECTION('',(0.99997224619817,0.00745029082567861,0.)) ;
#12858=DIRECTION('center_axis',(0.,0.,1.)) ;
#12859=DIRECTION('ref_axis',(0.939692620785908,0.342020143325669,0.)) ;
#12860=DIRECTION('center_axis',(0.,0.,1.)) ;
#12861=DIRECTION('ref_axis',(0.984807753012208,0.17364817766693,0.)) ;
#12862=DIRECTION('',(0.986074150277958,-0.166306254102495,0.)) ;
#12863=DIRECTION('',(-0.869726513699833,-0.49353398197848,0.)) ;
#12864=DIRECTION('center_axis',(-0.49353398197848,0.869726513699833,0.)) ;
#12865=DIRECTION('ref_axis',(-0.869726513699833,-0.49353398197848,0.)) ;
#12866=DIRECTION('',(0.,0.,1.)) ;
#12867=DIRECTION('center_axis',(-0.166306254102495,-0.986074150277958,0.)) ;
#12868=DIRECTION('ref_axis',(0.986074150277958,-0.166306254102495,0.)) ;
#12869=DIRECTION('center_axis',(-0.335009667654806,0.94221469027914,0.)) ;
#12870=DIRECTION('ref_axis',(-0.94221469027914,-0.335009667654806,0.)) ;
#12871=DIRECTION('',(-0.94221469027914,-0.335009667654806,0.)) ;
#12872=DIRECTION('',(0.,0.,1.)) ;
#12873=DIRECTION('center_axis',(-0.33500966765479,-0.942214690279146,0.)) ;
#12874=DIRECTION('ref_axis',(0.942214690279146,-0.33500966765479,0.)) ;
#12875=DIRECTION('',(0.942214690279146,-0.33500966765479,0.)) ;
#12876=DIRECTION('center_axis',(0.,0.,1.)) ;
#12877=DIRECTION('ref_axis',(1.,0.,0.)) ;
#12878=DIRECTION('center_axis',(0.,0.,1.)) ;
#12879=DIRECTION('ref_axis',(1.,0.,0.)) ;
#12880=DIRECTION('center_axis',(0.,-1.,0.)) ;
#12881=DIRECTION('ref_axis',(-1.,0.,0.)) ;
#12882=DIRECTION('center_axis',(0.,0.,1.)) ;
#12883=DIRECTION('ref_axis',(1.,0.,0.)) ;
#12884=DIRECTION('center_axis',(0.,0.,1.)) ;
#12885=DIRECTION('ref_axis',(1.,0.,0.)) ;
#12886=DIRECTION('center_axis',(0.,0.,-1.)) ;
#12887=DIRECTION('ref_axis',(1.,0.,0.)) ;
#12888=DIRECTION('',(0.70710678118654,8.65956056235484E-17,0.707106781186555)) ;
#12889=DIRECTION('center_axis',(0.,0.,1.)) ;
#12890=DIRECTION('ref_axis',(1.,0.,0.)) ;
#12891=DIRECTION('center_axis',(0.,0.,1.)) ;
#12892=DIRECTION('ref_axis',(1.,0.,0.)) ;
#12893=DIRECTION('center_axis',(0.,0.,1.)) ;
#12894=DIRECTION('ref_axis',(1.,0.,0.)) ;
#12895=DIRECTION('center_axis',(0.,0.,1.)) ;
#12896=DIRECTION('ref_axis',(1.,0.,0.)) ;
#12897=DIRECTION('center_axis',(0.,0.,1.)) ;
#12898=DIRECTION('ref_axis',(1.,0.,0.)) ;
#12899=DIRECTION('center_axis',(0.,0.,1.)) ;
#12900=DIRECTION('ref_axis',(1.,0.,0.)) ;
#12901=DIRECTION('center_axis',(0.,0.,1.)) ;
#12902=DIRECTION('ref_axis',(1.,0.,0.)) ;
#12903=DIRECTION('',(0.,0.,-1.)) ;
#12904=DIRECTION('',(0.,0.,1.)) ;
#12905=DIRECTION('center_axis',(0.,0.,-1.)) ;
#12906=DIRECTION('ref_axis',(1.,0.,0.)) ;
#12907=DIRECTION('center_axis',(0.,0.,1.)) ;
#12908=DIRECTION('ref_axis',(1.,0.,0.)) ;
#12909=DIRECTION('',(0.,0.,-1.)) ;
#12910=DIRECTION('',(0.,0.,1.)) ;
#12911=DIRECTION('center_axis',(0.,0.,-1.)) ;
#12912=DIRECTION('ref_axis',(1.,0.,0.)) ;
#12913=DIRECTION('center_axis',(0.,0.,1.)) ;
#12914=DIRECTION('ref_axis',(1.,0.,0.)) ;
#12915=DIRECTION('',(0.,0.,1.)) ;
#12916=DIRECTION('center_axis',(0.,0.,-1.)) ;
#12917=DIRECTION('ref_axis',(1.,0.,0.)) ;
#12918=DIRECTION('',(0.,0.,-1.)) ;
#12919=DIRECTION('center_axis',(0.,0.,1.)) ;
#12920=DIRECTION('ref_axis',(1.,0.,0.)) ;
#12921=DIRECTION('',(0.,0.,-1.)) ;
#12922=DIRECTION('',(0.,0.,1.)) ;
#12923=DIRECTION('center_axis',(0.,0.,-1.)) ;
#12924=DIRECTION('ref_axis',(1.,0.,0.)) ;
#12925=DIRECTION('center_axis',(0.,0.,1.)) ;
#12926=DIRECTION('ref_axis',(1.,0.,0.)) ;
#12927=DIRECTION('',(0.,0.,1.)) ;
#12928=DIRECTION('center_axis',(0.,0.,-1.)) ;
#12929=DIRECTION('ref_axis',(1.,0.,0.)) ;
#12930=DIRECTION('',(0.,0.,-1.)) ;
#12931=DIRECTION('center_axis',(0.,0.,1.)) ;
#12932=DIRECTION('ref_axis',(1.,0.,0.)) ;
#12933=DIRECTION('',(0.,0.,1.)) ;
#12934=DIRECTION('center_axis',(0.,0.,-1.)) ;
#12935=DIRECTION('ref_axis',(1.,0.,0.)) ;
#12936=DIRECTION('',(0.,0.,-1.)) ;
#12937=DIRECTION('center_axis',(0.,1.,0.)) ;
#12938=DIRECTION('ref_axis',(-1.,0.,0.)) ;
#12939=DIRECTION('',(-1.,0.,0.)) ;
#12940=DIRECTION('',(0.,0.,1.)) ;
#12941=DIRECTION('',(-1.,0.,0.)) ;
#12942=DIRECTION('',(0.,0.,1.)) ;
#12943=DIRECTION('center_axis',(0.866025403784449,0.499999999999982,0.)) ;
#12944=DIRECTION('ref_axis',(-0.499999999999982,0.866025403784449,0.)) ;
#12945=DIRECTION('',(-0.499999999999982,0.866025403784449,0.)) ;
#12946=DIRECTION('',(0.,0.,1.)) ;
#12947=DIRECTION('',(-0.499999999999982,0.866025403784449,0.)) ;
#12948=DIRECTION('center_axis',(0.866025403784449,-0.499999999999982,0.)) ;
#12949=DIRECTION('ref_axis',(0.499999999999982,0.866025403784449,0.)) ;
#12950=DIRECTION('',(0.499999999999982,0.866025403784449,0.)) ;
#12951=DIRECTION('',(0.,0.,1.)) ;
#12952=DIRECTION('',(0.499999999999982,0.866025403784449,0.)) ;
#12953=DIRECTION('center_axis',(0.,0.,1.)) ;
#12954=DIRECTION('ref_axis',(1.,0.,0.)) ;
#12955=DIRECTION('center_axis',(0.,0.,1.)) ;
#12956=DIRECTION('ref_axis',(1.,0.,0.)) ;
#12957=DIRECTION('center_axis',(0.,0.,1.)) ;
#12958=DIRECTION('ref_axis',(1.,0.,0.)) ;
#12959=DIRECTION('',(1.,0.,0.)) ;
#12960=DIRECTION('center_axis',(0.,0.,1.)) ;
#12961=DIRECTION('ref_axis',(1.,0.,0.)) ;
#12962=DIRECTION('center_axis',(0.,0.,1.)) ;
#12963=DIRECTION('ref_axis',(1.,0.,0.)) ;
#12964=DIRECTION('',(0.499999999999997,-0.86602540378444,0.)) ;
#12965=DIRECTION('center_axis',(0.,0.,1.)) ;
#12966=DIRECTION('ref_axis',(1.,0.,0.)) ;
#12967=DIRECTION('',(-0.499999999999997,-0.86602540378444,0.)) ;
#12968=DIRECTION('center_axis',(0.,0.,-1.)) ;
#12969=DIRECTION('ref_axis',(-1.,0.,0.)) ;
#12970=DIRECTION('',(1.,0.,0.)) ;
#12971=DIRECTION('center_axis',(0.,0.,1.)) ;
#12972=DIRECTION('ref_axis',(1.,0.,0.)) ;
#12973=DIRECTION('center_axis',(0.,0.,-1.)) ;
#12974=DIRECTION('ref_axis',(-1.,0.,0.)) ;
#12975=DIRECTION('center_axis',(0.,0.,1.)) ;
#12976=DIRECTION('ref_axis',(1.,0.,0.)) ;
#12977=DIRECTION('center_axis',(0.,0.,-1.)) ;
#12978=DIRECTION('ref_axis',(-1.,0.,0.)) ;
#12979=DIRECTION('center_axis',(0.,0.,1.)) ;
#12980=DIRECTION('ref_axis',(1.,0.,0.)) ;
#12981=DIRECTION('center_axis',(0.,0.,-1.)) ;
#12982=DIRECTION('ref_axis',(-1.,0.,0.)) ;
#12983=DIRECTION('center_axis',(0.,0.,1.)) ;
#12984=DIRECTION('ref_axis',(1.,0.,0.)) ;
#12985=DIRECTION('center_axis',(0.,0.,-1.)) ;
#12986=DIRECTION('ref_axis',(-1.,0.,0.)) ;
#12987=DIRECTION('',(-0.499999999999997,-0.86602540378444,0.)) ;
#12988=DIRECTION('center_axis',(0.,0.,1.)) ;
#12989=DIRECTION('ref_axis',(1.,0.,0.)) ;
#12990=DIRECTION('center_axis',(0.,0.,-1.)) ;
#12991=DIRECTION('ref_axis',(-1.,0.,0.)) ;
#12992=DIRECTION('',(0.499999999999997,-0.86602540378444,0.)) ;
#12993=DIRECTION('center_axis',(0.,0.,1.)) ;
#12994=DIRECTION('ref_axis',(1.,0.,0.)) ;
#12995=DIRECTION('center_axis',(0.,0.,-1.)) ;
#12996=DIRECTION('ref_axis',(1.,0.,0.)) ;
#12997=DIRECTION('',(0.857167300702111,1.04972719113862E-16,0.515038074910056)) ;
#12998=DIRECTION('center_axis',(0.,-1.,0.)) ;
#12999=DIRECTION('ref_axis',(1.,0.,0.)) ;
#13000=DIRECTION('',(0.,0.,1.)) ;
#13001=DIRECTION('center_axis',(-0.86602540378444,-0.499999999999997,0.)) ;
#13002=DIRECTION('ref_axis',(0.499999999999997,-0.86602540378444,0.)) ;
#13003=DIRECTION('',(0.,0.,1.)) ;
#13004=DIRECTION('center_axis',(-0.86602540378444,0.499999999999997,0.)) ;
#13005=DIRECTION('ref_axis',(-0.499999999999997,-0.86602540378444,0.)) ;
#15298=CARTESIAN_POINT('',(0.,0.,0.)) ;
#15299=CARTESIAN_POINT('Origin',(84.75,52.3,26.4)) ;
#15300=CARTESIAN_POINT('',(83.7822752358061,52.3006823179371,26.6289859168897)) ;
#15301=CARTESIAN_POINT('',(83.7824753621529,52.3008465510102,26.5710140831103)) ;
#15302=CARTESIAN_POINT('',(83.78325,52.3,26.4)) ;
#15303=CARTESIAN_POINT('',(85.1756413254134,53.1688316687951,26.5)) ;
#15304=CARTESIAN_POINT('Ctrl Pts',(83.7822752358061,52.3006823179371,26.6289859168897)) ;
#15305=CARTESIAN_POINT('Ctrl Pts',(83.7819669536534,52.3408924644816,26.626330348121)) ;
#15306=CARTESIAN_POINT('Ctrl Pts',(83.784257904817,52.381065877484,26.6236747793523)) ;
#15307=CARTESIAN_POINT('Ctrl Pts',(83.7892671574507,52.4208955203977,26.6210192105835)) ;
#15308=CARTESIAN_POINT('Ctrl Pts',(83.8289601627117,52.7365031252282,26.5999766493842)) ;
#15309=CARTESIAN_POINT('Ctrl Pts',(84.0393320199538,53.0305258231898,26.5789340881849)) ;
#15310=CARTESIAN_POINT('Ctrl Pts',(84.3252599776053,53.1701364250497,26.5578915269857)) ;
#15311=CARTESIAN_POINT('Ctrl Pts',(84.5874715008695,53.2981669572095,26.5385943513238)) ;
#15312=CARTESIAN_POINT('Ctrl Pts',(84.9132248715999,53.2963386188841,26.5192971756619)) ;
#15313=CARTESIAN_POINT('Ctrl Pts',(85.1761635223117,53.1694011139097,26.5)) ;
#15314=CARTESIAN_POINT('',(84.3248808714849,53.1682622236805,26.5)) ;
#15315=CARTESIAN_POINT('Origin',(84.75,52.3,26.5)) ;
#15316=CARTESIAN_POINT('Ctrl Pts',(84.3248808714849,53.1682622236805,26.5)) ;
#15317=CARTESIAN_POINT('Ctrl Pts',(84.037889141541,53.0277451416316,26.5210425611993)) ;
#15318=CARTESIAN_POINT('Ctrl Pts',(83.8284581828498,52.7349003276012,26.5420851223986)) ;
#15319=CARTESIAN_POINT('Ctrl Pts',(83.7892954018501,52.419717415322,26.5631276835978)) ;
#15320=CARTESIAN_POINT('Ctrl Pts',(83.7844028837125,52.3803423230635,26.5657564834353)) ;
#15321=CARTESIAN_POINT('Ctrl Pts',(83.7821677312968,52.3406186013818,26.5683852832728)) ;
#15322=CARTESIAN_POINT('Ctrl Pts',(83.7824753621529,52.3008465510102,26.5710140831103)) ;
#15323=CARTESIAN_POINT('Origin',(84.75,52.3,26.4)) ;
#15324=CARTESIAN_POINT('',(83.7847331702872,52.3001910598074,27.0289859168897)) ;
#15325=CARTESIAN_POINT('',(83.7847326912755,52.3002006015805,26.9710140831103)) ;
#15326=CARTESIAN_POINT('',(83.78325,52.3,26.4)) ;
#15327=CARTESIAN_POINT('Ctrl Pts',(83.7847331702872,52.3001910598074,27.0289859168897)) ;
#15328=CARTESIAN_POINT('Ctrl Pts',(83.7844687406298,52.4485469749339,27.0192523819834)) ;
#15329=CARTESIAN_POINT('Ctrl Pts',(83.8166138594215,52.5967941566235,27.0095188470771)) ;
#15330=CARTESIAN_POINT('Ctrl Pts',(83.881769803326,52.7287399208488,26.9997853121707)) ;
#15331=CARTESIAN_POINT('Ctrl Pts',(84.0226279756452,53.013988481153,26.9787427509714)) ;
#15332=CARTESIAN_POINT('Ctrl Pts',(84.3177671305919,53.2230499514336,26.9577001897721)) ;
#15333=CARTESIAN_POINT('Ctrl Pts',(84.6335926430084,53.2612954524669,26.9366576285729)) ;
#15334=CARTESIAN_POINT('Ctrl Pts',(84.9494181554248,53.2995409535003,26.9156150673736)) ;
#15335=CARTESIAN_POINT('Ctrl Pts',(85.2859300253108,53.1669704852863,26.8945725061743)) ;
#15336=CARTESIAN_POINT('Ctrl Pts',(85.4908016015415,52.9235850495878,26.873529944975)) ;
#15337=CARTESIAN_POINT('Ctrl Pts',(85.6956731777722,52.6801996138893,26.8524873837757)) ;
#15338=CARTESIAN_POINT('Ctrl Pts',(85.7689044603475,52.3259992107062,26.8314448225764)) ;
#15339=CARTESIAN_POINT('Ctrl Pts',(85.677353054767,52.0213297802181,26.8104022613771)) ;
#15340=CARTESIAN_POINT('Ctrl Pts',(85.5858016491865,51.7166603497299,26.7893597001778)) ;
#15341=CARTESIAN_POINT('Ctrl Pts',(85.3294675554503,51.4615218919368,26.7683171389785)) ;
#15342=CARTESIAN_POINT('Ctrl Pts',(85.0243692392349,51.371372572711,26.7472745777793)) ;
#15343=CARTESIAN_POINT('Ctrl Pts',(84.7192709230194,51.2812232534852,26.72623201658)) ;
#15344=CARTESIAN_POINT('Ctrl Pts',(84.3654083843247,51.3560630728268,26.7051894553807)) ;
#15345=CARTESIAN_POINT('Ctrl Pts',(84.1229841916173,51.5620792383473,26.6841468941814)) ;
#15346=CARTESIAN_POINT('Ctrl Pts',(83.9111539037505,51.7420961878111,26.6657599017508)) ;
#15347=CARTESIAN_POINT('Ctrl Pts',(83.7844097621927,52.0222697726265,26.6473729093203)) ;
#15348=CARTESIAN_POINT('Ctrl Pts',(83.7822752358061,52.3006823179371,26.6289859168897)) ;
#15349=CARTESIAN_POINT('Ctrl Pts',(83.7824753621529,52.3008465510102,26.5710140831103)) ;
#15350=CARTESIAN_POINT('Ctrl Pts',(83.7846302014414,52.0222581876176,26.5894278444721)) ;
#15351=CARTESIAN_POINT('Ctrl Pts',(83.9115461789277,51.7412985869987,26.6078416058339)) ;
#15352=CARTESIAN_POINT('Ctrl Pts',(84.1238435334506,51.5611752748842,26.6262553671957)) ;
#15353=CARTESIAN_POINT('Ctrl Pts',(84.366449049359,51.3553370572536,26.647297928395)) ;
#15354=CARTESIAN_POINT('Ctrl Pts',(84.720554684484,51.2811816325205,26.6683404895943)) ;
#15355=CARTESIAN_POINT('Ctrl Pts',(85.0255768160984,51.3717764490523,26.6893830507936)) ;
#15356=CARTESIAN_POINT('Ctrl Pts',(85.3305989477127,51.4623712655841,26.7104256119929)) ;
#15357=CARTESIAN_POINT('Ctrl Pts',(85.5865375758163,51.7177163233807,26.7314681731922)) ;
#15358=CARTESIAN_POINT('Ctrl Pts',(85.6776859602006,52.0224714271219,26.7525107343915)) ;
#15359=CARTESIAN_POINT('Ctrl Pts',(85.7688343445849,52.3272265308631,26.7735532955908)) ;
#15360=CARTESIAN_POINT('Ctrl Pts',(85.6951924852498,52.6813916805489,26.79459585679)) ;
#15361=CARTESIAN_POINT('Ctrl Pts',(85.4900232232115,52.9245330496733,26.8156384179893)) ;
#15362=CARTESIAN_POINT('Ctrl Pts',(85.2848539611732,53.1676744187977,26.8366809791886)) ;
#15363=CARTESIAN_POINT('Ctrl Pts',(84.9481572964317,53.2997920073608,26.8577235403879)) ;
#15364=CARTESIAN_POINT('Ctrl Pts',(84.6323757540708,53.2611409632297,26.8787661015872)) ;
#15365=CARTESIAN_POINT('Ctrl Pts',(84.3165942117099,53.2224899190985,26.8998086627865)) ;
#15366=CARTESIAN_POINT('Ctrl Pts',(84.0217277917296,53.0130702422731,26.9208512239858)) ;
#15367=CARTESIAN_POINT('Ctrl Pts',(83.8812317852022,52.7276477521024,26.9418937851851)) ;
#15368=CARTESIAN_POINT('Ctrl Pts',(83.8164220957884,52.5959846294495,26.9516005511601)) ;
#15369=CARTESIAN_POINT('Ctrl Pts',(83.7844609400415,52.4481488418597,26.9613073171352)) ;
#15370=CARTESIAN_POINT('Ctrl Pts',(83.7847326912755,52.3002006015805,26.9710140831103)) ;
#15371=CARTESIAN_POINT('Origin',(84.75,52.3,26.4)) ;
#15372=CARTESIAN_POINT('',(83.7829231651454,52.2991702952661,27.4289859168897)) ;
#15373=CARTESIAN_POINT('',(83.7829351910593,52.2991686072217,27.3710140831103)) ;
#15374=CARTESIAN_POINT('',(83.78325,52.3,26.4)) ;
#15375=CARTESIAN_POINT('Ctrl Pts',(83.7829231651454,52.2991702952661,27.4289859168897)) ;
#15376=CARTESIAN_POINT('Ctrl Pts',(83.7852242648531,52.5541918641273,27.4121744158458)) ;
#15377=CARTESIAN_POINT('Ctrl Pts',(83.8890401093448,52.810871192434,27.3953629148018)) ;
#15378=CARTESIAN_POINT('Ctrl Pts',(84.0699842686843,52.9893621083363,27.3785514137579)) ;
#15379=CARTESIAN_POINT('Ctrl Pts',(84.2964678251858,53.2127749976184,27.3575088525586)) ;
#15380=CARTESIAN_POINT('Ctrl Pts',(84.6437878592095,53.3136905607676,27.3364662913593)) ;
#15381=CARTESIAN_POINT('Ctrl Pts',(84.9547283733474,53.2464289555923,27.3154237301601)) ;
#15382=CARTESIAN_POINT('Ctrl Pts',(85.2656688874853,53.1791673504169,27.2943811689608)) ;
#15383=CARTESIAN_POINT('Ctrl Pts',(85.5402298817374,52.9437285769171,27.2733386077615)) ;
#15384=CARTESIAN_POINT('Ctrl Pts',(85.6541300102328,52.6466849747208,27.2522960465622)) ;
#15385=CARTESIAN_POINT('Ctrl Pts',(85.7680301387282,52.3496413725244,27.2312534853629)) ;
#15386=CARTESIAN_POINT('Ctrl Pts',(85.7212694014668,51.9909929416316,27.2102109241636)) ;
#15387=CARTESIAN_POINT('Ctrl Pts',(85.5350143493848,51.7330837735866,27.1891683629643)) ;
#15388=CARTESIAN_POINT('Ctrl Pts',(85.3487592973027,51.4751746055417,27.168125801765)) ;
#15389=CARTESIAN_POINT('Ctrl Pts',(85.0230099303999,51.3180047003446,27.1470832405657)) ;
#15390=CARTESIAN_POINT('Ctrl Pts',(84.7052180283029,51.3327172918697,27.1260406793665)) ;
#15391=CARTESIAN_POINT('Ctrl Pts',(84.387426126206,51.3474298833948,27.1049981181672)) ;
#15392=CARTESIAN_POINT('Ctrl Pts',(84.0775916889149,51.534024971642,27.0839555569679)) ;
#15393=CARTESIAN_POINT('Ctrl Pts',(83.9159630651151,51.8080403409294,27.0629129957686)) ;
#15394=CARTESIAN_POINT('Ctrl Pts',(83.8290980519193,51.9553060176977,27.0516039694756)) ;
#15395=CARTESIAN_POINT('Ctrl Pts',(83.785040401111,52.1278219296783,27.0402949431826)) ;
#15396=CARTESIAN_POINT('Ctrl Pts',(83.7847331702872,52.3001910598074,27.0289859168897)) ;
#15397=CARTESIAN_POINT('Ctrl Pts',(83.7847326912755,52.3002006015805,26.9710140831103)) ;
#15398=CARTESIAN_POINT('Ctrl Pts',(83.7850500489154,52.1274230812518,26.9823498783345)) ;
#15399=CARTESIAN_POINT('Ctrl Pts',(83.8293270681539,51.9544921964693,26.9936856735587)) ;
#15400=CARTESIAN_POINT('Ctrl Pts',(83.9165832441649,51.8069869482407,27.0050214687829)) ;
#15401=CARTESIAN_POINT('Ctrl Pts',(84.0785563027296,51.5331739380657,27.0260640299822)) ;
#15402=CARTESIAN_POINT('Ctrl Pts',(84.3886280129336,51.3469732212317,27.0471065911815)) ;
#15403=CARTESIAN_POINT('Ctrl Pts',(84.7064387677917,51.3326623797936,27.0681491523808)) ;
#15404=CARTESIAN_POINT('Ctrl Pts',(85.0242495226499,51.3183515383555,27.0891917135801)) ;
#15405=CARTESIAN_POINT('Ctrl Pts',(85.3497993221623,51.4759305723135,27.1102342747794)) ;
#15406=CARTESIAN_POINT('Ctrl Pts',(85.5357286216791,51.7340740692188,27.1312768359787)) ;
#15407=CARTESIAN_POINT('Ctrl Pts',(85.7216579211959,51.9922175661241,27.152319397178)) ;
#15408=CARTESIAN_POINT('Ctrl Pts',(85.7679667207172,52.3509255259768,27.1733619583772)) ;
#15409=CARTESIAN_POINT('Ctrl Pts',(85.6536921048407,52.6478254252983,27.1944045195765)) ;
#15410=CARTESIAN_POINT('Ctrl Pts',(85.5394174889643,52.9447253246197,27.2154470807758)) ;
#15411=CARTESIAN_POINT('Ctrl Pts',(85.2645594576901,53.1798171634098,27.2364896419751)) ;
#15412=CARTESIAN_POINT('Ctrl Pts',(84.9535342733738,53.2466863758117,27.2575322031744)) ;
#15413=CARTESIAN_POINT('Ctrl Pts',(84.6425090890574,53.3135555882136,27.2785747643737)) ;
#15414=CARTESIAN_POINT('Ctrl Pts',(84.2953167516988,53.2122021742272,27.299617325573)) ;
#15415=CARTESIAN_POINT('Ctrl Pts',(84.0691152289107,52.9885038104687,27.3206598867723)) ;
#15416=CARTESIAN_POINT('Ctrl Pts',(83.8886841526971,52.8100693948966,27.3374446188849)) ;
#15417=CARTESIAN_POINT('Ctrl Pts',(83.7852341620669,52.5537923176105,27.3542293509976)) ;
#15418=CARTESIAN_POINT('Ctrl Pts',(83.7829351910593,52.2991686072217,27.3710140831103)) ;
#15419=CARTESIAN_POINT('Origin',(84.75,52.3,26.4)) ;
#15420=CARTESIAN_POINT('',(83.782331408344,52.3006703987026,27.8289859168897)) ;
#15421=CARTESIAN_POINT('',(83.7823209222831,52.3006659823901,27.7710140831103)) ;
#15422=CARTESIAN_POINT('',(83.78325,52.3,26.4)) ;
#15423=CARTESIAN_POINT('Ctrl Pts',(83.782331408344,52.3006703987026,27.8289859168897)) ;
#15424=CARTESIAN_POINT('Ctrl Pts',(83.7819893417447,52.3437879615906,27.8261390109074)) ;
#15425=CARTESIAN_POINT('Ctrl Pts',(83.7846250624964,52.3868634658397,27.8232921049252)) ;
#15426=CARTESIAN_POINT('Ctrl Pts',(83.7903820188789,52.4295177032146,27.820445198943)) ;
#15427=CARTESIAN_POINT('Ctrl Pts',(83.8329338656059,52.744791339215,27.7994026377437)) ;
#15428=CARTESIAN_POINT('Ctrl Pts',(84.0460065682424,53.0370501194155,27.7783600765444)) ;
#15429=CARTESIAN_POINT('Ctrl Pts',(84.3331517830637,53.1740017558885,27.7573175153451)) ;
#15430=CARTESIAN_POINT('Ctrl Pts',(84.6202969978849,53.3109533923615,27.7362749541458)) ;
#15431=CARTESIAN_POINT('Ctrl Pts',(84.9815147248909,53.2925978851069,27.7152323929466)) ;
#15432=CARTESIAN_POINT('Ctrl Pts',(85.2532980908674,53.1272439400855,27.6941898317473)) ;
#15433=CARTESIAN_POINT('Ctrl Pts',(85.5250814568439,52.9618899950641,27.673147270548)) ;
#15434=CARTESIAN_POINT('Ctrl Pts',(85.7074304617909,52.6495376122759,27.6521047093487)) ;
#15435=CARTESIAN_POINT('Ctrl Pts',(85.7178039852687,52.3315745397791,27.6310621481494)) ;
#15436=CARTESIAN_POINT('Ctrl Pts',(85.7281775087464,52.0136114672823,27.6100195869501)) ;
#15437=CARTESIAN_POINT('Ctrl Pts',(85.5665755507549,51.6900377050768,27.5889770257508)) ;
#15438=CARTESIAN_POINT('Ctrl Pts',(85.3061479856785,51.5073204152145,27.5679344645515)) ;
#15439=CARTESIAN_POINT('Ctrl Pts',(85.0457204206021,51.3246031253523,27.5468919033522)) ;
#15440=CARTESIAN_POINT('Ctrl Pts',(84.6864672484407,51.2827423078331,27.5258493421529)) ;
#15441=CARTESIAN_POINT('Ctrl Pts',(84.3910060753508,51.4006864487252,27.5048067809536)) ;
#15442=CARTESIAN_POINT('Ctrl Pts',(84.095544902261,51.5186305896173,27.4837642197543)) ;
#15443=CARTESIAN_POINT('Ctrl Pts',(83.8638757282426,51.7963796889206,27.4627216585551)) ;
#15444=CARTESIAN_POINT('Ctrl Pts',(83.8008646807231,52.1082093462798,27.4416790973558)) ;
#15445=CARTESIAN_POINT('Ctrl Pts',(83.7881949524527,52.1709094152505,27.4374480372004)) ;
#15446=CARTESIAN_POINT('Ctrl Pts',(83.7823440323683,52.2349873531273,27.4332169770451)) ;
#15447=CARTESIAN_POINT('Ctrl Pts',(83.7829231651454,52.2991702952661,27.4289859168897)) ;
#15448=CARTESIAN_POINT('Ctrl Pts',(83.7829351910593,52.2991686072217,27.3710140831103)) ;
#15449=CARTESIAN_POINT('Ctrl Pts',(83.7823520047707,52.2345775114,27.3752719121969)) ;
#15450=CARTESIAN_POINT('Ctrl Pts',(83.7882778726445,52.1700928095101,27.3795297412835)) ;
#15451=CARTESIAN_POINT('Ctrl Pts',(83.8011073400004,52.1070121793185,27.3837875703701)) ;
#15452=CARTESIAN_POINT('Ctrl Pts',(83.8645116820959,51.7952622254577,27.4048301315694)) ;
#15453=CARTESIAN_POINT('Ctrl Pts',(84.0965310745045,51.5178056312668,27.4258726927687)) ;
#15454=CARTESIAN_POINT('Ctrl Pts',(84.3921408066335,51.4002343057104,27.446915253968)) ;
#15455=CARTESIAN_POINT('Ctrl Pts',(84.6877505387624,51.2826629801539,27.4679578151673)) ;
#15456=CARTESIAN_POINT('Ctrl Pts',(85.0469506106117,51.3249769232318,27.4890003763666)) ;
#15457=CARTESIAN_POINT('Ctrl Pts',(85.307147479323,51.5080225826629,27.5100429375659)) ;
#15458=CARTESIAN_POINT('Ctrl Pts',(85.5673443480344,51.691068242094,27.5310854987651)) ;
#15459=CARTESIAN_POINT('Ctrl Pts',(85.7285380136077,52.0148456178783,27.5521280599644)) ;
#15460=CARTESIAN_POINT('Ctrl Pts',(85.7177634037076,52.3327953600667,27.5731706211637)) ;
#15461=CARTESIAN_POINT('Ctrl Pts',(85.7069887938075,52.6507451022551,27.594213182363)) ;
#15462=CARTESIAN_POINT('Ctrl Pts',(85.5242459084338,52.9628672108476,27.6152557435623)) ;
#15463=CARTESIAN_POINT('Ctrl Pts',(85.2522541664254,53.1278781829457,27.6362983047616)) ;
#15464=CARTESIAN_POINT('Ctrl Pts',(84.9802624244171,53.2928891550439,27.6573408659609)) ;
#15465=CARTESIAN_POINT('Ctrl Pts',(84.6190218257741,53.3107889906478,27.6783834271602)) ;
#15466=CARTESIAN_POINT('Ctrl Pts',(84.3320495934087,53.1734752405106,27.6994259883595)) ;
#15467=CARTESIAN_POINT('Ctrl Pts',(84.0450773610434,53.0361614903734,27.7204685495587)) ;
#15468=CARTESIAN_POINT('Ctrl Pts',(83.8323734949557,52.7436341544952,27.741511110758)) ;
#15469=CARTESIAN_POINT('Ctrl Pts',(83.7902193849058,52.4283070863173,27.7625536719573)) ;
#15470=CARTESIAN_POINT('Ctrl Pts',(83.7845698650361,52.3860467578464,27.7653738090083)) ;
#15471=CARTESIAN_POINT('Ctrl Pts',(83.7819836790408,52.3433769113913,27.7681939460593)) ;
#15472=CARTESIAN_POINT('Ctrl Pts',(83.7823209222831,52.3006659823901,27.7710140831103)) ;
#15473=CARTESIAN_POINT('Origin',(84.75,52.3,26.4)) ;
#15474=CARTESIAN_POINT('',(83.7847482189314,52.300144797748,28.2289859168897)) ;
#15475=CARTESIAN_POINT('',(83.784746322328,52.3001512320295,28.1710140831103)) ;
#15476=CARTESIAN_POINT('',(83.78325,52.3,26.4)) ;
#15477=CARTESIAN_POINT('Ctrl Pts',(83.7847482189314,52.300144797748,28.2289859168897)) ;
#15478=CARTESIAN_POINT('Ctrl Pts',(83.7845434991546,52.451422798205,28.2190610447698)) ;
#15479=CARTESIAN_POINT('Ctrl Pts',(83.8180233821541,52.6026150775528,28.20913617265)) ;
#15480=CARTESIAN_POINT('Ctrl Pts',(83.8856705962109,52.7365503256865,28.1992113005302)) ;
#15481=CARTESIAN_POINT('Ctrl Pts',(84.0290951788721,53.0205177785228,28.1781687393309)) ;
#15482=CARTESIAN_POINT('Ctrl Pts',(84.3261081608466,53.2269117212532,28.1571261781316)) ;
#15483=CARTESIAN_POINT('Ctrl Pts',(84.6422652431795,53.2623069818343,28.1360836169323)) ;
#15484=CARTESIAN_POINT('Ctrl Pts',(84.9584223255125,53.2977022424154,28.115041055733)) ;
#15485=CARTESIAN_POINT('Ctrl Pts',(85.2937235082039,53.1620988208472,28.0939984945337)) ;
#15486=CARTESIAN_POINT('Ctrl Pts',(85.4963931612999,52.9168782326122,28.0729559333344)) ;
#15487=CARTESIAN_POINT('Ctrl Pts',(85.6990628143959,52.6716576443773,28.0519133721352)) ;
#15488=CARTESIAN_POINT('Ctrl Pts',(85.7691009378964,52.3168198894756,28.0308708109359)) ;
#15489=CARTESIAN_POINT('Ctrl Pts',(85.6748044515052,52.0129839175434,28.0098282497366)) ;
#15490=CARTESIAN_POINT('Ctrl Pts',(85.5805079651139,51.7091479456112,27.9887856885373)) ;
#15491=CARTESIAN_POINT('Ctrl Pts',(85.3218768688308,51.4563137566485,27.967743127338)) ;
#15492=CARTESIAN_POINT('Ctrl Pts',(85.0159817236842,51.3689279148218,27.9467005661387)) ;
#15493=CARTESIAN_POINT('Ctrl Pts',(84.7100865785376,51.2815420729951,27.9256580049394)) ;
#15494=CARTESIAN_POINT('Ctrl Pts',(84.3569273845274,51.3596045783045,27.9046154437401)) ;
#15495=CARTESIAN_POINT('Ctrl Pts',(84.116363282931,51.5677800768593,27.8835728825408)) ;
#15496=CARTESIAN_POINT('Ctrl Pts',(83.9083457603114,51.7477909396278,27.8653772273238)) ;
#15497=CARTESIAN_POINT('Ctrl Pts',(83.7845176856361,52.0250897111043,27.8471815721067)) ;
#15498=CARTESIAN_POINT('Ctrl Pts',(83.782331408344,52.3006703987026,27.8289859168897)) ;
#15499=CARTESIAN_POINT('Ctrl Pts',(83.7823209222831,52.3006659823901,27.7710140831103)) ;
#15500=CARTESIAN_POINT('Ctrl Pts',(83.7845000324795,52.0246876700055,27.7892365072586)) ;
#15501=CARTESIAN_POINT('Ctrl Pts',(83.9087366396395,51.7469941005196,27.8074589314069)) ;
#15502=CARTESIAN_POINT('Ctrl Pts',(84.1172874394612,51.5669813423512,27.8256813555552)) ;
#15503=CARTESIAN_POINT('Ctrl Pts',(84.3581139580789,51.3591094670406,27.8467239167545)) ;
#15504=CARTESIAN_POINT('Ctrl Pts',(84.7113713493266,51.281492516897,27.8677664779538)) ;
#15505=CARTESIAN_POINT('Ctrl Pts',(85.0171560228832,51.369264163824,27.8888090391531)) ;
#15506=CARTESIAN_POINT('Ctrl Pts',(85.3229406964397,51.4570358107511,27.9098516003523)) ;
#15507=CARTESIAN_POINT('Ctrl Pts',(85.5812526523051,51.7101960547489,27.9308941615516)) ;
#15508=CARTESIAN_POINT('Ctrl Pts',(85.675165789644,52.0141507410278,27.9519367227509)) ;
#15509=CARTESIAN_POINT('Ctrl Pts',(85.769078926983,52.3181054273066,27.9729792839502)) ;
#15510=CARTESIAN_POINT('Ctrl Pts',(85.6985932457955,52.6728545558666,27.9940218451495)) ;
#15511=CARTESIAN_POINT('Ctrl Pts',(85.495614415528,52.9178192943447,28.0150644063488)) ;
#15512=CARTESIAN_POINT('Ctrl Pts',(85.2926355852604,53.1627840328228,28.0361069675481)) ;
#15513=CARTESIAN_POINT('Ctrl Pts',(84.9571636059129,53.297964381219,28.0571495287474)) ;
#15514=CARTESIAN_POINT('Ctrl Pts',(84.6410514192883,53.2621703300033,28.0781920899466)) ;
#15515=CARTESIAN_POINT('Ctrl Pts',(84.3249392326637,53.2263762787877,28.0992346511459)) ;
#15516=CARTESIAN_POINT('Ctrl Pts',(84.0281868387621,53.0196078279602,28.1202772123452)) ;
#15517=CARTESIAN_POINT('Ctrl Pts',(83.8851205801658,52.7354596724217,28.1413197735445)) ;
#15518=CARTESIAN_POINT('Ctrl Pts',(83.8178243714495,52.6018006687607,28.1512178767331)) ;
#15519=CARTESIAN_POINT('Ctrl Pts',(83.7845330583397,52.4510204799289,28.1611159799217)) ;
#15520=CARTESIAN_POINT('Ctrl Pts',(83.784746322328,52.3001512320295,28.1710140831103)) ;
#15521=CARTESIAN_POINT('Origin',(84.75,52.3,26.4)) ;
#15522=CARTESIAN_POINT('',(83.7828374094831,52.29918392718,28.6289859168897)) ;
#15523=CARTESIAN_POINT('',(83.7828493504888,52.2991818538181,28.5710140831103)) ;
#15524=CARTESIAN_POINT('',(83.78325,52.3,26.4)) ;
#15525=CARTESIAN_POINT('Ctrl Pts',(83.7828374094831,52.29918392718,28.6289859168897)) ;
#15526=CARTESIAN_POINT('Ctrl Pts',(83.7851495737918,52.5570489842384,28.6119830786322)) ;
#15527=CARTESIAN_POINT('Ctrl Pts',(83.8916037184267,52.8166003859073,28.5949802403748)) ;
#15528=CARTESIAN_POINT('Ctrl Pts',(84.0762274939135,52.9954653946484,28.5779774021174)) ;
#15529=CARTESIAN_POINT('Ctrl Pts',(84.3047162341877,53.2168271364859,28.5569348409181)) ;
#15530=CARTESIAN_POINT('Ctrl Pts',(84.6529320602892,53.3146070398796,28.5358922797188)) ;
#15531=CARTESIAN_POINT('Ctrl Pts',(84.9632534692345,53.2445445796632,28.5148497185195)) ;
#15532=CARTESIAN_POINT('Ctrl Pts',(85.2735748781798,53.1744821194467,28.4938071573202)) ;
#15533=CARTESIAN_POINT('Ctrl Pts',(85.5460018699689,52.93657729562,28.4727645961209)) ;
#15534=CARTESIAN_POINT('Ctrl Pts',(85.6572191077321,52.6385188261787,28.4517220349216)) ;
#15535=CARTESIAN_POINT('Ctrl Pts',(85.7684363454952,52.3404603567374,28.4306794737223)) ;
#15536=CARTESIAN_POINT('Ctrl Pts',(85.7184438292325,51.9822482416814,28.4096369125231)) ;
#15537=CARTESIAN_POINT('Ctrl Pts',(85.5298709024732,51.7260288503878,28.3885943513238)) ;
#15538=CARTESIAN_POINT('Ctrl Pts',(85.3412979757139,51.4698094590941,28.3675517901245)) ;
#15539=CARTESIAN_POINT('Ctrl Pts',(85.0141446384581,51.3155827915627,28.3465092289252)) ;
#15540=CARTESIAN_POINT('Ctrl Pts',(84.6964983607722,51.3331602616194,28.3254666677259)) ;
#15541=CARTESIAN_POINT('Ctrl Pts',(84.3788520830862,51.3507377316761,28.3044241065266)) ;
#15542=CARTESIAN_POINT('Ctrl Pts',(84.07071286497,51.5401193393208,28.2833815453273)) ;
#15543=CARTESIAN_POINT('Ctrl Pts',(83.9115613475859,51.8155806246143,28.262338984128)) ;
#15544=CARTESIAN_POINT('Ctrl Pts',(83.8274747637313,51.9611186555753,28.2512212950486)) ;
#15545=CARTESIAN_POINT('Ctrl Pts',(83.7849775428762,52.1306855086675,28.2401036059691)) ;
#15546=CARTESIAN_POINT('Ctrl Pts',(83.7847482189314,52.300144797748,28.2289859168897)) ;
#15547=CARTESIAN_POINT('Ctrl Pts',(83.784746322328,52.3001512320295,28.1710140831103)) ;
#15548=CARTESIAN_POINT('Ctrl Pts',(83.784986440209,52.1302847468775,28.182158541121)) ;
#15549=CARTESIAN_POINT('Ctrl Pts',(83.8277000620734,51.9603053622059,28.1933029991317)) ;
#15550=CARTESIAN_POINT('Ctrl Pts',(83.9121730740077,51.8145233484151,28.2044474571424)) ;
#15551=CARTESIAN_POINT('Ctrl Pts',(84.0716719497369,51.5392630401967,28.2254900183417)) ;
#15552=CARTESIAN_POINT('Ctrl Pts',(84.3800498244863,51.3502702840097,28.246532579541)) ;
#15553=CARTESIAN_POINT('Ctrl Pts',(84.6977180280713,51.3330935243927,28.2675751407402)) ;
#15554=CARTESIAN_POINT('Ctrl Pts',(85.0153862316564,51.3159167647757,28.2886177019395)) ;
#15555=CARTESIAN_POINT('Ctrl Pts',(85.342344764077,51.4705560017287,28.3096602631388)) ;
#15556=CARTESIAN_POINT('Ctrl Pts',(85.530594334573,51.7270130699661,28.3307028243381)) ;
#15557=CARTESIAN_POINT('Ctrl Pts',(85.7188439050691,51.9834701382036,28.3517453855374)) ;
#15558=CARTESIAN_POINT('Ctrl Pts',(85.7683845136405,52.3417450377255,28.3727879467367)) ;
#15559=CARTESIAN_POINT('Ctrl Pts',(85.6567913748644,52.6396629794784,28.393830507936)) ;
#15560=CARTESIAN_POINT('Ctrl Pts',(85.5451982360883,52.9375809212313,28.4148730691353)) ;
#15561=CARTESIAN_POINT('Ctrl Pts',(85.2724713499645,53.1751419052153,28.4359156303346)) ;
#15562=CARTESIAN_POINT('Ctrl Pts',(84.9620618019187,53.2448128541275,28.4569581915338)) ;
#15563=CARTESIAN_POINT('Ctrl Pts',(84.6516522538729,53.3144838030397,28.4780007527331)) ;
#15564=CARTESIAN_POINT('Ctrl Pts',(84.3035600439051,53.2162647168803,28.4990433139324)) ;
#15565=CARTESIAN_POINT('Ctrl Pts',(84.0753507195849,52.9946149189247,28.5200858751317)) ;
#15566=CARTESIAN_POINT('Ctrl Pts',(83.8912430307036,52.8157991226631,28.5370619444579)) ;
#15567=CARTESIAN_POINT('Ctrl Pts',(83.7851604304188,52.5566491555032,28.5540380137841)) ;
#15568=CARTESIAN_POINT('Ctrl Pts',(83.7828493504888,52.2991818538181,28.5710140831103)) ;
#15569=CARTESIAN_POINT('Origin',(84.75,52.3,26.4)) ;
#15570=CARTESIAN_POINT('',(83.782407671779,52.3007005599052,29.0289859168897)) ;
#15571=CARTESIAN_POINT('',(83.782396840654,52.3006964898307,28.9710140831103)) ;
#15572=CARTESIAN_POINT('',(83.78325,52.3,26.4)) ;
#15573=CARTESIAN_POINT('Ctrl Pts',(83.782407671779,52.3007005599052,29.0289859168897)) ;
#15574=CARTESIAN_POINT('Ctrl Pts',(83.7820311033026,52.3467254751765,29.0259476736939)) ;
#15575=CARTESIAN_POINT('Ctrl Pts',(83.7850347520562,52.3927010359488,29.0229094304982)) ;
#15576=CARTESIAN_POINT('Ctrl Pts',(83.7915888137738,52.4381647684036,29.0198711873024)) ;
#15577=CARTESIAN_POINT('Ctrl Pts',(83.8369815739682,52.7530419230263,28.9988286261032)) ;
#15578=CARTESIAN_POINT('Ctrl Pts',(84.0526807466604,53.0433676675877,28.9777860649039)) ;
#15579=CARTESIAN_POINT('Ctrl Pts',(84.3410491044655,53.1777247120556,28.9567435037046)) ;
#15580=CARTESIAN_POINT('Ctrl Pts',(84.6294174622707,53.3120817565235,28.9357009425053)) ;
#15581=CARTESIAN_POINT('Ctrl Pts',(84.9904550051888,53.2904701008978,28.914658381306)) ;
#15582=CARTESIAN_POINT('Ctrl Pts',(85.2607364208631,53.122672360977,28.8936158201067)) ;
#15583=CARTESIAN_POINT('Ctrl Pts',(85.5310178365373,52.9548746210563,28.8725732589074)) ;
#15584=CARTESIAN_POINT('Ctrl Pts',(85.7105431249676,52.6408907968403,28.8515306977081)) ;
#15585=CARTESIAN_POINT('Ctrl Pts',(85.71804933466,52.3228471174543,28.8304881365088)) ;
#15586=CARTESIAN_POINT('Ctrl Pts',(85.7255555443523,52.0048034380682,28.8094455753095)) ;
#15587=CARTESIAN_POINT('Ctrl Pts',(85.5610426753067,51.6826999035119,28.7884030141103)) ;
#15588=CARTESIAN_POINT('Ctrl Pts',(85.2989782380021,51.5023381673217,28.767360452911)) ;
#15589=CARTESIAN_POINT('Ctrl Pts',(85.0369138006973,51.3219764311315,28.7463178917117)) ;
#15590=CARTESIAN_POINT('Ctrl Pts',(84.6772977951335,51.2833564933073,28.7252753305124)) ;
#15591=CARTESIAN_POINT('Ctrl Pts',(84.3829120682143,51.4039598471894,28.7042327693131)) ;
#15592=CARTESIAN_POINT('Ctrl Pts',(84.0885263412951,51.5245632010715,28.6831902081138)) ;
#15593=CARTESIAN_POINT('Ctrl Pts',(83.8593708930204,51.80438984666,28.6621476469145)) ;
#15594=CARTESIAN_POINT('Ctrl Pts',(83.7991739961065,52.1167749595949,28.6411050857152)) ;
#15595=CARTESIAN_POINT('Ctrl Pts',(83.7876174758146,52.1767462385407,28.6370653627734)) ;
#15596=CARTESIAN_POINT('Ctrl Pts',(83.7822880598356,52.2379174861818,28.6330256398315)) ;
#15597=CARTESIAN_POINT('Ctrl Pts',(83.7828374094831,52.29918392718,28.6289859168897)) ;
#15598=CARTESIAN_POINT('Ctrl Pts',(83.7828493504888,52.2991818538181,28.5710140831103)) ;
#15599=CARTESIAN_POINT('Ctrl Pts',(83.7822957483815,52.237507465609,28.5750805749834)) ;
#15600=CARTESIAN_POINT('Ctrl Pts',(83.7876966245727,52.175929629855,28.5791470668565)) ;
#15601=CARTESIAN_POINT('Ctrl Pts',(83.799405866669,52.115575677217,28.5832135587296)) ;
#15602=CARTESIAN_POINT('Ctrl Pts',(83.8599967767458,51.8032667432166,28.6042561199289)) ;
#15603=CARTESIAN_POINT('Ctrl Pts',(84.0895050355717,51.5237293849677,28.6252986811282)) ;
#15604=CARTESIAN_POINT('Ctrl Pts',(84.3840426691043,51.4034974795791,28.6463412423274)) ;
#15605=CARTESIAN_POINT('Ctrl Pts',(84.678580302637,51.2832655741904,28.6673838035267)) ;
#15606=CARTESIAN_POINT('Ctrl Pts',(85.0381473108762,51.3223391216621,28.688426364726)) ;
#15607=CARTESIAN_POINT('Ctrl Pts',(85.2999840257837,51.5030313001503,28.7094689259253)) ;
#15608=CARTESIAN_POINT('Ctrl Pts',(85.5618207406912,51.6837234786386,28.7305114871246)) ;
#15609=CARTESIAN_POINT('Ctrl Pts',(85.7259271622669,52.0060342881435,28.7515540483239)) ;
#15610=CARTESIAN_POINT('Ctrl Pts',(85.7180197603577,52.3240682511654,28.7725966095232)) ;
#15611=CARTESIAN_POINT('Ctrl Pts',(85.7101123584486,52.6421022141873,28.7936391707225)) ;
#15612=CARTESIAN_POINT('Ctrl Pts',(85.5301911330546,52.9558593307262,28.8146817319218)) ;
#15613=CARTESIAN_POINT('Ctrl Pts',(85.2596982583662,53.1233159919349,28.835724293121)) ;
#15614=CARTESIAN_POINT('Ctrl Pts',(84.9892053836778,53.2907726531436,28.8567668543203)) ;
#15615=CARTESIAN_POINT('Ctrl Pts',(84.628140859695,53.3119288590221,28.8778094155196)) ;
#15616=CARTESIAN_POINT('Ctrl Pts',(84.3399422118783,53.1772081552049,28.8988519767189)) ;
#15617=CARTESIAN_POINT('Ctrl Pts',(84.0517435640616,53.0424874513877,28.9198945379182)) ;
#15618=CARTESIAN_POINT('Ctrl Pts',(83.836410792411,52.7518898378748,28.9409370991175)) ;
#15619=CARTESIAN_POINT('Ctrl Pts',(83.7914152711865,52.4369556674358,28.9619796603168)) ;
#15620=CARTESIAN_POINT('Ctrl Pts',(83.784975805339,52.3918843407893,28.9649911345813)) ;
#15621=CARTESIAN_POINT('Ctrl Pts',(83.7820250967013,52.3463145656929,28.9680026088458)) ;
#15622=CARTESIAN_POINT('Ctrl Pts',(83.782396840654,52.3006964898307,28.9710140831103)) ;
#15623=CARTESIAN_POINT('Origin',(84.75,52.3,26.4)) ;
#15624=CARTESIAN_POINT('',(83.7847592665387,52.3000985915647,29.4289859168897)) ;
#15625=CARTESIAN_POINT('',(83.784757957323,52.3001050761132,29.3710140831103)) ;
#15626=CARTESIAN_POINT('',(83.78325,52.3,26.4)) ;
#15627=CARTESIAN_POINT('Ctrl Pts',(83.7847592665387,52.3000985915647,29.4289859168897)) ;
#15628=CARTESIAN_POINT('Ctrl Pts',(83.7846172807008,52.4542974257026,29.4188697075563)) ;
#15629=CARTESIAN_POINT('Ctrl Pts',(83.8194624052769,52.6084356653519,29.408753498223)) ;
#15630=CARTESIAN_POINT('Ctrl Pts',(83.8896418563525,52.7443257473643,29.3986372888896)) ;
#15631=CARTESIAN_POINT('Ctrl Pts',(84.035620982083,53.0269884793123,29.3775947276903)) ;
#15632=CARTESIAN_POINT('Ctrl Pts',(84.3344828276875,53.2306960351298,29.3565521664911)) ;
#15633=CARTESIAN_POINT('Ctrl Pts',(84.6509461975464,53.2632392482302,29.3355096052918)) ;
#15634=CARTESIAN_POINT('Ctrl Pts',(84.9674095674054,53.2957824613305,29.3144670440925)) ;
#15635=CARTESIAN_POINT('Ctrl Pts',(85.3014744615188,53.1571613317139,29.2934244828932)) ;
#15636=CARTESIAN_POINT('Ctrl Pts',(85.5019248616669,52.9101233543463,29.2723819216939)) ;
#15637=CARTESIAN_POINT('Ctrl Pts',(85.702375261815,52.6630853769787,29.2513393604946)) ;
#15638=CARTESIAN_POINT('Ctrl Pts',(85.7692111679977,52.3076305518603,29.2302967992953)) ;
#15639=CARTESIAN_POINT('Ctrl Pts',(85.6721789983957,52.004657148335,29.209254238096)) ;
#15640=CARTESIAN_POINT('Ctrl Pts',(85.5751468287936,51.7016837448097,29.1882116768967)) ;
#15641=CARTESIAN_POINT('Ctrl Pts',(85.3142465834066,51.4511917628776,29.1671691156975)) ;
#15642=CARTESIAN_POINT('Ctrl Pts',(85.0075759640742,51.3665675558227,29.1461265544982)) ;
#15643=CARTESIAN_POINT('Ctrl Pts',(84.7009053447418,51.2819433487679,29.1250839932989)) ;
#15644=CARTESIAN_POINT('Ctrl Pts',(84.3484643514639,51.3631869165903,29.1040414320996)) ;
#15645=CARTESIAN_POINT('Ctrl Pts',(84.1097870286733,51.5735229828435,29.0829988709003)) ;
#15646=CARTESIAN_POINT('Ctrl Pts',(83.9055712785534,51.7534895462563,29.0649945528968)) ;
#15647=CARTESIAN_POINT('Ctrl Pts',(83.7846391780019,52.0279616258427,29.0469902348932)) ;
#15648=CARTESIAN_POINT('Ctrl Pts',(83.782407671779,52.3007005599052,29.0289859168897)) ;
#15649=CARTESIAN_POINT('Ctrl Pts',(83.782396840654,52.3006964898307,28.9710140831103)) ;
#15650=CARTESIAN_POINT('Ctrl Pts',(83.7846226433473,52.0275600060296,28.9890451700451)) ;
#15651=CARTESIAN_POINT('Ctrl Pts',(83.9059573682543,51.7526919543628,29.0070762569799)) ;
#15652=CARTESIAN_POINT('Ctrl Pts',(84.1107039457943,51.5727159480407,29.0251073439146)) ;
#15653=CARTESIAN_POINT('Ctrl Pts',(84.3496464124251,51.3626811264497,29.0461499051139)) ;
#15654=CARTESIAN_POINT('Ctrl Pts',(84.7021896164851,51.2818822106329,29.0671924663132)) ;
#15655=CARTESIAN_POINT('Ctrl Pts',(85.0087532473587,51.3668932032513,29.0882350275125)) ;
#15656=CARTESIAN_POINT('Ctrl Pts',(85.3153168782323,51.4519041958698,29.1092775887118)) ;
#15657=CARTESIAN_POINT('Ctrl Pts',(85.5759009359194,51.7027250969235,29.1303201499111)) ;
#15658=CARTESIAN_POINT('Ctrl Pts',(85.6725508424044,52.0058206663679,29.1513627111104)) ;
#15659=CARTESIAN_POINT('Ctrl Pts',(85.7692007488893,52.3089162358123,29.1724052723097)) ;
#15660=CARTESIAN_POINT('Ctrl Pts',(85.7019165041721,52.6642864736473,29.1934478335089)) ;
#15661=CARTESIAN_POINT('Ctrl Pts',(85.5011546325818,52.9110713993538,29.2144903947082)) ;
#15662=CARTESIAN_POINT('Ctrl Pts',(85.3003927609915,53.1578563250602,29.2355329559075)) ;
#15663=CARTESIAN_POINT('Ctrl Pts',(84.9661532625282,53.296055938638,29.2565755171068)) ;
#15664=CARTESIAN_POINT('Ctrl Pts',(84.6497311908775,53.2631135463041,29.2776180783061)) ;
#15665=CARTESIAN_POINT('Ctrl Pts',(84.3333091192268,53.2301711539701,29.2986606395054)) ;
#15666=CARTESIAN_POINT('Ctrl Pts',(84.0347044743889,53.0260867557244,29.3197032007047)) ;
#15667=CARTESIAN_POINT('Ctrl Pts',(83.8890820288675,52.7432400976202,29.340745761904)) ;
#15668=CARTESIAN_POINT('Ctrl Pts',(83.8192593028512,52.6076214116222,29.3508352023061)) ;
#15669=CARTESIAN_POINT('Ctrl Pts',(83.7846070216412,52.4538953659082,29.3609246427082)) ;
#15670=CARTESIAN_POINT('Ctrl Pts',(83.784757957323,52.3001050761132,29.3710140831103)) ;
#15671=CARTESIAN_POINT('Origin',(84.75,52.3,26.4)) ;
#15672=CARTESIAN_POINT('',(83.7827524248469,52.2992003133627,29.8289859168897)) ;
#15673=CARTESIAN_POINT('',(83.7827642412961,52.2991978560061,29.7710140831103)) ;
#15674=CARTESIAN_POINT('',(83.78325,52.3,26.4)) ;
#15675=CARTESIAN_POINT('Ctrl Pts',(83.7827524248469,52.2992003133627,29.8289859168897)) ;
#15676=CARTESIAN_POINT('Ctrl Pts',(83.7850677815131,52.5599079824122,29.8117917414187)) ;
#15677=CARTESIAN_POINT('Ctrl Pts',(83.8942008215872,52.8223250596572,29.7945975659478)) ;
#15678=CARTESIAN_POINT('Ctrl Pts',(84.0825254981447,53.001512148494,29.7774033904768)) ;
#15679=CARTESIAN_POINT('Ctrl Pts',(84.3130008436182,53.2208047391355,29.7563608292775)) ;
#15680=CARTESIAN_POINT('Ctrl Pts',(84.6620841409586,53.3154410037131,29.7353182680783)) ;
#15681=CARTESIAN_POINT('Ctrl Pts',(84.971761222317,53.2425833996989,29.714275706879)) ;
#15682=CARTESIAN_POINT('Ctrl Pts',(85.2814383036755,53.1697257956847,29.6932331456797)) ;
#15683=CARTESIAN_POINT('Ctrl Pts',(85.551709169052,52.9293743230787,29.6721905844804)) ;
#15684=CARTESIAN_POINT('Ctrl Pts',(85.6602344621622,52.6303251867537,29.6511480232811)) ;
#15685=CARTESIAN_POINT('Ctrl Pts',(85.7687597552723,52.3312760504287,29.6301054620818)) ;
#15686=CARTESIAN_POINT('Ctrl Pts',(85.7155394761161,51.9735292503846,29.6090629008825)) ;
#15687=CARTESIAN_POINT('Ctrl Pts',(85.524664030014,51.7190205290081,29.5880203396832)) ;
#15688=CARTESIAN_POINT('Ctrl Pts',(85.3337885839119,51.4645118076316,29.566977778484)) ;
#15689=CARTESIAN_POINT('Ctrl Pts',(85.005257970864,51.3132411649226,29.5459352172847)) ;
#15690=CARTESIAN_POINT('Ctrl Pts',(84.6877830911888,51.333681956409,29.5248926560854)) ;
#15691=CARTESIAN_POINT('Ctrl Pts',(84.3703082115136,51.3541227478954,29.5038500948861)) ;
#15692=CARTESIAN_POINT('Ctrl Pts',(84.063889065211,51.5462749735772,29.4828075336868)) ;
#15693=CARTESIAN_POINT('Ctrl Pts',(83.9072276949881,51.8231600404575,29.4617649724875)) ;
#15694=CARTESIAN_POINT('Ctrl Pts',(83.8258812638838,51.9669326372676,29.4508386206216)) ;
#15695=CARTESIAN_POINT('Ctrl Pts',(83.7849126231147,52.1335509585936,29.4399122687556)) ;
#15696=CARTESIAN_POINT('Ctrl Pts',(83.7847592665387,52.3000985915647,29.4289859168897)) ;
#15697=CARTESIAN_POINT('Ctrl Pts',(83.784757957323,52.3001050761132,29.3710140831103)) ;
#15698=CARTESIAN_POINT('Ctrl Pts',(83.7849218134627,52.1331499671655,29.3819672039075)) ;
#15699=CARTESIAN_POINT('Ctrl Pts',(83.8261023948951,51.9661191444747,29.3929203247047)) ;
#15700=CARTESIAN_POINT('Ctrl Pts',(83.9078298636839,51.8220972916435,29.4038734455018)) ;
#15701=CARTESIAN_POINT('Ctrl Pts',(84.0648403902266,51.5454100617337,29.4249160067011)) ;
#15702=CARTESIAN_POINT('Ctrl Pts',(84.3715016895169,51.3536445198768,29.4459585679004)) ;
#15703=CARTESIAN_POINT('Ctrl Pts',(84.689002107179,51.3336042248495,29.4670011290997)) ;
#15704=CARTESIAN_POINT('Ctrl Pts',(85.006502524841,51.3135639298222,29.488043690299)) ;
#15705=CARTESIAN_POINT('Ctrl Pts',(85.3348420608748,51.4652488816244,29.5090862514983)) ;
#15706=CARTESIAN_POINT('Ctrl Pts',(85.5253963068553,51.7199981858024,29.5301288126976)) ;
#15707=CARTESIAN_POINT('Ctrl Pts',(85.7159505528357,51.9747474899804,29.5511713738969)) ;
#15708=CARTESIAN_POINT('Ctrl Pts',(85.7687195087629,52.3325611465344,29.5722139350961)) ;
#15709=CARTESIAN_POINT('Ctrl Pts',(85.6598170628616,52.6314731501694,29.5932564962954)) ;
#15710=CARTESIAN_POINT('Ctrl Pts',(85.5509146169603,52.9303851538044,29.6142990574947)) ;
#15711=CARTESIAN_POINT('Ctrl Pts',(85.2803407692306,53.1703955045205,29.635341618694)) ;
#15712=CARTESIAN_POINT('Ctrl Pts',(84.9705720223194,53.242862407845,29.6563841798933)) ;
#15713=CARTESIAN_POINT('Ctrl Pts',(84.6608032754083,53.3153293111694,29.6774267410926)) ;
#15714=CARTESIAN_POINT('Ctrl Pts',(84.3118396293156,53.2202527671022,29.6984693022919)) ;
#15715=CARTESIAN_POINT('Ctrl Pts',(84.0816410911999,53.0006696127169,29.7195118634912)) ;
#15716=CARTESIAN_POINT('Ctrl Pts',(83.8938354409632,52.8215244390423,29.7366792700309)) ;
#15717=CARTESIAN_POINT('Ctrl Pts',(83.7850796413422,52.5595078807163,29.7538466765706)) ;
#15718=CARTESIAN_POINT('Ctrl Pts',(83.7827642412961,52.2991978560061,29.7710140831103)) ;
#15719=CARTESIAN_POINT('Origin',(84.75,52.3,26.4)) ;
#15720=CARTESIAN_POINT('',(83.7824862293435,52.3007282075195,30.2289859168897)) ;
#15721=CARTESIAN_POINT('',(83.7824750955529,52.3007244933117,30.1710140831103)) ;
#15722=CARTESIAN_POINT('',(83.78325,52.3,26.4)) ;
#15723=CARTESIAN_POINT('Ctrl Pts',(83.7824862293435,52.3007282075195,30.2289859168897)) ;
#15724=CARTESIAN_POINT('Ctrl Pts',(83.782075295683,52.3496619525008,30.2257563364804)) ;
#15725=CARTESIAN_POINT('Ctrl Pts',(83.7854712604975,52.3985385126902,30.2225267560711)) ;
#15726=CARTESIAN_POINT('Ctrl Pts',(83.7928735252652,52.4468006010654,30.2192971756619)) ;
#15727=CARTESIAN_POINT('Ctrl Pts',(83.8411035086217,52.761255675579,30.1982546144626)) ;
#15728=CARTESIAN_POINT('Ctrl Pts',(84.0594116156069,53.0496247818971,30.1772120532633)) ;
#15729=CARTESIAN_POINT('Ctrl Pts',(84.3489796726717,53.1813763113338,30.156169492064)) ;
#15730=CARTESIAN_POINT('Ctrl Pts',(84.6385477297366,53.3131278407706,30.1351269308647)) ;
#15731=CARTESIAN_POINT('Ctrl Pts',(84.999375736881,53.288261793326,30.1140843696654)) ;
#15732=CARTESIAN_POINT('Ctrl Pts',(85.2681332290841,53.1180339002943,30.0930418084661)) ;
#15733=CARTESIAN_POINT('Ctrl Pts',(85.5368907212873,52.9478060072626,30.0719992472669)) ;
#15734=CARTESIAN_POINT('Ctrl Pts',(85.7135776985492,52.6322162686438,30.0509566860676)) ;
#15735=CARTESIAN_POINT('Ctrl Pts',(85.7182159840437,52.3141178381398,30.0299141248683)) ;
#15736=CARTESIAN_POINT('Ctrl Pts',(85.7228542695383,51.9960194076358,30.008871563669)) ;
#15737=CARTESIAN_POINT('Ctrl Pts',(85.5554438632655,51.6754122852466,29.9878290024697)) ;
#15738=CARTESIAN_POINT('Ctrl Pts',(85.2917638593211,51.4974207666249,29.9667864412704)) ;
#15739=CARTESIAN_POINT('Ctrl Pts',(85.0280838553767,51.3194292480032,29.9457438800711)) ;
#15740=CARTESIAN_POINT('Ctrl Pts',(84.6681342537607,51.284053333149,29.9247013188718)) ;
#15741=CARTESIAN_POINT('Ctrl Pts',(84.3748479051717,51.407306093413,29.9036587576725)) ;
#15742=CARTESIAN_POINT('Ctrl Pts',(84.0815615565827,51.530558853677,29.8826161964733)) ;
#15743=CARTESIAN_POINT('Ctrl Pts',(83.8549384610206,51.8124402890592,29.861573635274)) ;
#15744=CARTESIAN_POINT('Ctrl Pts',(83.7975606100427,52.125355465103,29.8405310740747)) ;
#15745=CARTESIAN_POINT('Ctrl Pts',(83.7870670156207,52.1825832087348,29.8366826883464)) ;
#15746=CARTESIAN_POINT('Ctrl Pts',(83.7822342036874,52.240848944637,29.832834302618)) ;
#15747=CARTESIAN_POINT('Ctrl Pts',(83.7827524248469,52.2992003133627,29.8289859168897)) ;
#15748=CARTESIAN_POINT('Ctrl Pts',(83.7827642412961,52.2991978560061,29.7710140831103)) ;
#15749=CARTESIAN_POINT('Ctrl Pts',(83.7822415919806,52.2404387415845,29.7748892377699)) ;
#15750=CARTESIAN_POINT('Ctrl Pts',(83.7871423870742,52.1817665799574,29.7787643924295)) ;
#15751=CARTESIAN_POINT('Ctrl Pts',(83.7977816579324,52.1241541408295,29.782639547089)) ;
#15752=CARTESIAN_POINT('Ctrl Pts',(83.855554192919,51.8113115880308,29.8036821082883)) ;
#15753=CARTESIAN_POINT('Ctrl Pts',(84.0825326930308,51.5297162471369,29.8247246694876)) ;
#15754=CARTESIAN_POINT('Ctrl Pts',(84.3759742911983,51.4068335506118,29.8457672306869)) ;
#15755=CARTESIAN_POINT('Ctrl Pts',(84.6694158893658,51.2839508540868,29.8668097918862)) ;
#15756=CARTESIAN_POINT('Ctrl Pts',(85.0293205855891,51.3197808019306,29.8878523530855)) ;
#15757=CARTESIAN_POINT('Ctrl Pts',(85.2927758558033,51.4981048026616,29.9088949142848)) ;
#15758=CARTESIAN_POINT('Ctrl Pts',(85.5562311260175,51.6764288033927,29.9299374754841)) ;
#15759=CARTESIAN_POINT('Ctrl Pts',(85.7232369702226,51.997246857011,29.9509800366833)) ;
#15760=CARTESIAN_POINT('Ctrl Pts',(85.7181974212124,52.3153391888679,29.9720225978826)) ;
#15761=CARTESIAN_POINT('Ctrl Pts',(85.7131578722021,52.6334315207248,29.9930651590819)) ;
#15762=CARTESIAN_POINT('Ctrl Pts',(85.5360729299765,52.9487981308203,30.0141077202812)) ;
#15763=CARTESIAN_POINT('Ctrl Pts',(85.2671009120418,53.1186868656103,30.0351502814805)) ;
#15764=CARTESIAN_POINT('Ctrl Pts',(84.9981288941072,53.2885756004003,30.0561928426798)) ;
#15765=CARTESIAN_POINT('Ctrl Pts',(84.6372698004635,53.3129864598848,30.0772354038791)) ;
#15766=CARTESIAN_POINT('Ctrl Pts',(84.3478681675789,53.1808697557022,30.0982779650784)) ;
#15767=CARTESIAN_POINT('Ctrl Pts',(84.0584665346943,53.0487530515197,30.1193205262777)) ;
#15768=CARTESIAN_POINT('Ctrl Pts',(83.8405223625687,52.76010878367,30.140363087477)) ;
#15769=CARTESIAN_POINT('Ctrl Pts',(83.7926890879558,52.4455931139805,30.1614056486763)) ;
#15770=CARTESIAN_POINT('Ctrl Pts',(83.7854085597202,52.397721831233,30.1646084601543)) ;
#15771=CARTESIAN_POINT('Ctrl Pts',(83.7820689521351,52.3492511915763,30.1678112716323)) ;
#15772=CARTESIAN_POINT('Ctrl Pts',(83.7824750955529,52.3007244933117,30.1710140831103)) ;
#15773=CARTESIAN_POINT('Origin',(84.75,52.3,26.4)) ;
#15774=CARTESIAN_POINT('',(83.7847661033277,52.3000521019819,30.6289859168897)) ;
#15775=CARTESIAN_POINT('',(83.7847653843543,52.3000586182133,30.5710140831103)) ;
#15776=CARTESIAN_POINT('',(83.78325,52.3,26.4)) ;
#15777=CARTESIAN_POINT('Ctrl Pts',(83.7847661033277,52.3000521019819,30.6289859168897)) ;
#15778=CARTESIAN_POINT('Ctrl Pts',(83.784689680815,52.4571702230074,30.6186783703428)) ;
#15779=CARTESIAN_POINT('Ctrl Pts',(83.8209307306342,52.6142551143286,30.6083708237959)) ;
#15780=CARTESIAN_POINT('Ctrl Pts',(83.8936830616376,52.7520650464375,30.5980632772491)) ;
#15781=CARTESIAN_POINT('Ctrl Pts',(84.0422048626859,53.033400077726,30.5770207160498)) ;
#15782=CARTESIAN_POINT('Ctrl Pts',(84.3428912751165,53.2344046855717,30.5559781548505)) ;
#15783=CARTESIAN_POINT('Ctrl Pts',(84.6596352047527,53.2640932054744,30.5349355936512)) ;
#15784=CARTESIAN_POINT('Ctrl Pts',(84.9763791343889,53.2937817253771,30.5138930324519)) ;
#15785=CARTESIAN_POINT('Ctrl Pts',(85.3091805812308,53.1521541573367,30.4928504712526)) ;
#15786=CARTESIAN_POINT('Ctrl Pts',(85.5073954322809,52.9033188744703,30.4718079100534)) ;
#15787=CARTESIAN_POINT('Ctrl Pts',(85.705610283331,52.6544835916039,30.4507653488541)) ;
#15788=CARTESIAN_POINT('Ctrl Pts',(85.7692385385893,52.2984405939114,30.4297227876548)) ;
#15789=CARTESIAN_POINT('Ctrl Pts',(85.6694785742636,51.9963543898182,30.4086802264555)) ;
#15790=CARTESIAN_POINT('Ctrl Pts',(85.5697186099378,51.694268185725,30.3876376652562)) ;
#15791=CARTESIAN_POINT('Ctrl Pts',(85.306570426028,51.446138775231,30.3665951040569)) ;
#15792=CARTESIAN_POINT('Ctrl Pts',(84.999149264129,51.3642830827168,30.3455525428576)) ;
#15793=CARTESIAN_POINT('Ctrl Pts',(84.6917281022299,51.2824273902026,30.3245099816583)) ;
#15794=CARTESIAN_POINT('Ctrl Pts',(84.3400339623416,51.3668454156681,30.303467420459)) ;
#15795=CARTESIAN_POINT('Ctrl Pts',(84.1032628222613,51.5793249497555,30.2824248592598)) ;
#15796=CARTESIAN_POINT('Ctrl Pts',(83.9028309580058,51.7591934468992,30.2646118784697)) ;
#15797=CARTESIAN_POINT('Ctrl Pts',(83.7847527632191,52.0308306515281,30.2467988976797)) ;
#15798=CARTESIAN_POINT('Ctrl Pts',(83.7824862293435,52.3007282075195,30.2289859168897)) ;
#15799=CARTESIAN_POINT('Ctrl Pts',(83.7824750955529,52.3007244933117,30.1710140831103)) ;
#15800=CARTESIAN_POINT('Ctrl Pts',(83.7847373257758,52.0304294235648,30.1888538328316)) ;
#15801=CARTESIAN_POINT('Ctrl Pts',(83.9032122760979,51.7583951236067,30.2066935825528)) ;
#15802=CARTESIAN_POINT('Ctrl Pts',(84.104172425537,51.5785096804386,30.2245333322741)) ;
#15803=CARTESIAN_POINT('Ctrl Pts',(84.3412114148312,51.3663289881155,30.2455758934734)) ;
#15804=CARTESIAN_POINT('Ctrl Pts',(84.69301177052,51.2823546749988,30.2666184546727)) ;
#15805=CARTESIAN_POINT('Ctrl Pts',(85.0003294357354,51.3645981020112,30.287661015872)) ;
#15806=CARTESIAN_POINT('Ctrl Pts',(85.3076471009508,51.4468415290236,30.3087035770713)) ;
#15807=CARTESIAN_POINT('Ctrl Pts',(85.5704820756929,51.6953026961652,30.3297461382705)) ;
#15808=CARTESIAN_POINT('Ctrl Pts',(85.6698608939394,51.997514507855,30.3507886994698)) ;
#15809=CARTESIAN_POINT('Ctrl Pts',(85.7692397121858,52.2997263195448,30.3718312606691)) ;
#15810=CARTESIAN_POINT('Ctrl Pts',(85.7051623739367,52.6556887757828,30.3928738218684)) ;
#15811=CARTESIAN_POINT('Ctrl Pts',(85.5066337824851,52.9042738256472,30.4139163830677)) ;
#15812=CARTESIAN_POINT('Ctrl Pts',(85.3081051910334,53.1528588755117,30.434958944267)) ;
#15813=CARTESIAN_POINT('Ctrl Pts',(84.9751253463793,53.2940665190026,30.4560015054663)) ;
#15814=CARTESIAN_POINT('Ctrl Pts',(84.6584191140949,53.2639784637058,30.4770440666656)) ;
#15815=CARTESIAN_POINT('Ctrl Pts',(84.3417128818105,53.233890408409,30.4980866278649)) ;
#15816=CARTESIAN_POINT('Ctrl Pts',(84.0412802618958,53.0325066543245,30.5191291890641)) ;
#15817=CARTESIAN_POINT('Ctrl Pts',(83.8931134682116,52.7509844884226,30.5401717502634)) ;
#15818=CARTESIAN_POINT('Ctrl Pts',(83.8207235228308,52.6134410233427,30.5504525278791)) ;
#15819=CARTESIAN_POINT('Ctrl Pts',(83.7846796237543,52.456768417478,30.5607333054947)) ;
#15820=CARTESIAN_POINT('Ctrl Pts',(83.7847653843543,52.3000586182133,30.5710140831103)) ;
#15821=CARTESIAN_POINT('Origin',(84.75,52.3,26.4)) ;
#15822=CARTESIAN_POINT('',(83.7826684881877,52.2992194180186,31.0289859168897)) ;
#15823=CARTESIAN_POINT('',(83.782680142622,52.2992165895442,30.9710140831103)) ;
#15824=CARTESIAN_POINT('',(83.78325,52.3,26.4)) ;
#15825=CARTESIAN_POINT('Ctrl Pts',(83.7826684881877,52.2992194180186,31.0289859168897)) ;
#15826=CARTESIAN_POINT('Ctrl Pts',(83.7849787270906,52.5627690272941,31.0116004042052)) ;
#15827=CARTESIAN_POINT('Ctrl Pts',(83.8968315418767,52.8280450612531,30.9942148915207)) ;
#15828=CARTESIAN_POINT('Ctrl Pts',(84.0888777674471,53.007501874752,30.9768293788363)) ;
#15829=CARTESIAN_POINT('Ctrl Pts',(84.3213209819787,53.2247074900949,30.955786817637)) ;
#15830=CARTESIAN_POINT('Ctrl Pts',(84.6712433690026,53.3161924146107,30.9347442564377)) ;
#15831=CARTESIAN_POINT('Ctrl Pts',(84.9802509462634,53.2405455880425,30.9137016952384)) ;
#15832=CARTESIAN_POINT('Ctrl Pts',(85.2892585235242,53.1648987614744,30.8926591340391)) ;
#15833=CARTESIAN_POINT('Ctrl Pts',(85.5573512910218,52.9221201838222,30.8716165728398)) ;
#15834=CARTESIAN_POINT('Ctrl Pts',(85.6631758168593,52.6221046935596,30.8505740116405)) ;
#15835=CARTESIAN_POINT('Ctrl Pts',(85.7690003426968,52.3220892032969,30.8295314504413)) ;
#15836=CARTESIAN_POINT('Ctrl Pts',(85.7125566268742,51.9648368004238,30.808488889242)) ;
#15837=CARTESIAN_POINT('Ctrl Pts',(85.5193941790459,51.7120594394717,30.7874463280427)) ;
#15838=CARTESIAN_POINT('Ctrl Pts',(85.3262317312177,51.4592820785195,30.7664037668434)) ;
#15839=CARTESIAN_POINT('Ctrl Pts',(84.9963505513838,51.3109797594882,30.7453612056441)) ;
#15840=CARTESIAN_POINT('Ctrl Pts',(84.6790728797514,51.3342822108441,30.7243186444448)) ;
#15841=CARTESIAN_POINT('Ctrl Pts',(84.361795208119,51.3575846622,30.7032760832455)) ;
#15842=CARTESIAN_POINT('Ctrl Pts',(84.0571210446882,51.552491883943,30.6822335220462)) ;
#15843=CARTESIAN_POINT('Ctrl Pts',(83.9029625578057,51.8307782221802,30.6611909608469)) ;
#15844=CARTESIAN_POINT('Ctrl Pts',(83.824317491751,51.9727480085695,30.6504559461945)) ;
#15845=CARTESIAN_POINT('Ctrl Pts',(83.7848456951869,52.1364180767848,30.6397209315421)) ;
#15846=CARTESIAN_POINT('Ctrl Pts',(83.7847661033277,52.3000521019819,30.6289859168897)) ;
#15847=CARTESIAN_POINT('Ctrl Pts',(83.7847653843543,52.3000586182133,30.5710140831103)) ;
#15848=CARTESIAN_POINT('Ctrl Pts',(83.7848551574291,52.1360168493726,30.581775866694)) ;
#15849=CARTESIAN_POINT('Ctrl Pts',(83.8245344699275,51.9719343253853,30.5925376502777)) ;
#15850=CARTESIAN_POINT('Ctrl Pts',(83.9035551198438,51.8297100872491,30.6032994338613)) ;
#15851=CARTESIAN_POINT('Ctrl Pts',(84.0580645326141,51.5516184296964,30.6243419950606)) ;
#15852=CARTESIAN_POINT('Ctrl Pts',(84.3629843256084,51.3570956923101,30.6453845562599)) ;
#15853=CARTESIAN_POINT('Ctrl Pts',(84.6802911452845,51.3341934910749,30.6664271174592)) ;
#15854=CARTESIAN_POINT('Ctrl Pts',(84.9975979649606,51.3112912898398,30.6874696786584)) ;
#15855=CARTESIAN_POINT('Ctrl Pts',(85.3272918113186,51.4600096247557,30.7085122398577)) ;
#15856=CARTESIAN_POINT('Ctrl Pts',(85.5201352411866,51.7130304543972,30.729554801057)) ;
#15857=CARTESIAN_POINT('Ctrl Pts',(85.7129786710545,51.9660512840388,30.7505973622563)) ;
#15858=CARTESIAN_POINT('Ctrl Pts',(85.7689716844323,52.323374608406,30.7716399234556)) ;
#15859=CARTESIAN_POINT('Ctrl Pts',(85.6627687848767,52.6232563729606,30.7926824846549)) ;
#15860=CARTESIAN_POINT('Ctrl Pts',(85.5565658853211,52.9231381375152,30.8137250458542)) ;
#15861=CARTESIAN_POINT('Ctrl Pts',(85.288167072832,53.1655783422572,30.8347676070535)) ;
#15862=CARTESIAN_POINT('Ctrl Pts',(84.9790643106336,53.2408353088181,30.8558101682527)) ;
#15863=CARTESIAN_POINT('Ctrl Pts',(84.6699615484351,53.3160922753791,30.876852729452)) ;
#15864=CARTESIAN_POINT('Ctrl Pts',(84.3201548365273,53.224166003759,30.8978952906514)) ;
#15865=CARTESIAN_POINT('Ctrl Pts',(84.0879857990347,53.006667344109,30.9189378518507)) ;
#15866=CARTESIAN_POINT('Ctrl Pts',(83.8964614503065,52.8272451025016,30.9362965956039)) ;
#15867=CARTESIAN_POINT('Ctrl Pts',(83.7849916140278,52.5623686358697,30.9536553393571)) ;
#15868=CARTESIAN_POINT('Ctrl Pts',(83.782680142622,52.2992165895442,30.9710140831103)) ;
#15869=CARTESIAN_POINT('Origin',(84.75,52.3,26.4)) ;
#15870=CARTESIAN_POINT('',(83.7825667404007,52.3007531219363,31.4289859168897)) ;
#15871=CARTESIAN_POINT('',(83.7825553766487,52.3007499079334,31.3710140831103)) ;
#15872=CARTESIAN_POINT('',(83.78325,52.3,26.4)) ;
#15873=CARTESIAN_POINT('Ctrl Pts',(83.7825667404007,52.3007531219363,31.4289859168897)) ;
#15874=CARTESIAN_POINT('Ctrl Pts',(83.7821217885114,52.3525970280063,31.4255649992669)) ;
#15875=CARTESIAN_POINT('Ctrl Pts',(83.7859345114109,52.4043754474013,31.4221440816441)) ;
#15876=CARTESIAN_POINT('Ctrl Pts',(83.7942359163689,52.4554239704382,31.4187231640213)) ;
#15877=CARTESIAN_POINT('Ctrl Pts',(83.8452990640768,52.7694308506349,31.397680602822)) ;
#15878=CARTESIAN_POINT('Ctrl Pts',(84.0661986252004,53.0558209430958,31.3766380416228)) ;
#15879=CARTESIAN_POINT('Ctrl Pts',(84.3569429082262,53.1849565172998,31.3555954804235)) ;
#15880=CARTESIAN_POINT('Ctrl Pts',(84.6476871912519,53.3140920915038,31.3345529192242)) ;
#15881=CARTESIAN_POINT('Ctrl Pts',(85.0082761961798,53.2859731474509,31.3135103580249)) ;
#15882=CARTESIAN_POINT('Ctrl Pts',(85.2754878820815,53.1133288069547,31.2924677968256)) ;
#15883=CARTESIAN_POINT('Ctrl Pts',(85.5426995679832,52.9406844664586,31.2714252356263)) ;
#15884=CARTESIAN_POINT('Ctrl Pts',(85.7165339348589,52.6235147295192,31.250382674427)) ;
#15885=CARTESIAN_POINT('Ctrl Pts',(85.7183039355651,52.3053874743441,31.2293401132277)) ;
#15886=CARTESIAN_POINT('Ctrl Pts',(85.7200739362713,51.9872602191691,31.2082975520285)) ;
#15887=CARTESIAN_POINT('Ctrl Pts',(85.5497795708082,51.6681754457583,31.1872549908292)) ;
#15888=CARTESIAN_POINT('Ctrl Pts',(85.2845054286732,51.4925685825908,31.1662124296299)) ;
#15889=CARTESIAN_POINT('Ctrl Pts',(85.0192312865381,51.3169617194232,31.1451698684306)) ;
#15890=CARTESIAN_POINT('Ctrl Pts',(84.6589773677312,51.2848327664989,31.1241273072313)) ;
#15891=CARTESIAN_POINT('Ctrl Pts',(84.3668142449798,51.4107249289525,31.103084746032)) ;
#15892=CARTESIAN_POINT('Ctrl Pts',(84.0746511222284,51.5366170914061,31.0820421848327)) ;
#15893=CARTESIAN_POINT('Ctrl Pts',(83.8505787955325,51.8205303692377,31.0609996236334)) ;
#15894=CARTESIAN_POINT('Ctrl Pts',(83.7960246532043,52.1339501612384,31.0399570624342)) ;
#15895=CARTESIAN_POINT('Ctrl Pts',(83.7865435285784,52.1884203074339,31.0363000139193)) ;
#15896=CARTESIAN_POINT('Ctrl Pts',(83.7821825286476,52.2437816679403,31.0326429654045)) ;
#15897=CARTESIAN_POINT('Ctrl Pts',(83.7826684881877,52.2992194180186,31.0289859168897)) ;
#15898=CARTESIAN_POINT('Ctrl Pts',(83.782680142622,52.2992165895442,30.9710140831103)) ;
#15899=CARTESIAN_POINT('Ctrl Pts',(83.7821896095044,52.2433712983756,30.9746979005564)) ;
#15900=CARTESIAN_POINT('Ctrl Pts',(83.7866151303081,52.1876036681652,30.9783817180024)) ;
#15901=CARTESIAN_POINT('Ctrl Pts',(83.7962348619755,52.1327468994487,30.9820655354485)) ;
#15902=CARTESIAN_POINT('Ctrl Pts',(83.8511843254861,51.8193961621186,31.0031080966478)) ;
#15903=CARTESIAN_POINT('Ctrl Pts',(84.0756146155844,51.5357657351382,31.0241506578471)) ;
#15904=CARTESIAN_POINT('Ctrl Pts',(84.3679363214755,51.4102422357509,31.0451932190464)) ;
#15905=CARTESIAN_POINT('Ctrl Pts',(84.6602580273666,51.2847187363636,31.0662357802457)) ;
#15906=CARTESIAN_POINT('Ctrl Pts',(85.0204711490505,51.3173021645692,31.0872783414449)) ;
#15907=CARTESIAN_POINT('Ctrl Pts',(85.2855235578632,51.4932434938774,31.1083209026442)) ;
#15908=CARTESIAN_POINT('Ctrl Pts',(85.550575966676,51.6691848231856,31.1293634638435)) ;
#15909=CARTESIAN_POINT('Ctrl Pts',(85.7204676626176,51.9884840535963,31.1504060250428)) ;
#15910=CARTESIAN_POINT('Ctrl Pts',(85.718296372969,52.3066088866807,31.1714485862421)) ;
#15911=CARTESIAN_POINT('Ctrl Pts',(85.7161250833204,52.6247337197652,31.1924911474414)) ;
#15912=CARTESIAN_POINT('Ctrl Pts',(85.5418908080815,52.9416841555234,31.2135337086407)) ;
#15913=CARTESIAN_POINT('Ctrl Pts',(85.2744615202819,53.113991167422,31.23457626984)) ;
#15914=CARTESIAN_POINT('Ctrl Pts',(85.0070322324822,53.2862981793206,31.2556188310392)) ;
#15915=CARTESIAN_POINT('Ctrl Pts',(84.6464079321218,53.3139617673597,31.2766613922386)) ;
#15916=CARTESIAN_POINT('Ctrl Pts',(84.3558268285061,53.1844597729726,31.2977039534378)) ;
#15917=CARTESIAN_POINT('Ctrl Pts',(84.0652457248903,53.0549577785855,31.3187465146371)) ;
#15918=CARTESIAN_POINT('Ctrl Pts',(83.8447078180192,52.7682902017724,31.3397890758364)) ;
#15919=CARTESIAN_POINT('Ctrl Pts',(83.7940407058406,52.4542186643746,31.3608316370357)) ;
#15920=CARTESIAN_POINT('Ctrl Pts',(83.7858681402068,52.4035591706175,31.3642257857272)) ;
#15921=CARTESIAN_POINT('Ctrl Pts',(83.7821151774617,52.3521866960117,31.3676199344188)) ;
#15922=CARTESIAN_POINT('Ctrl Pts',(83.7825553766487,52.3007499079334,31.3710140831103)) ;
#15923=CARTESIAN_POINT('Origin',(84.75,52.3,26.4)) ;
#15924=CARTESIAN_POINT('',(83.7847843561952,52.3000678891362,31.8289859168897)) ;
#15925=CARTESIAN_POINT('',(83.7847716506988,52.3000190203057,31.7710140831103)) ;
#15926=CARTESIAN_POINT('',(83.78325,52.3,26.4)) ;
#15927=CARTESIAN_POINT('Ctrl Pts',(83.7847843561952,52.3000678891362,31.8289859168897)) ;
#15928=CARTESIAN_POINT('Ctrl Pts',(83.7847679988345,52.4600707944189,31.8184870331293)) ;
#15929=CARTESIAN_POINT('Ctrl Pts',(83.8224240277508,52.6200556305873,31.8079881493689)) ;
#15930=CARTESIAN_POINT('Ctrl Pts',(83.8977846402365,52.7597306844102,31.7974892656085)) ;
#15931=CARTESIAN_POINT('Ctrl Pts',(84.0488273926318,53.0396767182138,31.7764467044092)) ;
#15932=CARTESIAN_POINT('Ctrl Pts',(84.3513326348141,53.2380366447095,31.75540414321)) ;
#15933=CARTESIAN_POINT('Ctrl Pts',(84.668336119238,53.264886980438,31.7343615820107)) ;
#15934=CARTESIAN_POINT('Ctrl Pts',(84.9853396036619,53.2917373161665,31.7133190208114)) ;
#15935=CARTESIAN_POINT('Ctrl Pts',(85.3168413303273,53.1470780611279,31.6922764596121)) ;
#15936=CARTESIAN_POINT('Ctrl Pts',(85.5128021802699,52.8964563788972,31.6712338984128)) ;
#15937=CARTESIAN_POINT('Ctrl Pts',(85.7087630302126,52.6458346966665,31.6501913372135)) ;
#15938=CARTESIAN_POINT('Ctrl Pts',(85.7691830034324,52.2892505872438,31.6291487760142)) ;
#15939=CARTESIAN_POINT('Ctrl Pts',(85.666704506489,51.9880807358278,31.608106214815)) ;
#15940=CARTESIAN_POINT('Ctrl Pts',(85.5642260095456,51.6869108844117,31.5870636536157)) ;
#15941=CARTESIAN_POINT('Ctrl Pts',(85.298849042439,51.4411552910024,31.5660210924164)) ;
#15942=CARTESIAN_POINT('Ctrl Pts',(84.9907017630098,51.3620725037616,31.5449785312171)) ;
#15943=CARTESIAN_POINT('Ctrl Pts',(84.6825544835806,51.2829897165209,31.5239359700178)) ;
#15944=CARTESIAN_POINT('Ctrl Pts',(84.3316368918287,51.3705797354487,31.5028934088185)) ;
#15945=CARTESIAN_POINT('Ctrl Pts',(84.0967914630988,51.5851865788789,31.4818508476192)) ;
#15946=CARTESIAN_POINT('Ctrl Pts',(83.9001251732181,51.7649044976337,31.4642292040427)) ;
#15947=CARTESIAN_POINT('Ctrl Pts',(83.7848587522135,52.0336976312407,31.4466075604662)) ;
#15948=CARTESIAN_POINT('Ctrl Pts',(83.7825667404007,52.3007531219363,31.4289859168897)) ;
#15949=CARTESIAN_POINT('Ctrl Pts',(83.7825553766487,52.3007499079334,31.3710140831103)) ;
#15950=CARTESIAN_POINT('Ctrl Pts',(83.7848442618873,52.0332961996321,31.388662495618)) ;
#15951=CARTESIAN_POINT('Ctrl Pts',(83.900501333443,51.7641036837555,31.4063109081258)) ;
#15952=CARTESIAN_POINT('Ctrl Pts',(84.097693462439,51.5843621896236,31.4239593206336)) ;
#15953=CARTESIAN_POINT('Ctrl Pts',(84.3328096487019,51.3700527502527,31.4450018818329)) ;
#15954=CARTESIAN_POINT('Ctrl Pts',(84.6838383387137,51.2829093694934,31.4660444430321)) ;
#15955=CARTESIAN_POINT('Ctrl Pts',(84.9918851656152,51.3623788006393,31.4870870042314)) ;
#15956=CARTESIAN_POINT('Ctrl Pts',(85.2999319925168,51.4418482317852,31.5081295654307)) ;
#15957=CARTESIAN_POINT('Ctrl Pts',(85.5649969563081,51.6879304748365,31.52917212663)) ;
#15958=CARTESIAN_POINT('Ctrl Pts',(85.6670963806458,51.9892334402438,31.5502146878293)) ;
#15959=CARTESIAN_POINT('Ctrl Pts',(85.7691958049835,52.2905364056511,31.5712572490286)) ;
#15960=CARTESIAN_POINT('Ctrl Pts',(85.7083296898676,52.6470600934144,31.5922998102279)) ;
#15961=CARTESIAN_POINT('Ctrl Pts',(85.5120509779309,52.8974261121282,31.6133423714272)) ;
#15962=CARTESIAN_POINT('Ctrl Pts',(85.3157722659941,53.1477921308421,31.6343849326264)) ;
#15963=CARTESIAN_POINT('Ctrl Pts',(84.9840809572364,53.2920004805065,31.6554274938257)) ;
#15964=CARTESIAN_POINT('Ctrl Pts',(84.6671153793743,53.2647670691806,31.676470055025)) ;
#15965=CARTESIAN_POINT('Ctrl Pts',(84.3501498015122,53.2375336578548,31.6975126162243)) ;
#15966=CARTESIAN_POINT('Ctrl Pts',(84.0479099545456,53.0388584855388,31.7185551774236)) ;
#15967=CARTESIAN_POINT('Ctrl Pts',(83.8972127505983,52.7586880401527,31.7395977386229)) ;
#15968=CARTESIAN_POINT('Ctrl Pts',(83.8222162513974,52.619257433392,31.750069853452)) ;
#15969=CARTESIAN_POINT('Ctrl Pts',(83.7847521621177,52.4596429764979,31.7605419682812)) ;
#15970=CARTESIAN_POINT('Ctrl Pts',(83.7847716506988,52.3000190203057,31.7710140831103)) ;
#15971=CARTESIAN_POINT('Origin',(84.75,52.3,25.7604774406976)) ;
#15972=CARTESIAN_POINT('',(84.012172416957,52.3000518747697,31.9604774406976)) ;
#15973=CARTESIAN_POINT('',(84.0115563622989,52.2999794994122,32.0395225593024)) ;
#15974=CARTESIAN_POINT('',(84.011,52.2999999999999,25.7604774406976)) ;
#15975=CARTESIAN_POINT('',(84.6290678012582,51.5698174568242,32.05)) ;
#15976=CARTESIAN_POINT('Ctrl Pts',(84.0121728877458,52.3000518956002,31.9604774406976)) ;
#15977=CARTESIAN_POINT('Ctrl Pts',(84.012185444936,52.1772211438289,31.9710211181365)) ;
#15978=CARTESIAN_POINT('Ctrl Pts',(84.0944207311608,51.8295445255366,32.0008619712373)) ;
#15979=CARTESIAN_POINT('Ctrl Pts',(84.4090991301214,51.6076008033498,32.0307028243381)) ;
#15980=CARTESIAN_POINT('Ctrl Pts',(84.6290682970003,51.5698134220425,32.05)) ;
#15981=CARTESIAN_POINT('',(84.0209858286879,52.1789242467453,32.05)) ;
#15982=CARTESIAN_POINT('Origin',(84.75,52.3,32.05)) ;
#15983=CARTESIAN_POINT('Ctrl Pts',(84.0115565511623,52.299979492453,32.0395225593024)) ;
#15984=CARTESIAN_POINT('Ctrl Pts',(84.0112610663628,52.2594454132586,32.0430150395349)) ;
#15985=CARTESIAN_POINT('Ctrl Pts',(84.0143436429872,52.2189177828097,32.0465075197675)) ;
#15986=CARTESIAN_POINT('Ctrl Pts',(84.0209858286879,52.1789242467453,32.05)) ;
#15987=CARTESIAN_POINT('Origin',(84.75,52.3,25.7604774406976)) ;
#15988=CARTESIAN_POINT('',(84.0104777048421,52.3005756991061,31.5604774406976)) ;
#15989=CARTESIAN_POINT('',(84.0121631754502,52.3000145394422,31.6395225593024)) ;
#15990=CARTESIAN_POINT('',(84.011,52.2999999999999,25.7604774406976)) ;
#15991=CARTESIAN_POINT('Ctrl Pts',(84.0104777048421,52.3005756991061,31.5604774406976)) ;
#15992=CARTESIAN_POINT('Ctrl Pts',(84.0122297573166,52.0964339792985,31.5780990842741)) ;
#15993=CARTESIAN_POINT('Ctrl Pts',(84.2055581925249,51.6456057548941,31.6167632890499)) ;
#15994=CARTESIAN_POINT('Ctrl Pts',(84.9666908338978,51.4556249045992,31.676470055025)) ;
#15995=CARTESIAN_POINT('Ctrl Pts',(85.5752667181236,52.0192040621772,31.7395977386228)) ;
#15996=CARTESIAN_POINT('Ctrl Pts',(85.4367085793821,52.836940778588,31.8027254222208)) ;
#15997=CARTESIAN_POINT('Ctrl Pts',(84.6764920518234,53.1686806993748,31.8658531058186)) ;
#15998=CARTESIAN_POINT('Ctrl Pts',(84.0986379054398,52.7897679070709,31.9184371119776)) ;
#15999=CARTESIAN_POINT('Ctrl Pts',(84.0121603839034,52.4223608141459,31.9499785569372)) ;
#16000=CARTESIAN_POINT('Ctrl Pts',(84.0121728877458,52.3000518956002,31.9604774406976)) ;
#16001=CARTESIAN_POINT('Ctrl Pts',(84.0121631754502,52.3000145394422,31.6395225593024)) ;
#16002=CARTESIAN_POINT('Ctrl Pts',(84.0121782127345,52.1768495541185,31.6500930056725)) ;
#16003=CARTESIAN_POINT('Ctrl Pts',(84.09953271401,51.8084782135297,31.681706013242)) ;
#16004=CARTESIAN_POINT('Ctrl Pts',(84.6793843110363,51.4310793972544,31.7343615820107)) ;
#16005=CARTESIAN_POINT('Ctrl Pts',(85.4385697001617,51.7654585545426,31.7974892656085)) ;
#16006=CARTESIAN_POINT('Ctrl Pts',(85.5742157004875,52.583371203896,31.8606169492065)) ;
#16007=CARTESIAN_POINT('Ctrl Pts',(84.9640410903861,53.1455422795452,31.9237446328042)) ;
#16008=CARTESIAN_POINT('Ctrl Pts',(84.203885152176,52.9519357106028,31.9833798361696)) ;
#16009=CARTESIAN_POINT('Ctrl Pts',(84.0130413933977,52.5036675091086,32.0219724783357)) ;
#16010=CARTESIAN_POINT('Ctrl Pts',(84.0115565511623,52.299979492453,32.0395225593024)) ;
#16011=CARTESIAN_POINT('Origin',(84.75,52.3,25.7604774406976)) ;
#16012=CARTESIAN_POINT('',(84.010555482566,52.2994033099723,31.1604774406976)) ;
#16013=CARTESIAN_POINT('',(84.0104690181984,52.3005732422681,31.2395225593024)) ;
#16014=CARTESIAN_POINT('',(84.011,52.2999999999999,25.7604774406976)) ;
#16015=CARTESIAN_POINT('Ctrl Pts',(84.010555482566,52.2994033099723,31.1604774406976)) ;
#16016=CARTESIAN_POINT('Ctrl Pts',(84.0101840069,52.2570257590979,31.1641344892124)) ;
#16017=CARTESIAN_POINT('Ctrl Pts',(84.0326992015831,51.9712032804197,31.1888340989266)) ;
#16018=CARTESIAN_POINT('Ctrl Pts',(84.4050365955573,51.4994291370381,31.2345762698399)) ;
#16019=CARTESIAN_POINT('Ctrl Pts',(85.2311891044738,51.5731088770259,31.2977039534378)) ;
#16020=CARTESIAN_POINT('Ctrl Pts',(85.6217167571572,52.3048502193085,31.3608316370357)) ;
#16021=CARTESIAN_POINT('Ctrl Pts',(85.2230709941749,53.0321999030888,31.4239593206336)) ;
#16022=CARTESIAN_POINT('Ctrl Pts',(84.3961500488167,53.0966836878991,31.4870870042314)) ;
#16023=CARTESIAN_POINT('Ctrl Pts',(84.0309796581042,52.6232505066463,31.5325930442528)) ;
#16024=CARTESIAN_POINT('Ctrl Pts',(84.0101375761158,52.3402060550262,31.5570565230748)) ;
#16025=CARTESIAN_POINT('Ctrl Pts',(84.0104777048421,52.3005756991061,31.5604774406976)) ;
#16026=CARTESIAN_POINT('Ctrl Pts',(84.0104690181984,52.3005732422681,31.2395225593024)) ;
#16027=CARTESIAN_POINT('Ctrl Pts',(84.0122186806669,52.0961271182085,31.2571709718101)) ;
#16028=CARTESIAN_POINT('Ctrl Pts',(84.2060421944615,51.6450017472081,31.2958619455172)) ;
#16029=CARTESIAN_POINT('Ctrl Pts',(84.9677571597911,51.4559049037231,31.3555954804235)) ;
#16030=CARTESIAN_POINT('Ctrl Pts',(85.5756175422327,52.0202331507826,31.4187231640214)) ;
#16031=CARTESIAN_POINT('Ctrl Pts',(85.4360362883285,52.8378313051878,31.4818508476192)) ;
#16032=CARTESIAN_POINT('Ctrl Pts',(84.6753850015265,53.1685371869628,31.5449785312171)) ;
#16033=CARTESIAN_POINT('Ctrl Pts',(84.0983317306906,52.7892154027258,31.5975357684448)) ;
#16034=CARTESIAN_POINT('Ctrl Pts',(84.0121482780501,52.4220337829137,31.6290504444732)) ;
#16035=CARTESIAN_POINT('Ctrl Pts',(84.0121631754502,52.3000145394422,31.6395225593024)) ;
#16036=CARTESIAN_POINT('Origin',(84.75,52.3,25.7604774406976)) ;
#16037=CARTESIAN_POINT('',(84.0121589349461,52.3000398276334,30.7604774406976)) ;
#16038=CARTESIAN_POINT('',(84.0105643914121,52.2994011478387,30.8395225593024)) ;
#16039=CARTESIAN_POINT('',(84.011,52.2999999999999,25.7604774406976)) ;
#16040=CARTESIAN_POINT('Ctrl Pts',(84.0121589349461,52.3000398276334,30.7604774406976)) ;
#16041=CARTESIAN_POINT('Ctrl Pts',(84.0122197763053,52.1749552198024,30.77121245535)) ;
#16042=CARTESIAN_POINT('Ctrl Pts',(84.1015370120932,51.8046007047638,30.8029900312018)) ;
#16043=CARTESIAN_POINT('Ctrl Pts',(84.6861477792349,51.4306114595269,30.8558101682528)) ;
#16044=CARTESIAN_POINT('Ctrl Pts',(85.4426479868293,51.7707058389346,30.9189378518506)) ;
#16045=CARTESIAN_POINT('Ctrl Pts',(85.5720875709808,52.5899751196893,30.9820655354485)) ;
#16046=CARTESIAN_POINT('Ctrl Pts',(84.9572836759283,53.14672723415,31.0451932190464)) ;
#16047=CARTESIAN_POINT('Ctrl Pts',(84.2013112353611,52.9490831729925,31.1046638541294)) ;
#16048=CARTESIAN_POINT('Ctrl Pts',(84.0123214681354,52.5008650749111,31.1430919280131)) ;
#16049=CARTESIAN_POINT('Ctrl Pts',(84.010555482566,52.2994033099723,31.1604774406976)) ;
#16050=CARTESIAN_POINT('Ctrl Pts',(84.0105643914121,52.2994011478387,30.8395225593024)) ;
#16051=CARTESIAN_POINT('Ctrl Pts',(84.0101894196264,52.2567120656835,30.8432063767484)) ;
#16052=CARTESIAN_POINT('Ctrl Pts',(84.0328962784322,51.9705745100615,30.8679327553938)) ;
#16053=CARTESIAN_POINT('Ctrl Pts',(84.406046739384,51.4989945619123,30.9137016952384)) ;
#16054=CARTESIAN_POINT('Ctrl Pts',(85.2321056902744,51.5737165276034,30.9768293788363)) ;
#16055=CARTESIAN_POINT('Ctrl Pts',(85.6217099208433,52.3059496735259,31.0399570624342)) ;
#16056=CARTESIAN_POINT('Ctrl Pts',(85.2221470677742,53.0327964447449,31.103084746032)) ;
#16057=CARTESIAN_POINT('Ctrl Pts',(84.3951451811447,53.0962359841114,31.1662124296299)) ;
#16058=CARTESIAN_POINT('Ctrl Pts',(84.0307871030694,52.6226228587488,31.21169170072)) ;
#16059=CARTESIAN_POINT('Ctrl Pts',(84.0101325225179,52.339892390331,31.2361284106108)) ;
#16060=CARTESIAN_POINT('Ctrl Pts',(84.0104690181984,52.3005732422681,31.2395225593024)) ;
#16061=CARTESIAN_POINT('Origin',(84.75,52.3,25.7604774406976)) ;
#16062=CARTESIAN_POINT('',(84.0104161608325,52.3005566541059,30.3604774406976)) ;
#16063=CARTESIAN_POINT('',(84.0121583853507,52.3000448087505,30.4395225593024)) ;
#16064=CARTESIAN_POINT('',(84.011,52.2999999999999,25.7604774406976)) ;
#16065=CARTESIAN_POINT('Ctrl Pts',(84.0104161608325,52.3005566541059,30.3604774406976)) ;
#16066=CARTESIAN_POINT('Ctrl Pts',(84.0121487375422,52.0942424116672,30.3782904214876)) ;
#16067=CARTESIAN_POINT('Ctrl Pts',(84.2090354168613,51.6413074113017,30.4171459634769)) ;
#16068=CARTESIAN_POINT('Ctrl Pts',(84.9742969091548,51.4576197781646,30.4770440666656)) ;
#16069=CARTESIAN_POINT('Ctrl Pts',(85.5777616350177,52.0266426931532,30.5401717502634)) ;
#16070=CARTESIAN_POINT('Ctrl Pts',(85.4318461016247,52.8431385047737,30.6032994338613)) ;
#16071=CARTESIAN_POINT('Ctrl Pts',(84.6686489900153,53.1679260075878,30.6664271174592)) ;
#16072=CARTESIAN_POINT('Ctrl Pts',(84.096359217492,52.7853584004575,30.7188197864046)) ;
#16073=CARTESIAN_POINT('Ctrl Pts',(84.0121005162889,52.4201435684535,30.7501698941507)) ;
#16074=CARTESIAN_POINT('Ctrl Pts',(84.0121589349461,52.3000398276334,30.7604774406976)) ;
#16075=CARTESIAN_POINT('Ctrl Pts',(84.0121583853507,52.3000448087505,30.4395225593024)) ;
#16076=CARTESIAN_POINT('Ctrl Pts',(84.0122270094027,52.1746485148035,30.450284342886)) ;
#16077=CARTESIAN_POINT('Ctrl Pts',(84.1018659252076,51.8039722448119,30.482088687669)) ;
#16078=CARTESIAN_POINT('Ctrl Pts',(84.6872445240728,51.4305315890238,30.5349355936513)) ;
#16079=CARTESIAN_POINT('Ctrl Pts',(85.4433151290645,51.7715799971008,30.5980632772491)) ;
#16080=CARTESIAN_POINT('Ctrl Pts',(85.5717211395724,52.5910119186134,30.661190960847)) ;
#16081=CARTESIAN_POINT('Ctrl Pts',(84.9562154066652,53.1469880592007,30.7243186444448)) ;
#16082=CARTESIAN_POINT('Ctrl Pts',(84.2008330365987,52.9484799043716,30.7837625105966)) ;
#16083=CARTESIAN_POINT('Ctrl Pts',(84.0123313191275,52.5005590089554,30.8221638155492)) ;
#16084=CARTESIAN_POINT('Ctrl Pts',(84.0105643914121,52.2994011478387,30.8395225593024)) ;
#16085=CARTESIAN_POINT('Origin',(84.75,52.3,25.7604774406976)) ;
#16086=CARTESIAN_POINT('',(84.0106196451636,52.2993887060512,29.9604774406976)) ;
#16087=CARTESIAN_POINT('',(84.0104076499753,52.3005538149027,30.0395225593024)) ;
#16088=CARTESIAN_POINT('',(84.011,52.2999999999999,25.7604774406976)) ;
#16089=CARTESIAN_POINT('Ctrl Pts',(84.0106196451636,52.2993887060512,29.9604774406976)) ;
#16090=CARTESIAN_POINT('Ctrl Pts',(84.0102235081717,52.2547839359573,29.9643258264259)) ;
#16091=CARTESIAN_POINT('Ctrl Pts',(84.0341177346705,51.9667084407867,29.9892167733536)) ;
#16092=CARTESIAN_POINT('Ctrl Pts',(84.4122688988207,51.4963512925987,30.0351502814805)) ;
#16093=CARTESIAN_POINT('Ctrl Pts',(85.237723532162,51.5774771299215,30.0982779650784)) ;
#16094=CARTESIAN_POINT('Ctrl Pts',(85.6216375437542,52.3127095998846,30.1614056486762)) ;
#16095=CARTESIAN_POINT('Ctrl Pts',(85.2164500303437,53.036435951597,30.2245333322741)) ;
#16096=CARTESIAN_POINT('Ctrl Pts',(84.3889809930133,53.0934600293675,30.2876610158719)) ;
#16097=CARTESIAN_POINT('Ctrl Pts',(84.029611953797,52.6187597073854,30.3329757186798)) ;
#16098=CARTESIAN_POINT('Ctrl Pts',(84.0101020362138,52.3379624338227,30.3572478602883)) ;
#16099=CARTESIAN_POINT('Ctrl Pts',(84.0104161608325,52.3005566541059,30.3604774406976)) ;
#16100=CARTESIAN_POINT('Ctrl Pts',(84.0104076499753,52.3005538149027,30.0395225593024)) ;
#16101=CARTESIAN_POINT('Ctrl Pts',(84.0121369369003,52.093935706247,30.0573623090236)) ;
#16102=CARTESIAN_POINT('Ctrl Pts',(84.2095246450093,51.6407071811469,30.0962446199442)) ;
#16103=CARTESIAN_POINT('Ctrl Pts',(84.975359359988,51.4579033746375,30.156169492064)) ;
#16104=CARTESIAN_POINT('Ctrl Pts',(85.5781058187447,52.0276870907513,30.2192971756619)) ;
#16105=CARTESIAN_POINT('Ctrl Pts',(85.4311604255217,52.8439982006345,30.2824248592598)) ;
#16106=CARTESIAN_POINT('Ctrl Pts',(84.6675542030255,53.1678227112312,30.3455525428576)) ;
#16107=CARTESIAN_POINT('Ctrl Pts',(84.0960396207762,52.7847293170448,30.3979184428719)) ;
#16108=CARTESIAN_POINT('Ctrl Pts',(84.0120928285021,52.4198364215321,30.4292417816868)) ;
#16109=CARTESIAN_POINT('Ctrl Pts',(84.0121583853507,52.3000448087505,30.4395225593024)) ;
#16110=CARTESIAN_POINT('Origin',(84.75,52.3,25.7604774406976)) ;
#16111=CARTESIAN_POINT('',(84.0121537087894,52.3000753650543,29.5604774406976)) ;
#16112=CARTESIAN_POINT('',(84.0106286778565,52.2993868276063,29.6395225593024)) ;
#16113=CARTESIAN_POINT('',(84.011,52.2999999999999,25.7604774406976)) ;
#16114=CARTESIAN_POINT('Ctrl Pts',(84.0121537087894,52.3000753650543,29.5604774406976)) ;
#16115=CARTESIAN_POINT('Ctrl Pts',(84.0122709371417,52.1727635463156,29.5714037925636)) ;
#16116=CARTESIAN_POINT('Ctrl Pts',(84.1039002651515,51.8001096205179,29.6033727056288)) ;
#16117=CARTESIAN_POINT('Ctrl Pts',(84.6939891568927,51.4300710793027,29.6563841798933)) ;
#16118=CARTESIAN_POINT('Ctrl Pts',(85.4473921764194,51.7769725687113,29.7195118634912)) ;
#16119=CARTESIAN_POINT('Ctrl Pts',(85.5694396125602,52.5973756260661,29.7826395470891)) ;
#16120=CARTESIAN_POINT('Ctrl Pts',(84.9496407932796,53.1485617804674,29.8457672306869)) ;
#16121=CARTESIAN_POINT('Ctrl Pts',(84.1979075099158,52.9447673553597,29.9050465285564)) ;
#16122=CARTESIAN_POINT('Ctrl Pts',(84.0123895428375,52.4986780439644,29.9432832652267)) ;
#16123=CARTESIAN_POINT('Ctrl Pts',(84.0106196451636,52.2993887060512,29.9604774406976)) ;
#16124=CARTESIAN_POINT('Ctrl Pts',(84.0106286778565,52.2993868276063,29.6395225593024)) ;
#16125=CARTESIAN_POINT('Ctrl Pts',(84.0102291559076,52.2544703698276,29.6433977139619)) ;
#16126=CARTESIAN_POINT('Ctrl Pts',(84.0343180016969,51.9660794808919,29.6683154298208)) ;
#16127=CARTESIAN_POINT('Ctrl Pts',(84.4132829291257,51.4959258854032,29.714275706879)) ;
#16128=CARTESIAN_POINT('Ctrl Pts',(85.2386345831491,51.5780929341436,29.7774033904768)) ;
#16129=CARTESIAN_POINT('Ctrl Pts',(85.6216208325441,52.3138091222706,29.8405310740747)) ;
#16130=CARTESIAN_POINT('Ctrl Pts',(85.2155206857491,53.0370237843669,29.9036587576725)) ;
#16131=CARTESIAN_POINT('Ctrl Pts',(84.3879803592861,53.0930040020832,29.9667864412704)) ;
#16132=CARTESIAN_POINT('Ctrl Pts',(84.0294223509248,52.6181314106496,30.012074375147)) ;
#16133=CARTESIAN_POINT('Ctrl Pts',(84.0100971870989,52.3376484412462,30.0363197478244)) ;
#16134=CARTESIAN_POINT('Ctrl Pts',(84.0104076499753,52.3005538149027,30.0395225593024)) ;
#16135=CARTESIAN_POINT('Origin',(84.75,52.3,25.7604774406976)) ;
#16136=CARTESIAN_POINT('',(84.0103561101056,52.3005355198033,29.1604774406976)) ;
#16137=CARTESIAN_POINT('',(84.0121527080028,52.3000803219525,29.2395225593024)) ;
#16138=CARTESIAN_POINT('',(84.011,52.2999999999999,25.7604774406976)) ;
#16139=CARTESIAN_POINT('Ctrl Pts',(84.0103561101056,52.3005355198033,29.1604774406976)) ;
#16140=CARTESIAN_POINT('Ctrl Pts',(84.012061911087,52.0920492800597,29.1784817587012)) ;
#16141=CARTESIAN_POINT('Ctrl Pts',(84.2125467370667,51.6370213192352,29.217528637904)) ;
#16142=CARTESIAN_POINT('Ctrl Pts',(84.9818830553883,51.4596763776764,29.2776180783061)) ;
#16143=CARTESIAN_POINT('Ctrl Pts',(85.5801926949256,52.0341172609902,29.340745761904)) ;
#16144=CARTESIAN_POINT('Ctrl Pts',(85.4269212141838,52.8492642455131,29.4038734455019)) ;
#16145=CARTESIAN_POINT('Ctrl Pts',(84.6608267013838,53.1671572316628,29.4670011290997)) ;
#16146=CARTESIAN_POINT('Ctrl Pts',(84.0940868976613,52.780861082125,29.5192024608316)) ;
#16147=CARTESIAN_POINT('Ctrl Pts',(84.0120451724208,52.4179475537566,29.5503612313643)) ;
#16148=CARTESIAN_POINT('Ctrl Pts',(84.0121537087894,52.3000753650543,29.5604774406976)) ;
#16149=CARTESIAN_POINT('Ctrl Pts',(84.0121527080028,52.3000803219525,29.2395225593024)) ;
#16150=CARTESIAN_POINT('Ctrl Pts',(84.0122779623987,52.172457021707,29.2504756800996)) ;
#16151=CARTESIAN_POINT('Ctrl Pts',(84.1042331481866,51.7994814638448,29.282471362096)) ;
#16152=CARTESIAN_POINT('Ctrl Pts',(84.6950865774281,51.4300011013776,29.3355096052917)) ;
#16153=CARTESIAN_POINT('Ctrl Pts',(85.4480514094807,51.7778527053553,29.3986372888896)) ;
#16154=CARTESIAN_POINT('Ctrl Pts',(85.5690638483639,52.5984090814401,29.4617649724875)) ;
#16155=CARTESIAN_POINT('Ctrl Pts',(84.9485702146255,53.148812957869,29.5248926560853)) ;
#16156=CARTESIAN_POINT('Ctrl Pts',(84.1974339403033,52.9441628692833,29.5841451850237)) ;
#16157=CARTESIAN_POINT('Ctrl Pts',(84.0123986086908,52.4983721994821,29.6223551527627)) ;
#16158=CARTESIAN_POINT('Ctrl Pts',(84.0106286778565,52.2993868276063,29.6395225593024)) ;
#16159=CARTESIAN_POINT('Origin',(84.75,52.3,25.7604774406976)) ;
#16160=CARTESIAN_POINT('',(84.0106846088523,52.2993761801769,28.7604774406976)) ;
#16161=CARTESIAN_POINT('',(84.0103478306111,52.3005324085697,28.8395225593024)) ;
#16162=CARTESIAN_POINT('',(84.011,52.2999999999999,25.7604774406976)) ;
#16163=CARTESIAN_POINT('Ctrl Pts',(84.0106846088524,52.2993761801769,28.7604774406976)) ;
#16164=CARTESIAN_POINT('Ctrl Pts',(84.0102646767194,52.2525430796879,28.7645171636395)) ;
#16165=CARTESIAN_POINT('Ctrl Pts',(84.0355591348416,51.962212287757,28.7895994477806)) ;
#16166=CARTESIAN_POINT('Ctrl Pts',(84.4195286707959,51.4933388306201,28.835724293121)) ;
#16167=CARTESIAN_POINT('Ctrl Pts',(85.2442182847965,51.5819040255063,28.8988519767189)) ;
#16168=CARTESIAN_POINT('Ctrl Pts',(85.6214875174565,52.3205681435423,28.9619796603168)) ;
#16169=CARTESIAN_POINT('Ctrl Pts',(85.2097910453075,53.0406117311157,29.0251073439146)) ;
#16170=CARTESIAN_POINT('Ctrl Pts',(84.3818414899421,53.090172672954,29.0882350275125)) ;
#16171=CARTESIAN_POINT('Ctrl Pts',(84.0282664307177,52.6142693996754,29.1333583931068)) ;
#16172=CARTESIAN_POINT('Ctrl Pts',(84.0100682548131,52.3357177410451,29.1574391975019)) ;
#16173=CARTESIAN_POINT('Ctrl Pts',(84.0103561101056,52.3005355198033,29.1604774406976)) ;
#16174=CARTESIAN_POINT('Ctrl Pts',(84.0103478306111,52.3005324085697,28.8395225593024)) ;
#16175=CARTESIAN_POINT('Ctrl Pts',(84.0120492717183,52.091742275103,28.8575536462372)) ;
#16176=CARTESIAN_POINT('Ctrl Pts',(84.2130406468208,51.6364224339068,28.8966272943712)) ;
#16177=CARTESIAN_POINT('Ctrl Pts',(84.9829429060078,51.4599695421454,28.9567435037046)) ;
#16178=CARTESIAN_POINT('Ctrl Pts',(85.5805274479185,52.0351647194261,29.0198711873024)) ;
#16179=CARTESIAN_POINT('Ctrl Pts',(85.4262278145717,52.8501177241122,29.0829988709003)) ;
#16180=CARTESIAN_POINT('Ctrl Pts',(84.6597328902445,53.1670440683605,29.1461265544982)) ;
#16181=CARTESIAN_POINT('Ctrl Pts',(84.0937711983123,52.7802317621059,29.1983011172988)) ;
#16182=CARTESIAN_POINT('Ctrl Pts',(84.0120373302227,52.4176402124707,29.2294331189003)) ;
#16183=CARTESIAN_POINT('Ctrl Pts',(84.0121527080028,52.3000803219525,29.2395225593024)) ;
#16184=CARTESIAN_POINT('Origin',(84.75,52.3,25.7604774406976)) ;
#16185=CARTESIAN_POINT('',(84.012145263812,52.3001106858399,28.3604774406976)) ;
#16186=CARTESIAN_POINT('',(84.0106937367584,52.299374595264,28.4395225593024)) ;
#16187=CARTESIAN_POINT('',(84.011,52.2999999999999,25.7604774406976)) ;
#16188=CARTESIAN_POINT('Ctrl Pts',(84.012145263812,52.3001106858399,28.3604774406976)) ;
#16189=CARTESIAN_POINT('Ctrl Pts',(84.012320562902,52.1705731480788,28.3715951297771)) ;
#16190=CARTESIAN_POINT('Ctrl Pts',(84.1062919598857,51.7956207689212,28.4037553800558)) ;
#16191=CARTESIAN_POINT('Ctrl Pts',(84.7018350882737,51.4296014229731,28.4569581915339)) ;
#16192=CARTESIAN_POINT('Ctrl Pts',(85.4520796692884,51.7832818180256,28.5200858751317)) ;
#16193=CARTESIAN_POINT('Ctrl Pts',(85.566725036296,52.6047519593021,28.5832135587296)) ;
#16194=CARTESIAN_POINT('Ctrl Pts',(84.9419816788649,53.1503273349667,28.6463412423274)) ;
#16195=CARTESIAN_POINT('Ctrl Pts',(84.1945368090908,52.9404428849206,28.7054292029835)) ;
#16196=CARTESIAN_POINT('Ctrl Pts',(84.0124520662344,52.4964925775559,28.7434746024402)) ;
#16197=CARTESIAN_POINT('Ctrl Pts',(84.0106846088524,52.2993761801769,28.7604774406976)) ;
#16198=CARTESIAN_POINT('Ctrl Pts',(84.0106937367584,52.299374595264,28.4395225593024)) ;
#16199=CARTESIAN_POINT('Ctrl Pts',(84.0102705539735,52.2522296530489,28.4435890511755)) ;
#16200=CARTESIAN_POINT('Ctrl Pts',(84.0357626124065,51.9615831483613,28.4686981042478)) ;
#16201=CARTESIAN_POINT('Ctrl Pts',(84.4205464955366,51.4929225836516,28.5148497185195)) ;
#16202=CARTESIAN_POINT('Ctrl Pts',(85.2451237463938,51.5825280191257,28.5779774021174)) ;
#16203=CARTESIAN_POINT('Ctrl Pts',(85.6214608931572,52.3216674705582,28.6411050857152)) ;
#16204=CARTESIAN_POINT('Ctrl Pts',(85.2088564383358,53.0411911606195,28.7042327693131)) ;
#16205=CARTESIAN_POINT('Ctrl Pts',(84.3808450086281,53.08970764206,28.767360452911)) ;
#16206=CARTESIAN_POINT('Ctrl Pts',(84.0280799537887,52.6136413086296,28.8124570495741)) ;
#16207=CARTESIAN_POINT('Ctrl Pts',(84.0100636632658,52.3354036349076,28.8365110850379)) ;
#16208=CARTESIAN_POINT('Ctrl Pts',(84.0103478306111,52.3005324085697,28.8395225593024)) ;
#16209=CARTESIAN_POINT('Origin',(84.75,52.3,25.7604774406976)) ;
#16210=CARTESIAN_POINT('',(84.0102978130501,52.3005124640715,27.9604774406976)) ;
#16211=CARTESIAN_POINT('',(84.0121438140165,52.3001156043131,28.0395225593024)) ;
#16212=CARTESIAN_POINT('',(84.011,52.2999999999999,25.7604774406976)) ;
#16213=CARTESIAN_POINT('Ctrl Pts',(84.0102978130501,52.3005124640715,27.9604774406976)) ;
#16214=CARTESIAN_POINT('Ctrl Pts',(84.0119690402742,52.0898539400114,27.9786730959147)) ;
#16215=CARTESIAN_POINT('Ctrl Pts',(84.2160915677973,51.6327449502991,28.017911312331)) ;
#16216=CARTESIAN_POINT('Ctrl Pts',(84.989450350052,51.4618012935295,28.0781920899466)) ;
#16217=CARTESIAN_POINT('Ctrl Pts',(85.5825562620867,52.0416134444791,28.1413197735445)) ;
#16218=CARTESIAN_POINT('Ctrl Pts',(85.4219412946177,52.8553453323684,28.2044474571424)) ;
#16219=CARTESIAN_POINT('Ctrl Pts',(84.6530116623168,53.1663179577801,28.2675751407402)) ;
#16220=CARTESIAN_POINT('Ctrl Pts',(84.0918423690182,52.7763621308894,28.3195851352587)) ;
#16221=CARTESIAN_POINT('Ctrl Pts',(84.011988772563,52.4157501400294,28.3505525685778)) ;
#16222=CARTESIAN_POINT('Ctrl Pts',(84.012145263812,52.3001106858399,28.3604774406976)) ;
#16223=CARTESIAN_POINT('Ctrl Pts',(84.0121438140165,52.3001156043131,28.0395225593024)) ;
#16224=CARTESIAN_POINT('Ctrl Pts',(84.0123273641732,52.1702667990095,28.0506670173131)) ;
#16225=CARTESIAN_POINT('Ctrl Pts',(84.1066288342844,51.794992936399,28.0828540365231)) ;
#16226=CARTESIAN_POINT('Ctrl Pts',(84.7029330951489,51.4295413427059,28.1360836169323)) ;
#16227=CARTESIAN_POINT('Ctrl Pts',(85.4527309398621,51.7841678628247,28.1992113005302)) ;
#16228=CARTESIAN_POINT('Ctrl Pts',(85.5663399692938,52.6057819846142,28.2623389841281)) ;
#16229=CARTESIAN_POINT('Ctrl Pts',(84.9409088790051,53.1505688493595,28.3254666677259)) ;
#16230=CARTESIAN_POINT('Ctrl Pts',(84.1940678498118,52.9398372061532,28.3845278594507)) ;
#16231=CARTESIAN_POINT('Ctrl Pts',(84.0124603652231,52.4961869417292,28.4225464899762)) ;
#16232=CARTESIAN_POINT('Ctrl Pts',(84.0106937367584,52.299374595264,28.4395225593024)) ;
#16233=CARTESIAN_POINT('Origin',(84.75,52.3,25.7604774406976)) ;
#16234=CARTESIAN_POINT('',(84.0107501619265,52.299365759712,27.5604774406976)) ;
#16235=CARTESIAN_POINT('',(84.0102897973284,52.3005090881678,27.6395225593024)) ;
#16236=CARTESIAN_POINT('',(84.011,52.2999999999999,25.7604774406976)) ;
#16237=CARTESIAN_POINT('Ctrl Pts',(84.0107501619265,52.299365759712,27.5604774406976)) ;
#16238=CARTESIAN_POINT('Ctrl Pts',(84.0103074630672,52.2503032365772,27.564708500853)) ;
#16239=CARTESIAN_POINT('Ctrl Pts',(84.0370235408122,51.9577148666482,27.5899821222076)) ;
#16240=CARTESIAN_POINT('Ctrl Pts',(84.4268153114771,51.490391953806,27.6362983047616)) ;
#16241=CARTESIAN_POINT('Ctrl Pts',(85.2506728575663,51.5863892979384,27.6994259883594)) ;
#16242=CARTESIAN_POINT('Ctrl Pts',(85.6212666417578,52.3284250163863,27.7625536719573)) ;
#16243=CARTESIAN_POINT('Ctrl Pts',(85.203094680064,53.0447272999564,27.8256813555552)) ;
#16244=CARTESIAN_POINT('Ctrl Pts',(84.3747319174341,53.0868210776482,27.8888090391531)) ;
#16245=CARTESIAN_POINT('Ctrl Pts',(84.0269431929634,52.6097805786841,27.9337410675339)) ;
#16246=CARTESIAN_POINT('Ctrl Pts',(84.0100363315741,52.3334722561318,27.9576305347154)) ;
#16247=CARTESIAN_POINT('Ctrl Pts',(84.0102978130501,52.3005124640715,27.9604774406976)) ;
#16248=CARTESIAN_POINT('Ctrl Pts',(84.0102897973284,52.3005090881678,27.6395225593024)) ;
#16249=CARTESIAN_POINT('Ctrl Pts',(84.0119555459036,52.0895466130168,27.6577449834507)) ;
#16250=CARTESIAN_POINT('Ctrl Pts',(84.2165901750469,51.6321474461671,27.6970099687983)) ;
#16251=CARTESIAN_POINT('Ctrl Pts',(84.9905075141293,51.4621040018937,27.7573175153451)) ;
#16252=CARTESIAN_POINT('Ctrl Pts',(85.5828815572153,52.042663878742,27.820445198943)) ;
#16253=CARTESIAN_POINT('Ctrl Pts',(85.4212402278205,52.8561925242217,27.8835728825408)) ;
#16254=CARTESIAN_POINT('Ctrl Pts',(84.6519189159883,53.1661949368354,27.9467005661387)) ;
#16255=CARTESIAN_POINT('Ctrl Pts',(84.0915305454382,52.7757325930713,27.9986837917259)) ;
#16256=CARTESIAN_POINT('Ctrl Pts',(84.011980791428,52.4154426011558,28.0296244561138)) ;
#16257=CARTESIAN_POINT('Ctrl Pts',(84.0121438140165,52.3001156043131,28.0395225593024)) ;
#16258=CARTESIAN_POINT('Origin',(84.75,52.3,25.7604774406976)) ;
#16259=CARTESIAN_POINT('',(84.0121337603747,52.3001460493381,27.1604774406976)) ;
#16260=CARTESIAN_POINT('',(84.0107593547378,52.2993644693424,27.2395225593024)) ;
#16261=CARTESIAN_POINT('',(84.011,52.2999999999999,25.7604774406976)) ;
#16262=CARTESIAN_POINT('Ctrl Pts',(84.0121337603747,52.3001460493381,27.1604774406976)) ;
#16263=CARTESIAN_POINT('Ctrl Pts',(84.0123686127965,52.1683841800178,27.1717864669906)) ;
#16264=CARTESIAN_POINT('Ctrl Pts',(84.1087120145737,51.7911337021563,27.2041380544828)) ;
#16265=CARTESIAN_POINT('Ctrl Pts',(84.7096850855178,51.4292029103844,27.2575322031744)) ;
#16266=CARTESIAN_POINT('Ctrl Pts',(85.4567100107038,51.7896328869262,27.3206598867723)) ;
#16267=CARTESIAN_POINT('Ctrl Pts',(85.5639440986358,52.6121036097496,27.3837875703701)) ;
#16268=CARTESIAN_POINT('Ctrl Pts',(84.934306938815,53.1520237140672,27.446915253968)) ;
#16269=CARTESIAN_POINT('Ctrl Pts',(84.1911990172918,52.9361100119052,27.5058118774105)) ;
#16270=CARTESIAN_POINT('Ctrl Pts',(84.012509161341,52.4943085467702,27.5436659396537)) ;
#16271=CARTESIAN_POINT('Ctrl Pts',(84.0107501619265,52.299365759712,27.5604774406976)) ;
#16272=CARTESIAN_POINT('Ctrl Pts',(84.0107593547378,52.2993644693424,27.2395225593024)) ;
#16273=CARTESIAN_POINT('Ctrl Pts',(84.010313557306,52.2499899466507,27.243780388389)) ;
#16274=CARTESIAN_POINT('Ctrl Pts',(84.0372302203536,51.95708550979,27.2690807786749)) ;
#16275=CARTESIAN_POINT('Ctrl Pts',(84.4278368710099,51.4899849375734,27.31542373016)) ;
#16276=CARTESIAN_POINT('Ctrl Pts',(85.2515726447776,51.5870214121571,27.3785514137579)) ;
#16277=CARTESIAN_POINT('Ctrl Pts',(85.6212301121436,52.3295240675631,27.4416790973558)) ;
#16278=CARTESIAN_POINT('Ctrl Pts',(85.2021548839321,53.0452982747,27.5048067809536)) ;
#16279=CARTESIAN_POINT('Ctrl Pts',(84.3737396709075,53.0863470831135,27.5679344645515)) ;
#16280=CARTESIAN_POINT('Ctrl Pts',(84.0267598229767,52.6091526983306,27.6128397240011)) ;
#16281=CARTESIAN_POINT('Ctrl Pts',(84.0100320029078,52.3331580424289,27.6367024222514)) ;
#16282=CARTESIAN_POINT('Ctrl Pts',(84.0102897973284,52.3005090881678,27.6395225593024)) ;
#16283=CARTESIAN_POINT('Origin',(84.75,52.3,25.7604774406976)) ;
#16284=CARTESIAN_POINT('',(84.010254873815,52.3005215753354,26.7604774406976)) ;
#16285=CARTESIAN_POINT('',(84.0121333942101,52.3001533432303,26.8395225593024)) ;
#16286=CARTESIAN_POINT('',(84.011,52.2999999999999,25.7604774406976)) ;
#16287=CARTESIAN_POINT('Ctrl Pts',(84.010254873815,52.3005215753354,26.7604774406976)) ;
#16288=CARTESIAN_POINT('Ctrl Pts',(84.0118865417744,52.0876983314931,26.7788644331282)) ;
#16289=CARTESIAN_POINT('Ctrl Pts',(84.2196500716081,51.6284277708823,26.818293986758)) ;
#16290=CARTESIAN_POINT('Ctrl Pts',(84.9970086663633,51.464021058011,26.8787661015872)) ;
#16291=CARTESIAN_POINT('Ctrl Pts',(85.584846975971,52.0491174747966,26.941893785185)) ;
#16292=CARTESIAN_POINT('Ctrl Pts',(85.4169092945958,52.8613877554865,27.0050214687829)) ;
#16293=CARTESIAN_POINT('Ctrl Pts',(84.6452032531813,53.1654050588536,27.0681491523808)) ;
#16294=CARTESIAN_POINT('Ctrl Pts',(84.0896257601006,52.7718624007159,27.1199678096857)) ;
#16295=CARTESIAN_POINT('Ctrl Pts',(84.0119316258861,52.4135518122329,27.1507439057913)) ;
#16296=CARTESIAN_POINT('Ctrl Pts',(84.0121337603747,52.3001460493381,27.1604774406976)) ;
#16297=CARTESIAN_POINT('Ctrl Pts',(84.0121333942101,52.3001533432303,26.8395225593024)) ;
#16298=CARTESIAN_POINT('Ctrl Pts',(84.0123759877409,52.1680792935557,26.8508583545266)) ;
#16299=CARTESIAN_POINT('Ctrl Pts',(84.1090503779434,51.7905022090762,26.8832367109501)) ;
#16300=CARTESIAN_POINT('Ctrl Pts',(84.710785203412,51.4291552942847,26.9366576285728)) ;
#16301=CARTESIAN_POINT('Ctrl Pts',(85.4573524705639,51.7905235055957,26.9997853121707)) ;
#16302=CARTESIAN_POINT('Ctrl Pts',(85.5635501520105,52.6131307432408,27.0629129957686)) ;
#16303=CARTESIAN_POINT('Ctrl Pts',(84.933231811866,53.1522552393336,27.1260406793665)) ;
#16304=CARTESIAN_POINT('Ctrl Pts',(84.1907347271212,52.9355032943271,27.1849105338777)) ;
#16305=CARTESIAN_POINT('Ctrl Pts',(84.0125167269381,52.4940031266761,27.2227378271897)) ;
#16306=CARTESIAN_POINT('Ctrl Pts',(84.0107593547378,52.2993644693424,27.2395225593024)) ;
#16307=CARTESIAN_POINT('Origin',(84.75,52.3,32.05)) ;
#16308=CARTESIAN_POINT('',(85.6645587247976,52.6133494876276,32.05)) ;
#16309=CARTESIAN_POINT('Ctrl Pts',(84.6290682970003,51.5698134220425,32.05)) ;
#16310=CARTESIAN_POINT('Ctrl Pts',(84.6486054756756,51.5633636415286,32.05)) ;
#16311=CARTESIAN_POINT('Ctrl Pts',(84.6683837217373,51.5577953863303,32.05)) ;
#16312=CARTESIAN_POINT('Ctrl Pts',(84.6883526700962,51.5531398112781,32.05)) ;
#16313=CARTESIAN_POINT('Ctrl Pts',(84.7208023354277,51.5455744728509,32.05)) ;
#16314=CARTESIAN_POINT('Ctrl Pts',(84.7537544638827,51.5404164732051,32.05)) ;
#16315=CARTESIAN_POINT('Ctrl Pts',(84.7869911094308,51.5375362654893,32.05)) ;
#16316=CARTESIAN_POINT('Ctrl Pts',(84.797421598867,51.5366323843767,32.05)) ;
#16317=CARTESIAN_POINT('Ctrl Pts',(84.8078802856998,51.5359531478234,32.05)) ;
#16318=CARTESIAN_POINT('Ctrl Pts',(84.818360849627,51.5354954119729,32.05)) ;
#16319=CARTESIAN_POINT('Ctrl Pts',(84.8273128543076,51.5351044355423,32.05)) ;
#16320=CARTESIAN_POINT('Ctrl Pts',(84.8362803076888,51.5348752539893,32.05)) ;
#16321=CARTESIAN_POINT('Ctrl Pts',(84.8452455423231,51.5348057051637,32.05)) ;
#16322=CARTESIAN_POINT('Ctrl Pts',(84.8809024636672,51.5345290925477,32.05)) ;
#16323=CARTESIAN_POINT('Ctrl Pts',(84.9165773339652,51.5367708227219,32.05)) ;
#16324=CARTESIAN_POINT('Ctrl Pts',(84.9520181276991,51.5413821237009,32.05)) ;
#16325=CARTESIAN_POINT('Ctrl Pts',(84.9775637855138,51.5447059408189,32.05)) ;
#16326=CARTESIAN_POINT('Ctrl Pts',(85.0029885312786,51.5492619056144,32.05)) ;
#16327=CARTESIAN_POINT('Ctrl Pts',(85.0282030317967,51.5550099525335,32.05)) ;
#16328=CARTESIAN_POINT('Ctrl Pts',(85.0362872843134,51.5568528866316,32.05)) ;
#16329=CARTESIAN_POINT('Ctrl Pts',(85.0443485937157,51.5588182817752,32.05)) ;
#16330=CARTESIAN_POINT('Ctrl Pts',(85.052372137682,51.5609014997111,32.05)) ;
#16331=CARTESIAN_POINT('Ctrl Pts',(85.0889237057945,51.5703916804338,32.05)) ;
#16332=CARTESIAN_POINT('Ctrl Pts',(85.1247567909586,51.5823375166551,32.05)) ;
#16333=CARTESIAN_POINT('Ctrl Pts',(85.1596013391966,51.5965816118641,32.05)) ;
#16334=CARTESIAN_POINT('Ctrl Pts',(85.1947214437706,51.6109383516871,32.05)) ;
#16335=CARTESIAN_POINT('Ctrl Pts',(85.2288386803151,51.627629956059,32.05)) ;
#16336=CARTESIAN_POINT('Ctrl Pts',(85.2616821666479,51.646548385543,32.05)) ;
#16337=CARTESIAN_POINT('Ctrl Pts',(85.2787824571817,51.6563984555794,32.05)) ;
#16338=CARTESIAN_POINT('Ctrl Pts',(85.2955374178107,51.6668530503173,32.05)) ;
#16339=CARTESIAN_POINT('Ctrl Pts',(85.3119074772461,51.677902377199,32.05)) ;
#16340=CARTESIAN_POINT('Ctrl Pts',(85.3200219818723,51.6833794381989,32.05)) ;
#16341=CARTESIAN_POINT('Ctrl Pts',(85.3280442877998,51.6890046707409,32.05)) ;
#16342=CARTESIAN_POINT('Ctrl Pts',(85.3359493062664,51.694761862387,32.05)) ;
#16343=CARTESIAN_POINT('Ctrl Pts',(85.3685071062967,51.7184735709857,32.05)) ;
#16344=CARTESIAN_POINT('Ctrl Pts',(85.3991472042605,51.7444650511667,32.05)) ;
#16345=CARTESIAN_POINT('Ctrl Pts',(85.4275676556062,51.7725897979014,32.05)) ;
#16346=CARTESIAN_POINT('Ctrl Pts',(85.4543169662164,51.799060791521,32.05)) ;
#16347=CARTESIAN_POINT('Ctrl Pts',(85.4791015982827,51.8274219759074,32.05)) ;
#16348=CARTESIAN_POINT('Ctrl Pts',(85.5019075504341,51.8574120322123,32.05)) ;
#16349=CARTESIAN_POINT('Ctrl Pts',(85.5123316294908,51.8711198009458,32.05)) ;
#16350=CARTESIAN_POINT('Ctrl Pts',(85.5223419418911,51.8851684883569,32.05)) ;
#16351=CARTESIAN_POINT('Ctrl Pts',(85.5319350286684,51.8995359094532,32.05)) ;
#16352=CARTESIAN_POINT('Ctrl Pts',(85.5372176410402,51.9074475981717,32.05)) ;
#16353=CARTESIAN_POINT('Ctrl Pts',(85.542373710439,51.9154559659869,32.05)) ;
#16354=CARTESIAN_POINT('Ctrl Pts',(85.5474024643045,51.9235574931787,32.05)) ;
#16355=CARTESIAN_POINT('Ctrl Pts',(85.5517120936517,51.9305004814967,32.05)) ;
#16356=CARTESIAN_POINT('Ctrl Pts',(85.5559234083183,51.9375042085288,32.05)) ;
#16357=CARTESIAN_POINT('Ctrl Pts',(85.5600348116964,51.9445630629369,32.05)) ;
#16358=CARTESIAN_POINT('Ctrl Pts',(85.5799659198025,51.9787827143242,32.05)) ;
#16359=CARTESIAN_POINT('Ctrl Pts',(85.5975643889103,52.0143151477684,32.05)) ;
#16360=CARTESIAN_POINT('Ctrl Pts',(85.6128251657119,52.050862155833,32.05)) ;
#16361=CARTESIAN_POINT('Ctrl Pts',(85.6284402685273,52.0882577154394,32.05)) ;
#16362=CARTESIAN_POINT('Ctrl Pts',(85.6416085142695,52.1267164034934,32.05)) ;
#16363=CARTESIAN_POINT('Ctrl Pts',(85.6522878131956,52.165959075351,32.05)) ;
#16364=CARTESIAN_POINT('Ctrl Pts',(85.6574156485319,52.184802068775,32.05)) ;
#16365=CARTESIAN_POINT('Ctrl Pts',(85.6619690371714,52.2038263204532,32.05)) ;
#16366=CARTESIAN_POINT('Ctrl Pts',(85.6659397311219,52.2230031348788,32.05)) ;
#16367=CARTESIAN_POINT('Ctrl Pts',(85.6677315738388,52.2316569963174,32.05)) ;
#16368=CARTESIAN_POINT('Ctrl Pts',(85.6694047219091,52.2403419407282,32.05)) ;
#16369=CARTESIAN_POINT('Ctrl Pts',(85.6709582458612,52.2490553928039,32.05)) ;
#16370=CARTESIAN_POINT('Ctrl Pts',(85.6723899282023,52.2570854559705,32.05)) ;
#16371=CARTESIAN_POINT('Ctrl Pts',(85.6737182376174,52.2651298209158,32.05)) ;
#16372=CARTESIAN_POINT('Ctrl Pts',(85.6749429936691,52.2731853280596,32.05)) ;
#16373=CARTESIAN_POINT('Ctrl Pts',(85.6813033393252,52.3150188097536,32.05)) ;
#16374=CARTESIAN_POINT('Ctrl Pts',(85.6848756544714,52.3571575210195,32.05)) ;
#16375=CARTESIAN_POINT('Ctrl Pts',(85.6856310209224,52.3992957021883,32.05)) ;
#16376=CARTESIAN_POINT('Ctrl Pts',(85.6863812796774,52.441148950098,32.05)) ;
#16377=CARTESIAN_POINT('Ctrl Pts',(85.6843530088631,52.4830028899044,32.05)) ;
#16378=CARTESIAN_POINT('Ctrl Pts',(85.6794724997026,52.5245795220203,32.05)) ;
#16379=CARTESIAN_POINT('Ctrl Pts',(85.6759784989651,52.5543446097399,32.05)) ;
#16380=CARTESIAN_POINT('Ctrl Pts',(85.6710217340403,52.5839680712491,32.05)) ;
#16381=CARTESIAN_POINT('Ctrl Pts',(85.6645587247976,52.6133494876276,32.05)) ;
#16382=CARTESIAN_POINT('',(83.78325,52.3,32.05)) ;
#16383=CARTESIAN_POINT('Origin',(84.75,52.3,32.05)) ;
#16384=CARTESIAN_POINT('',(85.0634162962529,53.2161025497301,32.05)) ;
#16385=CARTESIAN_POINT('Origin',(84.75,52.3,32.05)) ;
#16386=CARTESIAN_POINT('Ctrl Pts',(85.0634162962528,53.2161025497302,32.05)) ;
#16387=CARTESIAN_POINT('Ctrl Pts',(85.0375903626687,53.2219158833822,32.05)) ;
#16388=CARTESIAN_POINT('Ctrl Pts',(85.0115585907843,53.2265873685398,32.05)) ;
#16389=CARTESIAN_POINT('Ctrl Pts',(84.9853698812676,53.2300642668749,32.05)) ;
#16390=CARTESIAN_POINT('Ctrl Pts',(84.9482204181441,53.2349963505426,32.05)) ;
#16391=CARTESIAN_POINT('Ctrl Pts',(84.9107544993145,53.2375257569857,32.05)) ;
#16392=CARTESIAN_POINT('Ctrl Pts',(84.8731799721622,53.2377230918043,32.05)) ;
#16393=CARTESIAN_POINT('Ctrl Pts',(84.8583111944688,53.2378011800139,32.05)) ;
#16394=CARTESIAN_POINT('Ctrl Pts',(84.8434255126426,53.2375137512002,32.05)) ;
#16395=CARTESIAN_POINT('Ctrl Pts',(84.8285363533114,53.2368639235865,32.05)) ;
#16396=CARTESIAN_POINT('Ctrl Pts',(84.8151276070541,53.2362787076325,32.05)) ;
#16397=CARTESIAN_POINT('Ctrl Pts',(84.8017114154886,53.2353989415351,32.05)) ;
#16398=CARTESIAN_POINT('Ctrl Pts',(84.7883268826021,53.234229649649,32.05)) ;
#16399=CARTESIAN_POINT('Ctrl Pts',(84.7467495586251,53.2305973953159,32.05)) ;
#16400=CARTESIAN_POINT('Ctrl Pts',(84.7054263758008,53.2241747289076,32.05)) ;
#16401=CARTESIAN_POINT('Ctrl Pts',(84.6646494982219,53.2150591487198,32.05)) ;
#16402=CARTESIAN_POINT('Ctrl Pts',(84.6409788399251,53.2097676257633,32.05)) ;
#16403=CARTESIAN_POINT('Ctrl Pts',(84.6174926209232,53.2035677546806,32.05)) ;
#16404=CARTESIAN_POINT('Ctrl Pts',(84.5942525737568,53.1964719333739,32.05)) ;
#16405=CARTESIAN_POINT('Ctrl Pts',(84.585513077665,53.1938035264583,32.05)) ;
#16406=CARTESIAN_POINT('Ctrl Pts',(84.5768084370589,53.1910083729646,32.05)) ;
#16407=CARTESIAN_POINT('Ctrl Pts',(84.568142102793,53.188086977312,32.05)) ;
#16408=CARTESIAN_POINT('Ctrl Pts',(84.5599799601992,53.1853355431811,32.05)) ;
#16409=CARTESIAN_POINT('Ctrl Pts',(84.5518564838162,53.1824736325861,32.05)) ;
#16410=CARTESIAN_POINT('Ctrl Pts',(84.5437817785724,53.1795048835846,32.05)) ;
#16411=CARTESIAN_POINT('Ctrl Pts',(84.5061169942788,53.1656570355968,32.05)) ;
#16412=CARTESIAN_POINT('Ctrl Pts',(84.469460386035,53.1494709330162,32.05)) ;
#16413=CARTESIAN_POINT('Ctrl Pts',(84.4340761666869,53.1310298954467,32.05)) ;
#16414=CARTESIAN_POINT('Ctrl Pts',(84.3995110501093,53.1130157460563,32.05)) ;
#16415=CARTESIAN_POINT('Ctrl Pts',(84.3661592694239,53.0928491386052,32.05)) ;
#16416=CARTESIAN_POINT('Ctrl Pts',(84.3343026524149,53.070575118304,32.05)) ;
#16417=CARTESIAN_POINT('Ctrl Pts',(84.3189936953075,53.0598711561945,32.05)) ;
#16418=CARTESIAN_POINT('Ctrl Pts',(84.3040306344131,53.0486800927604,32.05)) ;
#16419=CARTESIAN_POINT('Ctrl Pts',(84.2894485931079,53.0370048640332,32.05)) ;
#16420=CARTESIAN_POINT('Ctrl Pts',(84.2821858372867,53.0311898801343,32.05)) ;
#16421=CARTESIAN_POINT('Ctrl Pts',(84.2750176419556,53.0252547731509,32.05)) ;
#16422=CARTESIAN_POINT('Ctrl Pts',(84.2679486148627,53.019199805017,32.05)) ;
#16423=CARTESIAN_POINT('Ctrl Pts',(84.2621177465606,53.0142053805654,32.05)) ;
#16424=CARTESIAN_POINT('Ctrl Pts',(84.2563618671862,53.0091358377593,32.05)) ;
#16425=CARTESIAN_POINT('Ctrl Pts',(84.2506831552877,53.0039919568579,32.05)) ;
#16426=CARTESIAN_POINT('Ctrl Pts',(84.2235295101632,52.97939568942,32.05)) ;
#16427=CARTESIAN_POINT('Ctrl Pts',(84.1981352605778,52.9531001772539,32.05)) ;
#16428=CARTESIAN_POINT('Ctrl Pts',(84.1747348706618,52.9251520670723,32.05)) ;
#16429=CARTESIAN_POINT('Ctrl Pts',(84.152837480384,52.8989990551623,32.05)) ;
#16430=CARTESIAN_POINT('Ctrl Pts',(84.1326864154153,52.8713977926676,32.05)) ;
#16431=CARTESIAN_POINT('Ctrl Pts',(84.1143384424733,52.8425442600233,32.05)) ;
#16432=CARTESIAN_POINT('Ctrl Pts',(84.1045838240468,52.8272044073818,32.05)) ;
#16433=CARTESIAN_POINT('Ctrl Pts',(84.0953393822899,52.8115104725868,32.05)) ;
#16434=CARTESIAN_POINT('Ctrl Pts',(84.0866173651522,52.7954916943026,32.05)) ;
#16435=CARTESIAN_POINT('Ctrl Pts',(84.0822883255137,52.7875410190106,32.05)) ;
#16436=CARTESIAN_POINT('Ctrl Pts',(84.0780880245306,52.7795103220941,32.05)) ;
#16437=CARTESIAN_POINT('Ctrl Pts',(84.0740181996644,52.7714032163815,32.05)) ;
#16438=CARTESIAN_POINT('Ctrl Pts',(84.0705530522315,52.764500630282,32.05)) ;
#16439=CARTESIAN_POINT('Ctrl Pts',(84.0671826623095,52.7575426978405,32.05)) ;
#16440=CARTESIAN_POINT('Ctrl Pts',(84.0639137672541,52.7505445638357,32.05)) ;
#16441=CARTESIAN_POINT('Ctrl Pts',(84.0481282892796,52.7167506095102,32.05)) ;
#16442=CARTESIAN_POINT('Ctrl Pts',(84.0346671737874,52.68194532237,32.05)) ;
#16443=CARTESIAN_POINT('Ctrl Pts',(84.0235884717775,52.6463938282192,32.05)) ;
#16444=CARTESIAN_POINT('Ctrl Pts',(84.012629449038,52.6112263841922,32.05)) ;
#16445=CARTESIAN_POINT('Ctrl Pts',(84.0040017040798,52.5753274496591,32.05)) ;
#16446=CARTESIAN_POINT('Ctrl Pts',(83.9978116824037,52.5389572210107,32.05)) ;
#16447=CARTESIAN_POINT('Ctrl Pts',(83.9950331653952,52.5226317048508,32.05)) ;
#16448=CARTESIAN_POINT('Ctrl Pts',(83.9927464851397,52.506211397335,32.05)) ;
#16449=CARTESIAN_POINT('Ctrl Pts',(83.9909645624641,52.4897211182932,32.05)) ;
#16450=CARTESIAN_POINT('Ctrl Pts',(83.9901106015459,52.4818183882679,32.05)) ;
#16451=CARTESIAN_POINT('Ctrl Pts',(83.9893724702862,52.4738979582126,32.05)) ;
#16452=CARTESIAN_POINT('Ctrl Pts',(83.9887521538462,52.4659678151963,32.05)) ;
#16453=CARTESIAN_POINT('Ctrl Pts',(83.9859881691425,52.4306329561157,32.05)) ;
#16454=CARTESIAN_POINT('Ctrl Pts',(83.9855712457582,52.3952704422441,32.05)) ;
#16455=CARTESIAN_POINT('Ctrl Pts',(83.9875754901947,52.3601137381126,32.05)) ;
#16456=CARTESIAN_POINT('Ctrl Pts',(83.9895070553043,52.3262319112097,32.05)) ;
#16457=CARTESIAN_POINT('Ctrl Pts',(83.9936877046826,52.2925403287002,32.05)) ;
#16458=CARTESIAN_POINT('Ctrl Pts',(84.0002271476368,52.2592666431595,32.05)) ;
#16459=CARTESIAN_POINT('Ctrl Pts',(84.0055541232017,52.2321621770649,32.05)) ;
#16460=CARTESIAN_POINT('Ctrl Pts',(84.0124471142095,52.2053351471932,32.05)) ;
#16461=CARTESIAN_POINT('Ctrl Pts',(84.0209858286879,52.1789242467454,32.05)) ;
#16462=CARTESIAN_POINT('Ctrl Pts',(84.4250317703929,52.9637142832168,26.3685084761921)) ;
#16463=CARTESIAN_POINT('Ctrl Pts',(84.2056504531666,52.8563006564942,26.3895510373913)) ;
#16464=CARTESIAN_POINT('Ctrl Pts',(83.8854653412497,52.4085896297169,26.4316361597899)) ;
#16465=CARTESIAN_POINT('Ctrl Pts',(84.1861228684965,51.6345693759381,26.4947638433878)) ;
#16466=CARTESIAN_POINT('Ctrl Pts',(84.998175822282,51.4645124050219,26.5578915269857)) ;
#16467=CARTESIAN_POINT('Ctrl Pts',(85.5851072300976,52.0500826073856,26.6210192105835)) ;
#16468=CARTESIAN_POINT('Ctrl Pts',(85.4162279933292,52.8622720429723,26.6841468941814)) ;
#16469=CARTESIAN_POINT('Ctrl Pts',(84.6440981710049,53.1652507798167,26.7472745777793)) ;
#16470=CARTESIAN_POINT('Ctrl Pts',(83.9678955818182,52.6849989840867,26.8104022613771)) ;
#16471=CARTESIAN_POINT('Ctrl Pts',(83.9997130735727,51.8561601965047,26.873529944975)) ;
#16472=CARTESIAN_POINT('Ctrl Pts',(84.710785203412,51.4291552942847,26.9366576285728)) ;
#16473=CARTESIAN_POINT('Ctrl Pts',(85.4573524705639,51.7905235055957,26.9997853121707)) ;
#16474=CARTESIAN_POINT('Ctrl Pts',(85.5635501520105,52.6131307432408,27.0629129957686)) ;
#16475=CARTESIAN_POINT('Ctrl Pts',(84.933231811866,53.1522552393336,27.1260406793665)) ;
#16476=CARTESIAN_POINT('Ctrl Pts',(84.1370327822058,52.9198264637372,27.1891683629643)) ;
#16477=CARTESIAN_POINT('Ctrl Pts',(83.8957582643692,52.1262624336389,27.2522960465622)) ;
#16478=CARTESIAN_POINT('Ctrl Pts',(84.4278368710099,51.4899849375734,27.31542373016)) ;
#16479=CARTESIAN_POINT('Ctrl Pts',(85.2515726447776,51.5870214121571,27.3785514137579)) ;
#16480=CARTESIAN_POINT('Ctrl Pts',(85.6212301121436,52.3295240675631,27.4416790973558)) ;
#16481=CARTESIAN_POINT('Ctrl Pts',(85.2021548839321,53.0452982747,27.5048067809536)) ;
#16482=CARTESIAN_POINT('Ctrl Pts',(84.3737396709075,53.0863470831135,27.5679344645515)) ;
#16483=CARTESIAN_POINT('Ctrl Pts',(83.885956406241,52.4155085999048,27.6310621481494)) ;
#16484=CARTESIAN_POINT('Ctrl Pts',(84.1803997961088,51.6400991179717,27.6941898317473)) ;
#16485=CARTESIAN_POINT('Ctrl Pts',(84.9905075141293,51.4621040018937,27.7573175153451)) ;
#16486=CARTESIAN_POINT('Ctrl Pts',(85.5828815572153,52.042663878742,27.820445198943)) ;
#16487=CARTESIAN_POINT('Ctrl Pts',(85.4212402278205,52.8561925242217,27.8835728825408)) ;
#16488=CARTESIAN_POINT('Ctrl Pts',(84.6519189159883,53.1661949368354,27.9467005661387)) ;
#16489=CARTESIAN_POINT('Ctrl Pts',(83.9713913160093,52.6920230666678,28.0098282497366)) ;
#16490=CARTESIAN_POINT('Ctrl Pts',(83.9957453544512,51.8629490907966,28.0729559333345)) ;
#16491=CARTESIAN_POINT('Ctrl Pts',(84.7029330951489,51.4295413427059,28.1360836169323)) ;
#16492=CARTESIAN_POINT('Ctrl Pts',(85.4527309398621,51.7841678628247,28.1992113005302)) ;
#16493=CARTESIAN_POINT('Ctrl Pts',(85.5663399692938,52.6057819846142,28.2623389841281)) ;
#16494=CARTESIAN_POINT('Ctrl Pts',(84.9409088790051,53.1505688493595,28.3254666677259)) ;
#16495=CARTESIAN_POINT('Ctrl Pts',(84.1426462159603,52.9253278728757,28.3885943513238)) ;
#16496=CARTESIAN_POINT('Ctrl Pts',(83.8942265474451,52.1339717931037,28.4517220349216)) ;
#16497=CARTESIAN_POINT('Ctrl Pts',(84.4205464955366,51.4929225836516,28.5148497185195)) ;
#16498=CARTESIAN_POINT('Ctrl Pts',(85.2451237463938,51.5825280191257,28.5779774021174)) ;
#16499=CARTESIAN_POINT('Ctrl Pts',(85.6214608931572,52.3216674705582,28.6411050857152)) ;
#16500=CARTESIAN_POINT('Ctrl Pts',(85.2088564383358,53.0411911606195,28.7042327693131)) ;
#16501=CARTESIAN_POINT('Ctrl Pts',(84.3808450086281,53.08970764206,28.767360452911)) ;
#16502=CARTESIAN_POINT('Ctrl Pts',(83.8870330047499,52.4232944957884,28.8304881365088)) ;
#16503=CARTESIAN_POINT('Ctrl Pts',(84.1744729981709,51.6452617028549,28.8936158201067)) ;
#16504=CARTESIAN_POINT('Ctrl Pts',(84.9829429060078,51.4599695421454,28.9567435037046)) ;
#16505=CARTESIAN_POINT('Ctrl Pts',(85.5805274479185,52.0351647194261,29.0198711873024)) ;
#16506=CARTESIAN_POINT('Ctrl Pts',(85.4262278145717,52.8501177241122,29.0829988709003)) ;
#16507=CARTESIAN_POINT('Ctrl Pts',(84.6597328902445,53.1670440683605,29.1461265544982)) ;
#16508=CARTESIAN_POINT('Ctrl Pts',(83.9749576147278,52.6990274033377,29.209254238096)) ;
#16509=CARTESIAN_POINT('Ctrl Pts',(83.9918353744007,51.8697675418188,29.2723819216939)) ;
#16510=CARTESIAN_POINT('Ctrl Pts',(84.6950865774281,51.4300011013776,29.3355096052917)) ;
#16511=CARTESIAN_POINT('Ctrl Pts',(85.4480514094807,51.7778527053553,29.3986372888896)) ;
#16512=CARTESIAN_POINT('Ctrl Pts',(85.5690638483639,52.5984090814401,29.4617649724875)) ;
#16513=CARTESIAN_POINT('Ctrl Pts',(84.9485702146255,53.148812957869,29.5248926560853)) ;
#16514=CARTESIAN_POINT('Ctrl Pts',(84.1483091301802,52.9307786178669,29.5880203396833)) ;
#16515=CARTESIAN_POINT('Ctrl Pts',(83.8927643516779,52.1416945647534,29.6511480232811)) ;
#16516=CARTESIAN_POINT('Ctrl Pts',(84.4132829291257,51.4959258854032,29.714275706879)) ;
#16517=CARTESIAN_POINT('Ctrl Pts',(85.2386345831491,51.5780929341436,29.7774033904768)) ;
#16518=CARTESIAN_POINT('Ctrl Pts',(85.6216208325441,52.3138091222706,29.8405310740747)) ;
#16519=CARTESIAN_POINT('Ctrl Pts',(85.2155206857491,53.0370237843669,29.9036587576725)) ;
#16520=CARTESIAN_POINT('Ctrl Pts',(84.3879803592861,53.0930040020832,29.9667864412704)) ;
#16521=CARTESIAN_POINT('Ctrl Pts',(83.8881797597493,52.4310703668902,30.0299141248683)) ;
#16522=CARTESIAN_POINT('Ctrl Pts',(84.1685929896107,51.6504775170526,30.0930418084662)) ;
#16523=CARTESIAN_POINT('Ctrl Pts',(84.975359359988,51.4579033746375,30.156169492064)) ;
#16524=CARTESIAN_POINT('Ctrl Pts',(85.5781058187447,52.0276870907513,30.2192971756619)) ;
#16525=CARTESIAN_POINT('Ctrl Pts',(85.4311604255217,52.8439982006345,30.2824248592598)) ;
#16526=CARTESIAN_POINT('Ctrl Pts',(84.6675542030255,53.1678227112312,30.3455525428576)) ;
#16527=CARTESIAN_POINT('Ctrl Pts',(83.9785869226004,52.7059993000024,30.4086802264556)) ;
#16528=CARTESIAN_POINT('Ctrl Pts',(83.9879870313722,51.8766209697171,30.4718079100533)) ;
#16529=CARTESIAN_POINT('Ctrl Pts',(84.6872445240728,51.4305315890238,30.5349355936513)) ;
#16530=CARTESIAN_POINT('Ctrl Pts',(85.4433151290645,51.7715799971008,30.5980632772491)) ;
#16531=CARTESIAN_POINT('Ctrl Pts',(85.5717211395724,52.5910119186134,30.661190960847)) ;
#16532=CARTESIAN_POINT('Ctrl Pts',(84.9562154066652,53.1469880592007,30.7243186444448)) ;
#16533=CARTESIAN_POINT('Ctrl Pts',(84.1540209610485,52.9361780833212,30.7874463280427)) ;
#16534=CARTESIAN_POINT('Ctrl Pts',(83.8913718460322,52.1494302036142,30.8505740116406)) ;
#16535=CARTESIAN_POINT('Ctrl Pts',(84.406046739384,51.4989945619123,30.9137016952384)) ;
#16536=CARTESIAN_POINT('Ctrl Pts',(85.2321056902744,51.5737165276034,30.9768293788363)) ;
#16537=CARTESIAN_POINT('Ctrl Pts',(85.6217099208433,52.3059496735259,31.0399570624342)) ;
#16538=CARTESIAN_POINT('Ctrl Pts',(85.2221470677742,53.0327964447449,31.103084746032)) ;
#16539=CARTESIAN_POINT('Ctrl Pts',(84.3951451811447,53.0962359841114,31.1662124296299)) ;
#16540=CARTESIAN_POINT('Ctrl Pts',(83.8893964978933,52.438835396788,31.2293401132277)) ;
#16541=CARTESIAN_POINT('Ctrl Pts',(84.1627604121769,51.6557465123538,31.2924677968256)) ;
#16542=CARTESIAN_POINT('Ctrl Pts',(84.9677571597911,51.4559049037231,31.3555954804235)) ;
#16543=CARTESIAN_POINT('Ctrl Pts',(85.5756175422327,52.0202331507826,31.4187231640214)) ;
#16544=CARTESIAN_POINT('Ctrl Pts',(85.4360362883285,52.8378313051878,31.4818508476192)) ;
#16545=CARTESIAN_POINT('Ctrl Pts',(84.6753850015265,53.1685371869628,31.5449785312171)) ;
#16546=CARTESIAN_POINT('Ctrl Pts',(83.9822732966132,52.7129252324505,31.608106214815)) ;
#16547=CARTESIAN_POINT('Ctrl Pts',(83.9842121002569,51.883535113167,31.6712338984128)) ;
#16548=CARTESIAN_POINT('Ctrl Pts',(84.6793843110363,51.4310793972544,31.7343615820107)) ;
#16549=CARTESIAN_POINT('Ctrl Pts',(85.4385697001617,51.7654585545426,31.7974892656085)) ;
#16550=CARTESIAN_POINT('Ctrl Pts',(85.5742157004875,52.583371203896,31.8606169492065)) ;
#16551=CARTESIAN_POINT('Ctrl Pts',(84.9640410903861,53.1455422795452,31.9237446328042)) ;
#16552=CARTESIAN_POINT('Ctrl Pts',(84.1593673264954,52.9405973219202,31.9868723164022)) ;
#16553=CARTESIAN_POINT('Ctrl Pts',(83.9809659603427,52.4198895133115,32.0289574388007)) ;
#16554=CARTESIAN_POINT('Ctrl Pts',(84.0209858286879,52.1789242467453,32.05)) ;
#16555=CARTESIAN_POINT('Ctrl Pts',(84.3916481374235,53.031896930038,26.412338984128)) ;
#16556=CARTESIAN_POINT('Ctrl Pts',(84.149730015958,52.9134488182067,26.4333815453273)) ;
#16557=CARTESIAN_POINT('Ctrl Pts',(83.7966526355526,52.4197449243348,26.4754666677259)) ;
#16558=CARTESIAN_POINT('Ctrl Pts',(84.1281963837424,51.5662104112876,26.5385943513238)) ;
#16559=CARTESIAN_POINT('Ctrl Pts',(85.0236706547243,51.3786836726104,26.6017220349216)) ;
#16560=CARTESIAN_POINT('Ctrl Pts',(85.6708968880384,52.0244088653162,26.6648497185195)) ;
#16561=CARTESIAN_POINT('Ctrl Pts',(85.4846688708576,52.9200336387264,26.7279774021174)) ;
#16562=CARTESIAN_POINT('Ctrl Pts',(84.6332189912334,53.2541370518524,26.7911050857152)) ;
#16563=CARTESIAN_POINT('Ctrl Pts',(83.8875508451285,52.7245495112071,26.8542327693131)) ;
#16564=CARTESIAN_POINT('Ctrl Pts',(83.9226369132237,51.8105650159697,26.917360452911)) ;
#16565=CARTESIAN_POINT('Ctrl Pts',(84.7067567099872,51.3396943643224,26.9804881365088)) ;
#16566=CARTESIAN_POINT('Ctrl Pts',(85.5300180209343,51.7381855391541,27.0436158201067)) ;
#16567=CARTESIAN_POINT('Ctrl Pts',(85.647125274753,52.6452983241038,27.1067435037046)) ;
#16568=CARTESIAN_POINT('Ctrl Pts',(84.9520550167161,53.2398064936223,27.1698711873024)) ;
#16569=CARTESIAN_POINT('Ctrl Pts',(84.0740633262505,52.9835005625718,27.2329988709003)) ;
#16570=CARTESIAN_POINT('Ctrl Pts',(83.8080029394754,52.1084145623087,27.2961265544982)) ;
#16571=CARTESIAN_POINT('Ctrl Pts',(84.3947414029776,51.4067729707409,27.359254238096)) ;
#16572=CARTESIAN_POINT('Ctrl Pts',(85.3030986573388,51.5137778968747,27.4223819216939)) ;
#16573=CARTESIAN_POINT('Ctrl Pts',(85.7107306344894,52.3325570429296,27.4855096052918)) ;
#16574=CARTESIAN_POINT('Ctrl Pts',(85.2486042636415,53.12186195628,27.5486372888896)) ;
#16575=CARTESIAN_POINT('Ctrl Pts',(84.3350868563152,53.1671276641595,27.6117649724875)) ;
#16576=CARTESIAN_POINT('Ctrl Pts',(83.7971941471168,52.4273746728089,27.6748926560853)) ;
#16577=CARTESIAN_POINT('Ctrl Pts',(84.1218853863496,51.5723082177092,27.7380203396832)) ;
#16578=CARTESIAN_POINT('Ctrl Pts',(85.015214589611,51.3760278568469,27.8011480232811)) ;
#16579=CARTESIAN_POINT('Ctrl Pts',(85.6684425742004,52.0162280187436,27.8642757068789)) ;
#16580=CARTESIAN_POINT('Ctrl Pts',(85.4901960067496,52.9133295776232,27.9274033904768)) ;
#16581=CARTESIAN_POINT('Ctrl Pts',(84.6418431528474,53.2551782010954,27.9905310740747)) ;
#16582=CARTESIAN_POINT('Ctrl Pts',(83.891405692293,52.7322951701561,28.0536587576726)) ;
#16583=CARTESIAN_POINT('Ctrl Pts',(83.91826159463,51.8180513259923,28.1167864412704)) ;
#16584=CARTESIAN_POINT('Ctrl Pts',(84.6980979631779,51.3401200710782,28.1799141248683)) ;
#16585=CARTESIAN_POINT('Ctrl Pts',(85.5249217254073,51.7311769881103,28.2430418084661)) ;
#16586=CARTESIAN_POINT('Ctrl Pts',(85.6502016869332,52.637194635492,28.306169492064)) ;
#16587=CARTESIAN_POINT('Ctrl Pts',(84.9605207406171,53.2379468626393,28.3692971756619)) ;
#16588=CARTESIAN_POINT('Ctrl Pts',(84.0802534219525,52.9895671254908,28.4324248592598)) ;
#16589=CARTESIAN_POINT('Ctrl Pts',(83.8063138709369,52.116915895891,28.4955525428576)) ;
#16590=CARTESIAN_POINT('Ctrl Pts',(84.3867020951568,51.4100123980073,28.5586802264555)) ;
#16591=CARTESIAN_POINT('Ctrl Pts',(85.2959872706344,51.5088229024618,28.6218079100534)) ;
#16592=CARTESIAN_POINT('Ctrl Pts',(85.7109851233857,52.3238933462549,28.6849355936512)) ;
#16593=CARTESIAN_POINT('Ctrl Pts',(85.255994261444,53.1173329228348,28.7480632772491)) ;
#16594=CARTESIAN_POINT('Ctrl Pts',(84.3429221176562,53.1708334496735,28.8111909608469)) ;
#16595=CARTESIAN_POINT('Ctrl Pts',(83.7983813434201,52.435960405313,28.8743186444449)) ;
#16596=CARTESIAN_POINT('Ctrl Pts',(84.1153497349023,51.5780011493255,28.9374463280427)) ;
#16597=CARTESIAN_POINT('Ctrl Pts',(85.0068728775201,51.3736741263689,29.0005740116406)) ;
#16598=CARTESIAN_POINT('Ctrl Pts',(85.6658466298146,52.0079584789432,29.0637016952384)) ;
#16599=CARTESIAN_POINT('Ctrl Pts',(85.495695962866,52.9066307199022,29.1268293788363)) ;
#16600=CARTESIAN_POINT('Ctrl Pts',(84.6504598481846,53.256114562979,29.1899570624342)) ;
#16601=CARTESIAN_POINT('Ctrl Pts',(83.8953383530021,52.740019054718,29.253084746032)) ;
#16602=CARTESIAN_POINT('Ctrl Pts',(83.9139499465792,51.8255702290761,29.3162124296299)) ;
#16603=CARTESIAN_POINT('Ctrl Pts',(84.6894453812211,51.3406270602584,29.3793401132277)) ;
#16604=CARTESIAN_POINT('Ctrl Pts',(85.5197614719567,51.7242130813791,29.4424677968257)) ;
#16605=CARTESIAN_POINT('Ctrl Pts',(85.6532053871393,52.6290643219895,29.5055954804234)) ;
#16606=CARTESIAN_POINT('Ctrl Pts',(84.9689691169173,53.2360105903249,29.5687231640214)) ;
#16607=CARTESIAN_POINT('Ctrl Pts',(84.0864980811943,52.9955778195896,29.6318508476192)) ;
#16608=CARTESIAN_POINT('Ctrl Pts',(83.8047014653877,52.1254320194772,29.6949785312171)) ;
#16609=CARTESIAN_POINT('Ctrl Pts',(84.3786923504646,51.4133242256831,29.7581062148149)) ;
#16610=CARTESIAN_POINT('Ctrl Pts',(85.2888314827036,51.5039322060206,29.8212338984128)) ;
#16611=CARTESIAN_POINT('Ctrl Pts',(85.7111614931719,52.3152277183902,29.8843615820107)) ;
#16612=CARTESIAN_POINT('Ctrl Pts',(85.2633431197498,53.1127374365499,29.9474892656085)) ;
#16613=CARTESIAN_POINT('Ctrl Pts',(84.3507904751306,53.1744684411786,30.0106169492064)) ;
#16614=CARTESIAN_POINT('Ctrl Pts',(83.799645903314,52.4445350832003,30.0737446328043)) ;
#16615=CARTESIAN_POINT('Ctrl Pts',(84.1088656794546,51.5837527784458,30.1368723164022)) ;
#16616=CARTESIAN_POINT('Ctrl Pts',(84.9985102820616,51.371395703719,30.2)) ;
#16617=CARTESIAN_POINT('Ctrl Pts',(85.6631762293081,51.9997126816031,30.2631276835979)) ;
#16618=CARTESIAN_POINT('Ctrl Pts',(85.5011352955771,52.8998825444299,30.3262553671958)) ;
#16619=CARTESIAN_POINT('Ctrl Pts',(84.6590846359253,53.2569731949853,30.3893830507936)) ;
#16620=CARTESIAN_POINT('Ctrl Pts',(83.8993404957274,52.7477071667482,30.4525107343915)) ;
#16621=CARTESIAN_POINT('Ctrl Pts',(83.9097062674547,51.8331277021723,30.5156384179893)) ;
#16622=CARTESIAN_POINT('Ctrl Pts',(84.6807977222494,51.3412120443238,30.5787661015873)) ;
#16623=CARTESIAN_POINT('Ctrl Pts',(85.5145386386019,51.7172959846245,30.641893785185)) ;
#16624=CARTESIAN_POINT('Ctrl Pts',(85.656135658985,52.6209072566667,30.705021468783)) ;
#16625=CARTESIAN_POINT('Ctrl Pts',(84.9773996912245,53.2339982218002,30.7681491523808)) ;
#16626=CARTESIAN_POINT('Ctrl Pts',(84.0927966822388,53.0015319662604,30.8312768359787)) ;
#16627=CARTESIAN_POINT('Ctrl Pts',(83.8031659091507,52.1339623321091,30.8944045195766)) ;
#16628=CARTESIAN_POINT('Ctrl Pts',(84.370712794817,51.4167081439941,30.9575322031743)) ;
#16629=CARTESIAN_POINT('Ctrl Pts',(85.281631883761,51.499106215994,31.0206598867723)) ;
#16630=CARTESIAN_POINT('Ctrl Pts',(85.7112597334154,52.3065608770196,31.0837875703701)) ;
#16631=CARTESIAN_POINT('Ctrl Pts',(85.2706502227969,53.1080758269238,31.146915253968)) ;
#16632=CARTESIAN_POINT('Ctrl Pts',(84.3586913313503,53.1780324412071,31.2100429375659)) ;
#16633=CARTESIAN_POINT('Ctrl Pts',(83.800987635645,52.4530978061784,31.2731706211637)) ;
#16634=CARTESIAN_POINT('Ctrl Pts',(84.1024339276812,51.5895630519065,31.3362983047616)) ;
#16635=CARTESIAN_POINT('Ctrl Pts',(84.9901271161026,51.3691919320601,31.3994259883595)) ;
#16636=CARTESIAN_POINT('Ctrl Pts',(85.660432334855,51.9914930064843,31.4625536719573)) ;
#16637=CARTESIAN_POINT('Ctrl Pts',(85.5065120504696,52.8930821305178,31.5256813555552)) ;
#16638=CARTESIAN_POINT('Ctrl Pts',(84.6677198838439,53.2577610680321,31.588809039153)) ;
#16639=CARTESIAN_POINT('Ctrl Pts',(83.9034055669352,52.7553445927079,31.6519367227509)) ;
#16640=CARTESIAN_POINT('Ctrl Pts',(83.9055435417695,51.8407521280628,31.7150644063488)) ;
#16641=CARTESIAN_POINT('Ctrl Pts',(84.6721300380722,51.3418161282985,31.7781920899467)) ;
#16642=CARTESIAN_POINT('Ctrl Pts',(85.5093057169464,51.7105456929264,31.8413197735445)) ;
#16643=CARTESIAN_POINT('Ctrl Pts',(85.6588864834312,52.6124816196323,31.9044474571424)) ;
#16644=CARTESIAN_POINT('Ctrl Pts',(84.9860292989271,53.2324039187721,31.9675751407402)) ;
#16645=CARTESIAN_POINT('Ctrl Pts',(84.0986922739962,53.0064051884369,32.0307028243381)) ;
#16646=CARTESIAN_POINT('Ctrl Pts',(83.9019639294307,52.4322056326875,32.0727879467367)) ;
#16647=CARTESIAN_POINT('Ctrl Pts',(83.9460949953472,52.1664862662295,32.093830507936)) ;
#16648=CARTESIAN_POINT('Ctrl Pts',(84.3582645044542,53.1000795768593,26.456169492064)) ;
#16649=CARTESIAN_POINT('Ctrl Pts',(84.0938095787495,52.9705969799192,26.4772120532633)) ;
#16650=CARTESIAN_POINT('Ctrl Pts',(83.7078399298555,52.4309002189528,26.5192971756619)) ;
#16651=CARTESIAN_POINT('Ctrl Pts',(84.0702698989883,51.4978514466372,26.5824248592598)) ;
#16652=CARTESIAN_POINT('Ctrl Pts',(85.0491654871666,51.292854940199,26.6455525428576)) ;
#16653=CARTESIAN_POINT('Ctrl Pts',(85.7566865459792,51.9987351232468,26.7086802264555)) ;
#16654=CARTESIAN_POINT('Ctrl Pts',(85.553109748386,52.9777952344805,26.7718079100534)) ;
#16655=CARTESIAN_POINT('Ctrl Pts',(84.6223398114619,53.3430233238882,26.8349355936512)) ;
#16656=CARTESIAN_POINT('Ctrl Pts',(83.8072061084389,52.7641000383273,26.8980632772491)) ;
#16657=CARTESIAN_POINT('Ctrl Pts',(83.8455607528747,51.7649698354348,26.961190960847)) ;
#16658=CARTESIAN_POINT('Ctrl Pts',(84.7027282165623,51.2502334343599,27.0243186444448)) ;
#16659=CARTESIAN_POINT('Ctrl Pts',(85.6026835713044,51.6858475727128,27.0874463280427)) ;
#16660=CARTESIAN_POINT('Ctrl Pts',(85.7307003974957,52.6774659049666,27.1505740116405)) ;
#16661=CARTESIAN_POINT('Ctrl Pts',(84.9708782215659,53.3273577479112,27.2137016952384)) ;
#16662=CARTESIAN_POINT('Ctrl Pts',(84.0110938702955,53.0471746614063,27.2768293788363)) ;
#16663=CARTESIAN_POINT('Ctrl Pts',(83.7202476145812,52.0905666909787,27.3399570624342)) ;
#16664=CARTESIAN_POINT('Ctrl Pts',(84.3616459349454,51.3235610039085,27.403084746032)) ;
#16665=CARTESIAN_POINT('Ctrl Pts',(85.3546246698999,51.4405343815921,27.4662124296299)) ;
#16666=CARTESIAN_POINT('Ctrl Pts',(85.8002311568352,52.335590018296,27.5293401132277)) ;
#16667=CARTESIAN_POINT('Ctrl Pts',(85.295053643351,53.1984256378601,27.5924677968256)) ;
#16668=CARTESIAN_POINT('Ctrl Pts',(84.2964340417231,53.2479082452055,27.6555954804235)) ;
#16669=CARTESIAN_POINT('Ctrl Pts',(83.7084318879924,52.439240745713,27.7187231640213)) ;
#16670=CARTESIAN_POINT('Ctrl Pts',(84.0633709765903,51.5045173174467,27.7818508476192)) ;
#16671=CARTESIAN_POINT('Ctrl Pts',(85.0399216650928,51.2899517118001,27.8449785312171)) ;
#16672=CARTESIAN_POINT('Ctrl Pts',(85.7540035911854,51.9897921587451,27.908106214815)) ;
#16673=CARTESIAN_POINT('Ctrl Pts',(85.5591517856788,52.9704666310249,27.9712338984128)) ;
#16674=CARTESIAN_POINT('Ctrl Pts',(84.6317673897063,53.3441614653553,28.0343615820107)) ;
#16675=CARTESIAN_POINT('Ctrl Pts',(83.8114200685767,52.7725672736444,28.0974892656085)) ;
#16676=CARTESIAN_POINT('Ctrl Pts',(83.8407778348087,51.773153561188,28.1606169492064)) ;
#16677=CARTESIAN_POINT('Ctrl Pts',(84.6932628312068,51.2506987994505,28.2237446328043)) ;
#16678=CARTESIAN_POINT('Ctrl Pts',(85.5971125109525,51.678186113396,28.2868723164021)) ;
#16679=CARTESIAN_POINT('Ctrl Pts',(85.7340634045725,52.6686072863696,28.35)) ;
#16680=CARTESIAN_POINT('Ctrl Pts',(84.980132602229,53.3253248759193,28.4131276835978)) ;
#16681=CARTESIAN_POINT('Ctrl Pts',(84.0178606279449,53.0538063781057,28.4762553671958)) ;
#16682=CARTESIAN_POINT('Ctrl Pts',(83.7184011944283,52.0998599986783,28.5393830507936)) ;
#16683=CARTESIAN_POINT('Ctrl Pts',(84.3528576947773,51.3271022123631,28.6025107343915)) ;
#16684=CARTESIAN_POINT('Ctrl Pts',(85.3468507948749,51.4351177857977,28.6656384179893)) ;
#16685=CARTESIAN_POINT('Ctrl Pts',(85.8005093536141,52.3261192219517,28.7287661015872)) ;
#16686=CARTESIAN_POINT('Ctrl Pts',(85.3031320845523,53.1934746850499,28.7918937851851)) ;
#16687=CARTESIAN_POINT('Ctrl Pts',(84.3049992266842,53.2519592572871,28.8550214687829)) ;
#16688=CARTESIAN_POINT('Ctrl Pts',(83.7097296820902,52.4486263148374,28.9181491523808)) ;
#16689=CARTESIAN_POINT('Ctrl Pts',(84.0562264716337,51.5107405957961,28.9812768359787)) ;
#16690=CARTESIAN_POINT('Ctrl Pts',(85.0308028490327,51.2873787105924,29.0444045195765)) ;
#16691=CARTESIAN_POINT('Ctrl Pts',(85.7511658117106,51.9807522384602,29.1075322031744)) ;
#16692=CARTESIAN_POINT('Ctrl Pts',(85.5651641111605,52.9631437156923,29.1706598867723)) ;
#16693=CARTESIAN_POINT('Ctrl Pts',(84.6411868061246,53.3451850575975,29.2337875703701)) ;
#16694=CARTESIAN_POINT('Ctrl Pts',(83.8157190912767,52.7810107060983,29.296915253968)) ;
#16695=CARTESIAN_POINT('Ctrl Pts',(83.8360645187576,51.7813729163333,29.3600429375658)) ;
#16696=CARTESIAN_POINT('Ctrl Pts',(84.6838041850143,51.2512530191392,29.4231706211637)) ;
#16697=CARTESIAN_POINT('Ctrl Pts',(85.5914715344326,51.6705734574028,29.4862983047616)) ;
#16698=CARTESIAN_POINT('Ctrl Pts',(85.7373469259147,52.6597195625389,29.5494259883594)) ;
#16699=CARTESIAN_POINT('Ctrl Pts',(84.9893680192092,53.3232082227807,29.6125536719573)) ;
#16700=CARTESIAN_POINT('Ctrl Pts',(84.0246870322085,53.0603770213123,29.6756813555552)) ;
#16701=CARTESIAN_POINT('Ctrl Pts',(83.7166385790976,52.109169474201,29.7388090391531)) ;
#16702=CARTESIAN_POINT('Ctrl Pts',(84.3441017718036,51.330722565963,29.8019367227509)) ;
#16703=CARTESIAN_POINT('Ctrl Pts',(85.339028382258,51.4297714778975,29.8650644063488)) ;
#16704=CARTESIAN_POINT('Ctrl Pts',(85.8007021537997,52.3166463145098,29.9281920899466)) ;
#16705=CARTESIAN_POINT('Ctrl Pts',(85.3111655537503,53.1884510887328,29.9913197735445)) ;
#16706=CARTESIAN_POINT('Ctrl Pts',(84.3136005909752,53.2559328802739,30.0544474571424)) ;
#16707=CARTESIAN_POINT('Ctrl Pts',(83.7111120468786,52.4579997995102,30.1175751407403)) ;
#16708=CARTESIAN_POINT('Ctrl Pts',(84.0491383692985,51.5170280398391,30.1807028243381)) ;
#16709=CARTESIAN_POINT('Ctrl Pts',(85.0216612041352,51.2848880328004,30.243830507936)) ;
#16710=CARTESIAN_POINT('Ctrl Pts',(85.7482466398716,51.971738272455,30.3069581915338)) ;
#16711=CARTESIAN_POINT('Ctrl Pts',(85.5711101656323,52.9557668882253,30.3700858751317)) ;
#16712=CARTESIAN_POINT('Ctrl Pts',(84.6506150688253,53.3461236787394,30.4332135587296)) ;
#16713=CARTESIAN_POINT('Ctrl Pts',(83.8200940688542,52.7894150334941,30.4963412423275)) ;
#16714=CARTESIAN_POINT('Ctrl Pts',(83.8314255035372,51.7896344346275,30.5594689259253)) ;
#16715=CARTESIAN_POINT('Ctrl Pts',(84.6743509204261,51.2518924996238,30.6225966095232)) ;
#16716=CARTESIAN_POINT('Ctrl Pts',(85.5857621481392,51.663011972148,30.685724293121)) ;
#16717=CARTESIAN_POINT('Ctrl Pts',(85.7405501783976,52.65080259472,30.7488519767189)) ;
#16718=CARTESIAN_POINT('Ctrl Pts',(84.9985839757837,53.3210083843996,30.8119796603168)) ;
#16719=CARTESIAN_POINT('Ctrl Pts',(84.0315724034291,53.0668858491997,30.8751073439147)) ;
#16720=CARTESIAN_POINT('Ctrl Pts',(83.7149599722692,52.118494460604,30.9382350275124)) ;
#16721=CARTESIAN_POINT('Ctrl Pts',(84.3353788502498,51.334421726076,31.0013627111105)) ;
#16722=CARTESIAN_POINT('Ctrl Pts',(85.3311580772478,51.4244959043844,31.0644903947082)) ;
#16723=CARTESIAN_POINT('Ctrl Pts',(85.8008095459872,52.3071720805132,31.1276180783062)) ;
#16724=CARTESIAN_POINT('Ctrl Pts',(85.3191533778198,53.1833552091027,31.190745761904)) ;
#16725=CARTESIAN_POINT('Ctrl Pts',(84.3222374815559,53.2598288983029,31.2538734455018)) ;
#16726=CARTESIAN_POINT('Ctrl Pts',(83.7125787733965,52.4673602155687,31.3170011290997)) ;
#16727=CARTESIAN_POINT('Ctrl Pts',(84.0421074431857,51.5233795914594,31.3801288126976)) ;
#16728=CARTESIAN_POINT('Ctrl Pts',(85.0124970724141,51.282478960397,31.4432564962955)) ;
#16729=CARTESIAN_POINT('Ctrl Pts',(85.7452471274772,51.962752862186,31.5063841798933)) ;
#16730=CARTESIAN_POINT('Ctrl Pts',(85.5769878126107,52.9483329558477,31.5695118634912)) ;
#16731=CARTESIAN_POINT('Ctrl Pts',(84.6600547661612,53.3469849491015,31.632639547089)) ;
#16732=CARTESIAN_POINT('Ctrl Pts',(83.8245378372572,52.7977639529653,31.6957672306869)) ;
#16733=CARTESIAN_POINT('Ctrl Pts',(83.8268749832821,51.7979691429585,31.7588949142848)) ;
#16734=CARTESIAN_POINT('Ctrl Pts',(84.6648757651081,51.2525528593426,31.8220225978826)) ;
#16735=CARTESIAN_POINT('Ctrl Pts',(85.5800417337311,51.6556328313103,31.8851502814805)) ;
#16736=CARTESIAN_POINT('Ctrl Pts',(85.7435572663748,52.6415920353685,31.9482779650784)) ;
#16737=CARTESIAN_POINT('Ctrl Pts',(85.0080175074681,53.3192655579993,32.0114056486762)) ;
#16738=CARTESIAN_POINT('Ctrl Pts',(84.0380172214971,53.0722130549535,32.0745333322741)) ;
#16739=CARTESIAN_POINT('Ctrl Pts',(83.8229618985187,52.4445217520636,32.1166184546727)) ;
#16740=CARTESIAN_POINT('Ctrl Pts',(83.8712041620066,52.1540482857136,32.137661015872)) ;
#16741=CARTESIAN_POINT('Ctrl Pts',(84.3248808714849,53.1682622236805,26.5)) ;
#16742=CARTESIAN_POINT('Ctrl Pts',(84.037889141541,53.0277451416317,26.5210425611993)) ;
#16743=CARTESIAN_POINT('Ctrl Pts',(83.6190272241585,52.4420555135708,26.5631276835978)) ;
#16744=CARTESIAN_POINT('Ctrl Pts',(84.0123434142341,51.4294924819867,26.6262553671958)) ;
#16745=CARTESIAN_POINT('Ctrl Pts',(85.074660319609,51.2070262077874,26.6893830507936)) ;
#16746=CARTESIAN_POINT('Ctrl Pts',(85.8424762039199,51.9730613811773,26.7525107343915)) ;
#16747=CARTESIAN_POINT('Ctrl Pts',(85.6215506259147,53.0355568302346,26.8156384179893)) ;
#16748=CARTESIAN_POINT('Ctrl Pts',(84.6114606316903,53.4319095959239,26.8787661015872)) ;
#16749=CARTESIAN_POINT('Ctrl Pts',(83.7268613717493,52.8036505654477,26.941893785185)) ;
#16750=CARTESIAN_POINT('Ctrl Pts',(83.7684845925257,51.7193746548998,27.0050214687829)) ;
#16751=CARTESIAN_POINT('Ctrl Pts',(84.6986997231375,51.1607725043976,27.0681491523808)) ;
#16752=CARTESIAN_POINT('Ctrl Pts',(85.6753491216747,51.6335096062714,27.1312768359787)) ;
#16753=CARTESIAN_POINT('Ctrl Pts',(85.8142755202384,52.7096334858295,27.1944045195765)) ;
#16754=CARTESIAN_POINT('Ctrl Pts',(84.989701426416,53.4149090021999,27.2575322031744)) ;
#16755=CARTESIAN_POINT('Ctrl Pts',(83.9481244143403,53.1108487602408,27.3206598867722)) ;
#16756=CARTESIAN_POINT('Ctrl Pts',(83.6324922896873,52.0727188196486,27.3837875703701)) ;
#16757=CARTESIAN_POINT('Ctrl Pts',(84.3285504669132,51.240349037076,27.446915253968)) ;
#16758=CARTESIAN_POINT('Ctrl Pts',(85.406150682461,51.3672908663097,27.5100429375659)) ;
#16759=CARTESIAN_POINT('Ctrl Pts',(85.8897316791811,52.3386229936625,27.5731706211637)) ;
#16760=CARTESIAN_POINT('Ctrl Pts',(85.3415030230601,53.2749893194401,27.6362983047616)) ;
#16761=CARTESIAN_POINT('Ctrl Pts',(84.257781227131,53.3286888262516,27.6994259883595)) ;
#16762=CARTESIAN_POINT('Ctrl Pts',(83.6196696288681,52.451106818617,27.7625536719573)) ;
#16763=CARTESIAN_POINT('Ctrl Pts',(84.0048565668312,51.4367264171842,27.8256813555552)) ;
#16764=CARTESIAN_POINT('Ctrl Pts',(85.0646287405743,51.2038755667533,27.8888090391531)) ;
#16765=CARTESIAN_POINT('Ctrl Pts',(85.8395646081705,51.9633562987467,27.9519367227509)) ;
#16766=CARTESIAN_POINT('Ctrl Pts',(85.628107564608,53.0276036844266,28.0150644063488)) ;
#16767=CARTESIAN_POINT('Ctrl Pts',(84.6216916265653,53.4331447296151,28.0781920899466)) ;
#16768=CARTESIAN_POINT('Ctrl Pts',(83.7314344448605,52.8128393771328,28.1413197735445)) ;
#16769=CARTESIAN_POINT('Ctrl Pts',(83.7632940749875,51.7282557963837,28.2044474571424)) ;
#16770=CARTESIAN_POINT('Ctrl Pts',(84.6884276992357,51.1612775278227,28.2675751407402)) ;
#16771=CARTESIAN_POINT('Ctrl Pts',(85.6693032964976,51.6251952386817,28.3307028243381)) ;
#16772=CARTESIAN_POINT('Ctrl Pts',(85.817925122212,52.7000199372473,28.393830507936)) ;
#16773=CARTESIAN_POINT('Ctrl Pts',(84.9997444638408,53.4127028891992,28.4569581915338)) ;
#16774=CARTESIAN_POINT('Ctrl Pts',(83.9554678339372,53.1180456307208,28.5200858751317)) ;
#16775=CARTESIAN_POINT('Ctrl Pts',(83.6304885179198,52.0828041014656,28.5832135587296)) ;
#16776=CARTESIAN_POINT('Ctrl Pts',(84.3190132943977,51.2441920267188,28.6463412423274)) ;
#16777=CARTESIAN_POINT('Ctrl Pts',(85.3977143191155,51.3614126691337,28.7094689259253)) ;
#16778=CARTESIAN_POINT('Ctrl Pts',(85.8900335838426,52.3283450976483,28.7725966095232)) ;
#16779=CARTESIAN_POINT('Ctrl Pts',(85.3502699076606,53.2696164472651,28.835724293121)) ;
#16780=CARTESIAN_POINT('Ctrl Pts',(84.2670763357121,53.3330850649006,28.8988519767189)) ;
#16781=CARTESIAN_POINT('Ctrl Pts',(83.6210780207605,52.4612922243619,28.9619796603168)) ;
#16782=CARTESIAN_POINT('Ctrl Pts',(83.997103208365,51.4434800422666,29.0251073439146)) ;
#16783=CARTESIAN_POINT('Ctrl Pts',(85.0547328205452,51.201083294816,29.0882350275125)) ;
#16784=CARTESIAN_POINT('Ctrl Pts',(85.8364849936065,51.9535459979772,29.1513627111104)) ;
#16785=CARTESIAN_POINT('Ctrl Pts',(85.6346322594548,53.0196567114824,29.2144903947082)) ;
#16786=CARTESIAN_POINT('Ctrl Pts',(84.6319137640648,53.4342555522159,29.2776180783061)) ;
#16787=CARTESIAN_POINT('Ctrl Pts',(83.7360998295509,52.8220023574787,29.3407457619039)) ;
#16788=CARTESIAN_POINT('Ctrl Pts',(83.7581790909362,51.7371756035905,29.4038734455019)) ;
#16789=CARTESIAN_POINT('Ctrl Pts',(84.6781629888073,51.16187897802,29.4670011290997)) ;
#16790=CARTESIAN_POINT('Ctrl Pts',(85.6631815969086,51.6169338334265,29.5301288126976)) ;
#16791=CARTESIAN_POINT('Ctrl Pts',(85.82148846469,52.6903748030883,29.5932564962954)) ;
#16792=CARTESIAN_POINT('Ctrl Pts',(85.009766921501,53.4104058552366,29.6563841798933)) ;
#16793=CARTESIAN_POINT('Ctrl Pts',(83.9628759832229,53.125176223035,29.7195118634911)) ;
#16794=CARTESIAN_POINT('Ctrl Pts',(83.6285756928073,52.0929069289247,29.782639547089)) ;
#16795=CARTESIAN_POINT('Ctrl Pts',(84.3095111931425,51.248120906243,29.8457672306869)) ;
#16796=CARTESIAN_POINT('Ctrl Pts',(85.3892252818123,51.3556107497744,29.9088949142848)) ;
#16797=CARTESIAN_POINT('Ctrl Pts',(85.8902428144277,52.3180649106294,29.9720225978826)) ;
#16798=CARTESIAN_POINT('Ctrl Pts',(85.3589879877509,53.2641647409157,30.0351502814805)) ;
#16799=CARTESIAN_POINT('Ctrl Pts',(84.2764107068199,53.3373973193694,30.0982779650783)) ;
#16800=CARTESIAN_POINT('Ctrl Pts',(83.6225781904432,52.4714645158203,30.1614056486763)) ;
#16801=CARTESIAN_POINT('Ctrl Pts',(83.9894110591425,51.4503033012323,30.2245333322741)) ;
#16802=CARTESIAN_POINT('Ctrl Pts',(85.0448121262088,51.198380361882,30.287661015872)) ;
#16803=CARTESIAN_POINT('Ctrl Pts',(85.833317050435,51.9437638633069,30.3507886994698)) ;
#16804=CARTESIAN_POINT('Ctrl Pts',(85.6410850356875,53.0116512320208,30.4139163830677)) ;
#16805=CARTESIAN_POINT('Ctrl Pts',(84.6421455017252,53.4352741624935,30.4770440666656)) ;
#16806=CARTESIAN_POINT('Ctrl Pts',(83.7408476419811,52.8311229002399,30.5401717502634)) ;
#16807=CARTESIAN_POINT('Ctrl Pts',(83.7531447396198,51.7461411670827,30.6032994338613)) ;
#16808=CARTESIAN_POINT('Ctrl Pts',(84.6679041186026,51.1625729549238,30.6664271174591)) ;
#16809=CARTESIAN_POINT('Ctrl Pts',(85.6569856576766,51.6087279596716,30.729554801057)) ;
#16810=CARTESIAN_POINT('Ctrl Pts',(85.8249646978101,52.6806979327732,30.7926824846549)) ;
#16811=CARTESIAN_POINT('Ctrl Pts',(85.019768260343,53.4080185469991,30.8558101682527)) ;
#16812=CARTESIAN_POINT('Ctrl Pts',(83.9703481246194,53.132239732139,30.9189378518507)) ;
#16813=CARTESIAN_POINT('Ctrl Pts',(83.6267540353877,52.1030265890989,30.9820655354484)) ;
#16814=CARTESIAN_POINT('Ctrl Pts',(84.3000449056827,51.2521353081579,31.0451932190464)) ;
#16815=CARTESIAN_POINT('Ctrl Pts',(85.3806842707344,51.3498855927749,31.1083209026442)) ;
#16816=CARTESIAN_POINT('Ctrl Pts',(85.8903593585592,52.3077832840069,31.1714485862421)) ;
#16817=CARTESIAN_POINT('Ctrl Pts',(85.3676565328426,53.2586345912816,31.2345762698399)) ;
#16818=CARTESIAN_POINT('Ctrl Pts',(84.2857836317614,53.3416253553987,31.2977039534379)) ;
#16819=CARTESIAN_POINT('Ctrl Pts',(83.6241699111481,52.4816226249592,31.3608316370356)) ;
#16820=CARTESIAN_POINT('Ctrl Pts',(83.9817809586901,51.4571961310121,31.4239593206336)) ;
#16821=CARTESIAN_POINT('Ctrl Pts',(85.0348670287255,51.195765988734,31.4870870042314)) ;
#16822=CARTESIAN_POINT('Ctrl Pts',(85.8300619200994,51.9340127178877,31.5502146878293)) ;
#16823=CARTESIAN_POINT('Ctrl Pts',(85.6474635747518,53.0035837811777,31.6133423714272)) ;
#16824=CARTESIAN_POINT('Ctrl Pts',(84.6523896484787,53.4362088301708,31.676470055025)) ;
#16825=CARTESIAN_POINT('Ctrl Pts',(83.745670107579,52.8401833132227,31.7395977386229)) ;
#16826=CARTESIAN_POINT('Ctrl Pts',(83.7482064247947,51.7551861578542,31.8027254222207)) ;
#16827=CARTESIAN_POINT('Ctrl Pts',(84.657621492144,51.1632895903866,31.8658531058187)) ;
#16828=CARTESIAN_POINT('Ctrl Pts',(85.6507777505159,51.6007199696942,31.9289807894165)) ;
#16829=CARTESIAN_POINT('Ctrl Pts',(85.8282280493184,52.6707024511047,31.9921084730144)) ;
#16830=CARTESIAN_POINT('Ctrl Pts',(85.0300057160091,53.4061271972263,32.0552361566122)) ;
#16831=CARTESIAN_POINT('Ctrl Pts',(83.9773421689979,53.1380209214701,32.1183638402101)) ;
#16832=CARTESIAN_POINT('Ctrl Pts',(83.7439598676067,52.4568378714396,32.1604489626087)) ;
#16833=CARTESIAN_POINT('Ctrl Pts',(83.7963133286659,52.1416103051977,32.1814915238079)) ;
#16834=CARTESIAN_POINT('Ctrl Pts',(83.7847716506988,52.3000190203057,31.7710140831103)) ;
#16835=CARTESIAN_POINT('Ctrl Pts',(83.7847913222747,52.1388962198161,31.7815845294805)) ;
#16836=CARTESIAN_POINT('Ctrl Pts',(83.8230018066232,51.977763740797,31.7921549758506)) ;
#16837=CARTESIAN_POINT('Ctrl Pts',(83.8993528831503,51.837369589171,31.8027254222207)) ;
#16838=CARTESIAN_POINT('Ctrl Pts',(84.0513447805778,51.5578873020316,31.82376798342)) ;
#16839=CARTESIAN_POINT('Ctrl Pts',(84.3544831363609,51.3605884462091,31.8448105446193)) ;
#16840=CARTESIAN_POINT('Ctrl Pts',(84.6715783573144,51.3348440815158,31.8658531058186)) ;
#16841=CARTESIAN_POINT('Ctrl Pts',(84.988673578268,51.3090997168225,31.8868956670179)) ;
#16842=CARTESIAN_POINT('Ctrl Pts',(85.319725664392,51.4549098432584,31.9079382282172)) ;
#16843=CARTESIAN_POINT('Ctrl Pts',(85.5148267572544,51.7061453200447,31.9289807894165)) ;
#16844=CARTESIAN_POINT('Ctrl Pts',(85.7099278501168,51.9573807968311,31.9500233506158)) ;
#16845=CARTESIAN_POINT('Ctrl Pts',(85.7690779497176,52.3140416239679,31.9710659118151)) ;
#16846=CARTESIAN_POINT('Ctrl Pts',(85.6656159439665,52.6149428285566,31.9921084730144)) ;
#16847=CARTESIAN_POINT('Ctrl Pts',(85.5707356449191,52.8908856354625,32.0114056486762)) ;
#16848=CARTESIAN_POINT('Ctrl Pts',(85.3391003580094,53.1199352145346,32.0307028243381)) ;
#16849=CARTESIAN_POINT('Ctrl Pts',(85.0634162962529,53.2161025497301,32.05)) ;
#16850=CARTESIAN_POINT('',(84.3201226220477,51.6988956497206,26.5)) ;
#16851=CARTESIAN_POINT('Ctrl Pts',(84.3191917355919,51.698168494003,26.5)) ;
#16852=CARTESIAN_POINT('Ctrl Pts',(84.300816180799,51.7074226812205,26.5)) ;
#16853=CARTESIAN_POINT('Ctrl Pts',(84.2828934982845,51.7174706610443,26.5)) ;
#16854=CARTESIAN_POINT('Ctrl Pts',(84.2654813313523,51.7282988497271,26.5)) ;
#16855=CARTESIAN_POINT('Ctrl Pts',(84.2371864517476,51.7458947237105,26.5)) ;
#16856=CARTESIAN_POINT('Ctrl Pts',(84.2102385230316,51.7655481374333,26.5)) ;
#16857=CARTESIAN_POINT('Ctrl Pts',(84.1847000527494,51.7870133766027,26.5)) ;
#16858=CARTESIAN_POINT('Ctrl Pts',(84.1766854424536,51.793749705167,26.5)) ;
#16859=CARTESIAN_POINT('Ctrl Pts',(84.1688097413242,51.8006648199525,26.5)) ;
#16860=CARTESIAN_POINT('Ctrl Pts',(84.1610751954445,51.8077520287958,26.5)) ;
#16861=CARTESIAN_POINT('Ctrl Pts',(84.1544687104645,51.8138055889534,26.5)) ;
#16862=CARTESIAN_POINT('Ctrl Pts',(84.1479657078829,51.8199844792118,26.5)) ;
#16863=CARTESIAN_POINT('Ctrl Pts',(84.1415771515967,51.8262746779352,26.5)) ;
#16864=CARTESIAN_POINT('Ctrl Pts',(84.1161683064708,51.8512923310664,26.5)) ;
#16865=CARTESIAN_POINT('Ctrl Pts',(84.0925275072523,51.8781034129898,26.5)) ;
#16866=CARTESIAN_POINT('Ctrl Pts',(84.0707277650994,51.9064245173419,26.5)) ;
#16867=CARTESIAN_POINT('Ctrl Pts',(84.0550145507544,51.9268383176543,26.5)) ;
#16868=CARTESIAN_POINT('Ctrl Pts',(84.0402580944232,51.9480378802971,26.5)) ;
#16869=CARTESIAN_POINT('Ctrl Pts',(84.0264932335582,51.9699317066184,26.5)) ;
#16870=CARTESIAN_POINT('Ctrl Pts',(84.0220799558424,51.976951286167,26.5)) ;
#16871=CARTESIAN_POINT('Ctrl Pts',(84.0177694943993,51.9840412354974,26.5)) ;
#16872=CARTESIAN_POINT('Ctrl Pts',(84.0135690504379,51.9911877939304,26.5)) ;
#16873=CARTESIAN_POINT('Ctrl Pts',(83.9944337627959,52.0237442218985,26.5)) ;
#16874=CARTESIAN_POINT('Ctrl Pts',(83.9775429300529,52.0575290164857,26.5)) ;
#16875=CARTESIAN_POINT('Ctrl Pts',(83.9629762129376,52.0922399248873,26.5)) ;
#16876=CARTESIAN_POINT('Ctrl Pts',(83.9482943003256,52.1272253316746,26.5)) ;
#16877=CARTESIAN_POINT('Ctrl Pts',(83.9359725208531,52.1631526026432,26.5)) ;
#16878=CARTESIAN_POINT('Ctrl Pts',(83.9261260215936,52.1997538001073,26.5)) ;
#16879=CARTESIAN_POINT('Ctrl Pts',(83.9209993423921,52.2188105829134,26.5)) ;
#16880=CARTESIAN_POINT('Ctrl Pts',(83.9165443118937,52.2380506443706,26.5)) ;
#16881=CARTESIAN_POINT('Ctrl Pts',(83.9127819868296,52.2574390790074,26.5)) ;
#16882=CARTESIAN_POINT('Ctrl Pts',(83.9109170346052,52.2670497595544,26.5)) ;
#16883=CARTESIAN_POINT('Ctrl Pts',(83.9092220495422,52.2767000188718,26.5)) ;
#16884=CARTESIAN_POINT('Ctrl Pts',(83.9077033081333,52.2863606526602,26.5)) ;
#16885=CARTESIAN_POINT('Ctrl Pts',(83.901448178839,52.3261491993201,26.5)) ;
#16886=CARTESIAN_POINT('Ctrl Pts',(83.8981611108834,52.3661937690171,26.5)) ;
#16887=CARTESIAN_POINT('Ctrl Pts',(83.8979520164386,52.4061772604385,26.5)) ;
#16888=CARTESIAN_POINT('Ctrl Pts',(83.8977552168724,52.4438096986319,26.5)) ;
#16889=CARTESIAN_POINT('Ctrl Pts',(83.9002842209716,52.4813894674705,26.5)) ;
#16890=CARTESIAN_POINT('Ctrl Pts',(83.9053641490143,52.5187218857782,26.5)) ;
#16891=CARTESIAN_POINT('Ctrl Pts',(83.9076860678112,52.5357856794139,26.5)) ;
#16892=CARTESIAN_POINT('Ctrl Pts',(83.9105416295862,52.5527979619798,26.5)) ;
#16893=CARTESIAN_POINT('Ctrl Pts',(83.9139175930541,52.5697406004266,26.5)) ;
#16894=CARTESIAN_POINT('Ctrl Pts',(83.9157766295873,52.5790703766937,26.5)) ;
#16895=CARTESIAN_POINT('Ctrl Pts',(83.9177935077873,52.5883790360894,26.5)) ;
#16896=CARTESIAN_POINT('Ctrl Pts',(83.9199662851238,52.5976635435118,26.5)) ;
#16897=CARTESIAN_POINT('Ctrl Pts',(83.9218283515739,52.6056203504461,26.5)) ;
#16898=CARTESIAN_POINT('Ctrl Pts',(83.9238028858573,52.6135505871988,26.5)) ;
#16899=CARTESIAN_POINT('Ctrl Pts',(83.9258870491201,52.6214491569347,26.5)) ;
#16900=CARTESIAN_POINT('Ctrl Pts',(83.9359905736557,52.6597395320452,26.5)) ;
#16901=CARTESIAN_POINT('Ctrl Pts',(83.9486718000006,52.6973087601356,26.5)) ;
#16902=CARTESIAN_POINT('Ctrl Pts',(83.9637234370183,52.7339424030372,26.5)) ;
#16903=CARTESIAN_POINT('Ctrl Pts',(83.9791245442229,52.7714266089717,26.5)) ;
#16904=CARTESIAN_POINT('Ctrl Pts',(83.9970075859867,52.8079323713265,26.5)) ;
#16905=CARTESIAN_POINT('Ctrl Pts',(84.017204939325,52.8432325426417,26.5)) ;
#16906=CARTESIAN_POINT('Ctrl Pts',(84.0269030196574,52.8601824811523,26.5)) ;
#16907=CARTESIAN_POINT('Ctrl Pts',(84.0371354640833,52.8768543934362,26.5)) ;
#16908=CARTESIAN_POINT('Ctrl Pts',(84.0478878140445,52.8932221564482,26.5)) ;
#16909=CARTESIAN_POINT('Ctrl Pts',(84.0527399920078,52.9006083835783,26.5)) ;
#16910=CARTESIAN_POINT('Ctrl Pts',(84.0576980786753,52.9079326599278,26.5)) ;
#16911=CARTESIAN_POINT('Ctrl Pts',(84.0627609102679,52.9151925072417,26.5)) ;
#16912=CARTESIAN_POINT('Ctrl Pts',(84.0674266702075,52.9218829736626,26.5)) ;
#16913=CARTESIAN_POINT('Ctrl Pts',(84.0721756387589,52.9285104572487,26.5)) ;
#16914=CARTESIAN_POINT('Ctrl Pts',(84.077005709343,52.9350725962358,26.5)) ;
#16915=CARTESIAN_POINT('Ctrl Pts',(84.1020890028368,52.9691507852175,26.5)) ;
#16916=CARTESIAN_POINT('Ctrl Pts',(84.1293595617806,53.0014733682414,26.5)) ;
#16917=CARTESIAN_POINT('Ctrl Pts',(84.1586216298365,53.0318036918634,26.5)) ;
#16918=CARTESIAN_POINT('Ctrl Pts',(84.1876858283235,53.0619289223917,26.5)) ;
#16919=CARTESIAN_POINT('Ctrl Pts',(84.218715233164,53.0900899244461,26.5)) ;
#16920=CARTESIAN_POINT('Ctrl Pts',(84.2515653891372,53.1160380022807,26.5)) ;
#16921=CARTESIAN_POINT('Ctrl Pts',(84.2750831177722,53.1346144697293,26.5)) ;
#16922=CARTESIAN_POINT('Ctrl Pts',(84.2995350324732,53.1520564609265,26.5)) ;
#16923=CARTESIAN_POINT('Ctrl Pts',(84.3248808714849,53.1682622236805,26.5)) ;
#16924=CARTESIAN_POINT('Ctrl Pts',(84.3191917355918,51.698168494003,26.5)) ;
#16925=CARTESIAN_POINT('Ctrl Pts',(84.5014531352299,51.5693465265704,26.5192971756619)) ;
#16926=CARTESIAN_POINT('Ctrl Pts',(85.0144035932418,51.4807025406976,26.5596369125231)) ;
#16927=CARTESIAN_POINT('Ctrl Pts',(85.5851072300976,52.0500826073856,26.6210192105835)) ;
#16928=CARTESIAN_POINT('Ctrl Pts',(85.4162279933292,52.8622720429723,26.6841468941814)) ;
#16929=CARTESIAN_POINT('Ctrl Pts',(84.6440981710049,53.1652507798167,26.7472745777793)) ;
#16930=CARTESIAN_POINT('Ctrl Pts',(84.0893208210195,52.7712374725307,26.7990664661529)) ;
#16931=CARTESIAN_POINT('Ctrl Pts',(84.0119256629849,52.4132474725981,26.8298157933273)) ;
#16932=CARTESIAN_POINT('Ctrl Pts',(84.0121333942101,52.3001533432303,26.8395225593024)) ;
#16933=CARTESIAN_POINT('Origin',(84.75,52.3,26.5)) ;
#16934=CARTESIAN_POINT('',(85.71675,52.3,26.5)) ;
#16935=CARTESIAN_POINT('Origin',(84.75,52.3,26.5)) ;
#16936=CARTESIAN_POINT('',(85.1798773779524,51.6988956497206,26.5)) ;
#16937=CARTESIAN_POINT('Ctrl Pts',(85.1761635223117,53.1694011139097,26.5)) ;
#16938=CARTESIAN_POINT('Ctrl Pts',(85.1985358633421,53.1552500678604,26.5)) ;
#16939=CARTESIAN_POINT('Ctrl Pts',(85.2202463454435,53.140146062992,26.5)) ;
#16940=CARTESIAN_POINT('Ctrl Pts',(85.2412230990218,53.124086385618,26.5)) ;
#16941=CARTESIAN_POINT('Ctrl Pts',(85.2709792476784,53.1013052557575,26.5)) ;
#16942=CARTESIAN_POINT('Ctrl Pts',(85.299260215467,53.0766014077599,26.5)) ;
#16943=CARTESIAN_POINT('Ctrl Pts',(85.3259689576471,53.0501717378542,26.5)) ;
#16944=CARTESIAN_POINT('Ctrl Pts',(85.3365379879513,53.0397131404302,26.5)) ;
#16945=CARTESIAN_POINT('Ctrl Pts',(85.3468605118166,53.0289841303707,26.5)) ;
#16946=CARTESIAN_POINT('Ctrl Pts',(85.3569292400932,53.0179964066639,26.5)) ;
#16947=CARTESIAN_POINT('Ctrl Pts',(85.3659968469546,53.008101178971,26.5)) ;
#16948=CARTESIAN_POINT('Ctrl Pts',(85.3748614400538,52.9979924081547,26.5)) ;
#16949=CARTESIAN_POINT('Ctrl Pts',(85.3834989214389,52.9877012976841,26.5)) ;
#16950=CARTESIAN_POINT('Ctrl Pts',(85.4103301405326,52.9557332936509,26.5)) ;
#16951=CARTESIAN_POINT('Ctrl Pts',(85.4350085357348,52.9219718748241,26.5)) ;
#16952=CARTESIAN_POINT('Ctrl Pts',(85.4573964573398,52.8866925744485,26.5)) ;
#16953=CARTESIAN_POINT('Ctrl Pts',(85.47039247077,52.8662132164456,26.5)) ;
#16954=CARTESIAN_POINT('Ctrl Pts',(85.4826157668332,52.8452219775538,26.5)) ;
#16955=CARTESIAN_POINT('Ctrl Pts',(85.4940314606313,52.8237712759791,26.5)) ;
#16956=CARTESIAN_POINT('Ctrl Pts',(85.4983243680267,52.8157046724896,26.5)) ;
#16957=CARTESIAN_POINT('Ctrl Pts',(85.5025030055992,52.8075730922421,26.5)) ;
#16958=CARTESIAN_POINT('Ctrl Pts',(85.5065652899046,52.7993793320376,26.5)) ;
#16959=CARTESIAN_POINT('Ctrl Pts',(85.5103912382234,52.7916622692417,26.5)) ;
#16960=CARTESIAN_POINT('Ctrl Pts',(85.5141117268159,52.7838944289501,26.5)) ;
#16961=CARTESIAN_POINT('Ctrl Pts',(85.5177221829035,52.7760855289403,26.5)) ;
#16962=CARTESIAN_POINT('Ctrl Pts',(85.5345633035423,52.7396605942701,26.5)) ;
#16963=CARTESIAN_POINT('Ctrl Pts',(85.5490381405068,52.702295152328,26.5)) ;
#16964=CARTESIAN_POINT('Ctrl Pts',(85.5610187828003,52.6642349459369,26.5)) ;
#16965=CARTESIAN_POINT('Ctrl Pts',(85.5727220868461,52.627055790051,26.5)) ;
#16966=CARTESIAN_POINT('Ctrl Pts',(85.5820454153636,52.5892125751062,26.5)) ;
#16967=CARTESIAN_POINT('Ctrl Pts',(85.5888213376671,52.5509364354455,26.5)) ;
#16968=CARTESIAN_POINT('Ctrl Pts',(85.5920775623131,52.5325425248108,26.5)) ;
#16969=CARTESIAN_POINT('Ctrl Pts',(85.5947447687977,52.5140487672799,26.5)) ;
#16970=CARTESIAN_POINT('Ctrl Pts',(85.5968001972194,52.4954820749433,26.5)) ;
#16971=CARTESIAN_POINT('Ctrl Pts',(85.5978239244134,52.4862347435132,26.5)) ;
#16972=CARTESIAN_POINT('Ctrl Pts',(85.5986958482688,52.4769693367571,26.5)) ;
#16973=CARTESIAN_POINT('Ctrl Pts',(85.5994128958565,52.4676892980339,26.5)) ;
#16974=CARTESIAN_POINT('Ctrl Pts',(85.6000043549324,52.4600346273781,26.5)) ;
#16975=CARTESIAN_POINT('Ctrl Pts',(85.6004896712265,52.4523798650142,26.5)) ;
#16976=CARTESIAN_POINT('Ctrl Pts',(85.6008678559599,52.4447271034925,26.5)) ;
#16977=CARTESIAN_POINT('Ctrl Pts',(85.6026761979484,52.4081343783921,26.5)) ;
#16978=CARTESIAN_POINT('Ctrl Pts',(85.6020389100667,52.3715841873092,26.5)) ;
#16979=CARTESIAN_POINT('Ctrl Pts',(85.5988231850837,52.3352753060488,26.5)) ;
#16980=CARTESIAN_POINT('Ctrl Pts',(85.5958140040931,52.301298521387,26.5)) ;
#16981=CARTESIAN_POINT('Ctrl Pts',(85.5905459134365,52.2675325087441,26.5)) ;
#16982=CARTESIAN_POINT('Ctrl Pts',(85.5831173524095,52.2341559873963,26.5)) ;
#16983=CARTESIAN_POINT('Ctrl Pts',(85.579167991973,52.2164115127345,26.5)) ;
#16984=CARTESIAN_POINT('Ctrl Pts',(85.5746075077317,52.1987774139026,26.5)) ;
#16985=CARTESIAN_POINT('Ctrl Pts',(85.5694479139689,52.1812830263565,26.5)) ;
#16986=CARTESIAN_POINT('Ctrl Pts',(85.5668870334088,52.1725999712483,26.5)) ;
#16987=CARTESIAN_POINT('Ctrl Pts',(85.564178537469,52.1639513642352,26.5)) ;
#16988=CARTESIAN_POINT('Ctrl Pts',(85.561323752231,52.1553409885211,26.5)) ;
#16989=CARTESIAN_POINT('Ctrl Pts',(85.5588931172939,52.148009901141,26.5)) ;
#16990=CARTESIAN_POINT('Ctrl Pts',(85.5563563430786,52.1407066816808,26.5)) ;
#16991=CARTESIAN_POINT('Ctrl Pts',(85.5537193745141,52.133446803083,26.5)) ;
#16992=CARTESIAN_POINT('Ctrl Pts',(85.5409854555251,52.0983888554173,26.5)) ;
#16993=CARTESIAN_POINT('Ctrl Pts',(85.5258928434259,52.0642593605704,26.5)) ;
#16994=CARTESIAN_POINT('Ctrl Pts',(85.508587962428,52.0312868386761,26.5)) ;
#16995=CARTESIAN_POINT('Ctrl Pts',(85.4914700182882,51.9986705041284,26.5)) ;
#16996=CARTESIAN_POINT('Ctrl Pts',(85.4721863693872,51.9671853904795,26.5)) ;
#16997=CARTESIAN_POINT('Ctrl Pts',(85.4508457342638,51.9370907524033,26.5)) ;
#16998=CARTESIAN_POINT('Ctrl Pts',(85.4412665554904,51.9235821610897,26.5)) ;
#16999=CARTESIAN_POINT('Ctrl Pts',(85.4312725678517,51.9103543233663,26.5)) ;
#17000=CARTESIAN_POINT('Ctrl Pts',(85.4208721852388,51.8974339258895,26.5)) ;
#17001=CARTESIAN_POINT('Ctrl Pts',(85.4158879561118,51.8912420170114,26.5)) ;
#17002=CARTESIAN_POINT('Ctrl Pts',(85.4108093073963,51.8851194961188,26.5)) ;
#17003=CARTESIAN_POINT('Ctrl Pts',(85.4056404831104,51.8790734146626,26.5)) ;
#17004=CARTESIAN_POINT('Ctrl Pts',(85.3826093912735,51.8521334667038,26.5)) ;
#17005=CARTESIAN_POINT('Ctrl Pts',(85.3578991214674,51.8268335867781,26.5)) ;
#17006=CARTESIAN_POINT('Ctrl Pts',(85.3316223570636,51.8033912601801,26.5)) ;
#17007=CARTESIAN_POINT('Ctrl Pts',(85.3062984575833,51.7807990142998,26.5)) ;
#17008=CARTESIAN_POINT('Ctrl Pts',(85.2795187383892,51.7599316341875,26.5)) ;
#17009=CARTESIAN_POINT('Ctrl Pts',(85.2513665981943,51.741027670526,26.5)) ;
#17010=CARTESIAN_POINT('Ctrl Pts',(85.2284341168372,51.7256286709742,26.5)) ;
#17011=CARTESIAN_POINT('Ctrl Pts',(85.2045904738039,51.7115331865253,26.5)) ;
#17012=CARTESIAN_POINT('Ctrl Pts',(85.1798773779524,51.6988956497206,26.5)) ;
#17013=CARTESIAN_POINT('Origin',(84.75,52.3,26.5)) ;
#17014=CARTESIAN_POINT('Origin',(84.75,52.3,26.5)) ;
#17015=CARTESIAN_POINT('Origin',(84.75,52.3,25.7604774406976)) ;
#17016=CARTESIAN_POINT('Ctrl Pts',(85.1798773779524,51.6988956497206,26.5)) ;
#17017=CARTESIAN_POINT('Ctrl Pts',(85.3785638722607,51.8409855034509,26.5210425611993)) ;
#17018=CARTESIAN_POINT('Ctrl Pts',(85.6206111574732,52.3353302012154,26.5631276835978)) ;
#17019=CARTESIAN_POINT('Ctrl Pts',(85.1965387349045,53.0492386288041,26.6262553671958)) ;
#17020=CARTESIAN_POINT('Ctrl Pts',(84.3675652084279,53.0831821640869,26.6893830507936)) ;
#17021=CARTESIAN_POINT('Ctrl Pts',(84.0256471893491,52.6053061792988,26.7341237419609)) ;
#17022=CARTESIAN_POINT('Ctrl Pts',(84.0100192177397,52.3312588893219,26.7578218719289)) ;
#17023=CARTESIAN_POINT('Ctrl Pts',(84.010254873815,52.3005215753354,26.7604774406976)) ;
#17024=CARTESIAN_POINT('Ctrl Pts',(85.3123598851629,51.5136432603077,26.3685084761921)) ;
#17025=CARTESIAN_POINT('Ctrl Pts',(85.5722789222031,51.6995233226808,26.3895510373913)) ;
#17026=CARTESIAN_POINT('Ctrl Pts',(85.8889219708895,52.3462185007104,26.4316361597899)) ;
#17027=CARTESIAN_POINT('Ctrl Pts',(85.3341560513787,53.2801440384254,26.4947638433878)) ;
#17028=CARTESIAN_POINT('Ctrl Pts',(84.2497038771959,53.3245485211515,26.5578915269856)) ;
#17029=CARTESIAN_POINT('Ctrl Pts',(83.6185883054696,52.4424804272665,26.6210192105836)) ;
#17030=CARTESIAN_POINT('Ctrl Pts',(84.01154584563,51.4309028921684,26.6841468941814)) ;
#17031=CARTESIAN_POINT('Ctrl Pts',(85.0731334617142,51.2063834341436,26.7472745777793)) ;
#17032=CARTESIAN_POINT('Ctrl Pts',(85.8421357429227,51.9717988075231,26.8104022613771)) ;
#17033=CARTESIAN_POINT('Ctrl Pts',(85.622441895197,53.0344000170724,26.873529944975)) ;
#17034=CARTESIAN_POINT('Ctrl Pts',(84.6129062855387,53.4321114217142,26.9366576285728)) ;
#17035=CARTESIAN_POINT('Ctrl Pts',(83.7274888206984,52.8049270108724,26.9997853121707)) ;
#17036=CARTESIAN_POINT('Ctrl Pts',(83.7677572516237,51.7206200598891,27.0629129957686)) ;
#17037=CARTESIAN_POINT('Ctrl Pts',(84.6972605634971,51.1608347951476,27.1260406793665)) ;
#17038=CARTESIAN_POINT('Ctrl Pts',(85.6745086642054,51.6323445107387,27.1891683629643)) ;
#17039=CARTESIAN_POINT('Ctrl Pts',(85.8147908759896,52.7082898034173,27.2522960465622)) ;
#17040=CARTESIAN_POINT('Ctrl Pts',(84.9911078932332,53.4146061239167,27.3154237301601)) ;
#17041=CARTESIAN_POINT('Ctrl Pts',(83.9491477911621,53.1118594344693,27.3785514137579)) ;
#17042=CARTESIAN_POINT('Ctrl Pts',(83.6322065542242,52.074128788224,27.4416790973558)) ;
#17043=CARTESIAN_POINT('Ctrl Pts',(84.3272140762793,51.2408814903139,27.5048067809536)) ;
#17044=CARTESIAN_POINT('Ctrl Pts',(85.4049735927635,51.3664639428714,27.5679344645516)) ;
#17045=CARTESIAN_POINT('Ctrl Pts',(85.8897794667379,52.3371852294877,27.6310621481493)) ;
#17046=CARTESIAN_POINT('Ctrl Pts',(85.3427324518969,53.2742423778523,27.6941898317473)) ;
#17047=CARTESIAN_POINT('Ctrl Pts',(84.2590792708789,53.3293088996161,27.7573175153451)) ;
#17048=CARTESIAN_POINT('Ctrl Pts',(83.6198611629693,52.4525325590144,27.820445198943)) ;
#17049=CARTESIAN_POINT('Ctrl Pts',(84.0037681905173,51.437667083614,27.8835728825408)) ;
#17050=CARTESIAN_POINT('Ctrl Pts',(85.0632457725477,51.2034795676857,27.9467005661387)) ;
#17051=CARTESIAN_POINT('Ctrl Pts',(85.839139061397,51.9619821345739,28.0098282497366)) ;
#17052=CARTESIAN_POINT('Ctrl Pts',(85.6290246908954,53.0264953992789,28.0729559333345)) ;
#17053=CARTESIAN_POINT('Ctrl Pts',(84.623121142821,53.4333056639836,28.1360836169323)) ;
#17054=CARTESIAN_POINT('Ctrl Pts',(83.7320821968977,52.8141238357924,28.1992113005302)) ;
#17055=CARTESIAN_POINT('Ctrl Pts',(83.7625736468539,51.7295009469655,28.2623389841281)) ;
#17056=CARTESIAN_POINT('Ctrl Pts',(84.6869913012024,51.1613561240314,28.3254666677259)) ;
#17057=CARTESIAN_POINT('Ctrl Pts',(85.6684513129697,51.6240361266255,28.3885943513238)) ;
#17058=CARTESIAN_POINT('Ctrl Pts',(85.818428861758,52.6986724717933,28.4517220349216)) ;
#17059=CARTESIAN_POINT('Ctrl Pts',(85.0011478863907,53.4123869432734,28.5148497185195)) ;
#17060=CARTESIAN_POINT('Ctrl Pts',(83.9565004080862,53.1190472330921,28.5779774021174)) ;
#17061=CARTESIAN_POINT('Ctrl Pts',(83.6302154447458,52.0842164922485,28.6411050857152)) ;
#17062=CARTESIAN_POINT('Ctrl Pts',(84.3176817895697,51.2447365554831,28.7042327693131)) ;
#17063=CARTESIAN_POINT('Ctrl Pts',(85.3965298062611,51.3605963689557,28.767360452911)) ;
#17064=CARTESIAN_POINT('Ctrl Pts',(85.890068413398,52.3269069726244,28.8304881365088)) ;
#17065=CARTESIAN_POINT('Ctrl Pts',(85.351492548107,53.2688584452722,28.8936158201067)) ;
#17066=CARTESIAN_POINT('Ctrl Pts',(84.2683799193525,53.3336934121491,28.9567435037046)) ;
#17067=CARTESIAN_POINT('Ctrl Pts',(83.6212824012761,52.4627161784649,29.0198711873024)) ;
#17068=CARTESIAN_POINT('Ctrl Pts',(83.9960233581859,51.4444304844127,29.0829988709003)) ;
#17069=CARTESIAN_POINT('Ctrl Pts',(85.0533463380197,51.2006997809454,29.1461265544982)) ;
#17070=CARTESIAN_POINT('Ctrl Pts',(85.8360470741805,51.9521757267418,29.209254238096)) ;
#17071=CARTESIAN_POINT('Ctrl Pts',(85.6355393556322,53.0185402020971,29.2723819216939)) ;
#17072=CARTESIAN_POINT('Ctrl Pts',(84.6333446732919,53.4344035909473,29.3355096052918)) ;
#17073=CARTESIAN_POINT('Ctrl Pts',(83.7367591364786,52.8232809234949,29.3986372888896)) ;
#17074=CARTESIAN_POINT('Ctrl Pts',(83.7574699189085,51.7384271992591,29.4617649724875)) ;
#17075=CARTESIAN_POINT('Ctrl Pts',(84.6767273578161,51.1619705222136,29.5248926560853)) ;
#17076=CARTESIAN_POINT('Ctrl Pts',(85.6623191969598,51.6157824503406,29.5880203396833)) ;
#17077=CARTESIAN_POINT('Ctrl Pts',(85.8219800344285,52.6890228504728,29.6511480232811)) ;
#17078=CARTESIAN_POINT('Ctrl Pts',(85.011167438299,53.4100772682907,29.714275706879)) ;
#17079=CARTESIAN_POINT('Ctrl Pts',(83.9639175462777,53.126168474558,29.7774033904768)) ;
#17080=CARTESIAN_POINT('Ctrl Pts',(83.6283153654585,52.0943217244413,29.8405310740747)) ;
#17081=CARTESIAN_POINT('Ctrl Pts',(84.3081846521447,51.2486774182948,29.9036587576725)) ;
#17082=CARTESIAN_POINT('Ctrl Pts',(85.3880334569927,51.3548051628574,29.9667864412704)) ;
#17083=CARTESIAN_POINT('Ctrl Pts',(85.8902646758111,52.3166265300249,30.0299141248683)) ;
#17084=CARTESIAN_POINT('Ctrl Pts',(85.3602037440254,53.2633957458814,30.0930418084661)) ;
#17085=CARTESIAN_POINT('Ctrl Pts',(84.2777197225921,53.3379938882152,30.156169492064)) ;
#17086=CARTESIAN_POINT('Ctrl Pts',(83.6227954016365,52.4728865692609,30.2192971756619)) ;
#17087=CARTESIAN_POINT('Ctrl Pts',(83.9883398224533,51.4512634411337,30.2824248592598)) ;
#17088=CARTESIAN_POINT('Ctrl Pts',(85.0434222421183,51.198009364737,30.3455525428576)) ;
#17089=CARTESIAN_POINT('Ctrl Pts',(85.8328667938476,51.9423975962189,30.4086802264555)) ;
#17090=CARTESIAN_POINT('Ctrl Pts',(85.6419820280726,53.0105265892964,30.4718079100534)) ;
#17091=CARTESIAN_POINT('Ctrl Pts',(84.6435776875471,53.4354092934174,30.5349355936512)) ;
#17092=CARTESIAN_POINT('Ctrl Pts',(83.7415184502553,52.8323954698803,30.5980632772491)) ;
#17093=CARTESIAN_POINT('Ctrl Pts',(83.7524468812573,51.747399105686,30.6611909608469)) ;
#17094=CARTESIAN_POINT('Ctrl Pts',(84.6664693715499,51.1626774404569,30.7243186444448)) ;
#17095=CARTESIAN_POINT('Ctrl Pts',(85.6561129110516,51.6075843975507,30.7874463280427)) ;
#17096=CARTESIAN_POINT('Ctrl Pts',(85.8254440585195,52.67934160617,30.8505740116405)) ;
#17097=CARTESIAN_POINT('Ctrl Pts',(85.0211657560265,53.4076773391265,30.9137016952384)) ;
#17098=CARTESIAN_POINT('Ctrl Pts',(83.9713985949548,53.1332225655791,30.9768293788363)) ;
#17099=CARTESIAN_POINT('Ctrl Pts',(83.6265064688367,52.1044436470692,31.0399570624342)) ;
#17100=CARTESIAN_POINT('Ctrl Pts',(84.2987234489242,51.2527038135746,31.103084746032)) ;
#17101=CARTESIAN_POINT('Ctrl Pts',(85.379485205345,51.3490906723475,31.1662124296299)) ;
#17102=CARTESIAN_POINT('Ctrl Pts',(85.8903683017345,52.3063449925798,31.2293401132277)) ;
#17103=CARTESIAN_POINT('Ctrl Pts',(85.3688652011076,53.2578542033979,31.2924677968256)) ;
#17104=CARTESIAN_POINT('Ctrl Pts',(84.2870981863241,53.3422110355567,31.3555954804235)) ;
#17105=CARTESIAN_POINT('Ctrl Pts',(83.6243995029531,52.483040758174,31.4187231640213)) ;
#17106=CARTESIAN_POINT('Ctrl Pts',(83.9807193000769,51.4581697543765,31.4818508476192)) ;
#17107=CARTESIAN_POINT('Ctrl Pts',(85.0334720753324,51.195399697593,31.5449785312171)) ;
#17108=CARTESIAN_POINT('Ctrl Pts',(85.8296029766522,51.9326664778211,31.608106214815)) ;
#17109=CARTESIAN_POINT('Ctrl Pts',(85.6483430569928,53.0024188060892,31.6712338984128)) ;
#17110=CARTESIAN_POINT('Ctrl Pts',(84.6538378769964,53.4363965712052,31.7343615820107)) ;
#17111=CARTESIAN_POINT('Ctrl Pts',(83.7463221504495,52.8413167917181,31.7974892656085)) ;
#17112=CARTESIAN_POINT('Ctrl Pts',(83.7475813626246,51.7567203683836,31.8606169492064)) ;
#17113=CARTESIAN_POINT('Ctrl Pts',(84.6560601317181,51.1628562405876,31.9237446328043)) ;
#17114=CARTESIAN_POINT('Ctrl Pts',(85.6501671264575,51.6007299877531,31.9868723164022)) ;
#17115=CARTESIAN_POINT('Ctrl Pts',(85.7681319415962,52.3110551076506,32.0289574388007)) ;
#17116=CARTESIAN_POINT('Ctrl Pts',(85.6645587247976,52.6133494876276,32.05)) ;
#17117=CARTESIAN_POINT('Ctrl Pts',(85.2681990494261,51.5753940567787,26.412338984128)) ;
#17118=CARTESIAN_POINT('Ctrl Pts',(85.507707238889,51.7466773829375,26.4333815453273)) ;
#17119=CARTESIAN_POINT('Ctrl Pts',(85.799485033084,52.3425890675454,26.4754666677259)) ;
#17120=CARTESIAN_POINT('Ctrl Pts',(85.288283612554,53.2031755685516,26.5385943513238)) ;
#17121=CARTESIAN_POINT('Ctrl Pts',(84.2889909876065,53.2440930687966,26.6017220349216)) ;
#17122=CARTESIAN_POINT('Ctrl Pts',(83.7074354784476,52.4312917651477,26.6648497185195)) ;
#17123=CARTESIAN_POINT('Ctrl Pts',(84.0695349616227,51.4991511005327,26.7279774021173)) ;
#17124=CARTESIAN_POINT('Ctrl Pts',(85.0477585299305,51.2922626420993,26.7911050857153)) ;
#17125=CARTESIAN_POINT('Ctrl Pts',(85.7563728206055,51.9975716966143,26.8542327693131)) ;
#17126=CARTESIAN_POINT('Ctrl Pts',(85.5539310283299,52.9767292632104,26.917360452911)) ;
#17127=CARTESIAN_POINT('Ctrl Pts',(84.6236719414196,53.3432093007606,26.9804881365088)) ;
#17128=CARTESIAN_POINT('Ctrl Pts',(83.807784285257,52.7652762474119,27.0436158201067)) ;
#17129=CARTESIAN_POINT('Ctrl Pts',(83.8448905283904,51.7661174416184,27.1067435037046)) ;
#17130=CARTESIAN_POINT('Ctrl Pts',(84.7014020708374,51.2502908335599,27.1698711873024)) ;
#17131=CARTESIAN_POINT('Ctrl Pts',(85.6019091130382,51.6847739694679,27.2329988709003)) ;
#17132=CARTESIAN_POINT('Ctrl Pts',(85.7311752835383,52.6762277388613,27.2961265544982)) ;
#17133=CARTESIAN_POINT('Ctrl Pts',(84.9721742417605,53.3270786539669,27.359254238096)) ;
#17134=CARTESIAN_POINT('Ctrl Pts',(84.0120368836758,53.0481059696989,27.4223819216939)) ;
#17135=CARTESIAN_POINT('Ctrl Pts',(83.7199843172707,52.0918659379462,27.4855096052918)) ;
#17136=CARTESIAN_POINT('Ctrl Pts',(84.3604144880119,51.3240516448113,27.5486372888896)) ;
#17137=CARTESIAN_POINT('Ctrl Pts',(85.3535400143643,51.4397723945604,27.6117649724875)) ;
#17138=CARTESIAN_POINT('Ctrl Pts',(85.8002751917446,52.3342651584539,27.6748926560853)) ;
#17139=CARTESIAN_POINT('Ctrl Pts',(85.2961865279525,53.197737351887,27.7380203396833)) ;
#17140=CARTESIAN_POINT('Ctrl Pts',(84.2976301530641,53.2484796256268,27.8011480232811)) ;
#17141=CARTESIAN_POINT('Ctrl Pts',(83.7086083813586,52.4405545259773,27.864275706879)) ;
#17142=CARTESIAN_POINT('Ctrl Pts',(84.0623680679795,51.5053841154929,27.9274033904768)) ;
#17143=CARTESIAN_POINT('Ctrl Pts',(85.0386472983824,51.2895868096337,27.9905310740747)) ;
#17144=CARTESIAN_POINT('Ctrl Pts',(85.7536114616269,51.9885259045423,28.0536587576725)) ;
#17145=CARTESIAN_POINT('Ctrl Pts',(85.5599968921362,52.9694453769754,28.1167864412704)) ;
#17146=CARTESIAN_POINT('Ctrl Pts',(84.6330846493196,53.3443097619158,28.1799141248683)) ;
#17147=CARTESIAN_POINT('Ctrl Pts',(83.8120169541277,52.7737508667029,28.2430418084662)) ;
#17148=CARTESIAN_POINT('Ctrl Pts',(83.840113980249,51.7743009329421,28.306169492064)) ;
#17149=CARTESIAN_POINT('Ctrl Pts',(84.6919392302261,51.2507712236786,28.3692971756619)) ;
#17150=CARTESIAN_POINT('Ctrl Pts',(85.5963274317427,51.6771180237589,28.4324248592598)) ;
#17151=CARTESIAN_POINT('Ctrl Pts',(85.7345275866039,52.6673656342962,28.4955525428576)) ;
#17152=CARTESIAN_POINT('Ctrl Pts',(84.9814258172154,53.3250337405045,28.5586802264555)) ;
#17153=CARTESIAN_POINT('Ctrl Pts',(84.0188121164073,53.0547293269334,28.6218079100534)) ;
#17154=CARTESIAN_POINT('Ctrl Pts',(83.7181495650662,52.101161477643,28.6849355936512)) ;
#17155=CARTESIAN_POINT('Ctrl Pts',(84.3516307499784,51.3276039805287,28.7480632772491)) ;
#17156=CARTESIAN_POINT('Ctrl Pts',(85.3457592991063,51.4343655878059,28.8111909608469)) ;
#17157=CARTESIAN_POINT('Ctrl Pts',(85.8005414480841,52.324794029597,28.8743186444448)) ;
#17158=CARTESIAN_POINT('Ctrl Pts',(85.3042587138404,53.19277620722,28.9374463280427)) ;
#17159=CARTESIAN_POINT('Ctrl Pts',(84.3062004428825,53.2525198324174,29.0005740116406)) ;
#17160=CARTESIAN_POINT('Ctrl Pts',(83.7099180130712,52.4499384490811,29.0637016952384)) ;
#17161=CARTESIAN_POINT('Ctrl Pts',(84.0552314196198,51.511616401894,29.1268293788363)) ;
#17162=CARTESIAN_POINT('Ctrl Pts',(85.0295252438092,51.2870253131891,29.1899570624341)) ;
#17163=CARTESIAN_POINT('Ctrl Pts',(85.7507622810954,51.9794895714913,29.253084746032)) ;
#17164=CARTESIAN_POINT('Ctrl Pts',(85.5659999751495,52.9621148832358,29.3162124296299)) ;
#17165=CARTESIAN_POINT('Ctrl Pts',(84.6425053493224,53.3453214711857,29.3793401132277)) ;
#17166=CARTESIAN_POINT('Ctrl Pts',(83.8163266243389,52.7821888692492,29.4424677968256)) ;
#17167=CARTESIAN_POINT('Ctrl Pts',(83.8354110363875,51.7825262270562,29.5055954804235)) ;
#17168=CARTESIAN_POINT('Ctrl Pts',(84.6824812908417,51.2513373745766,29.5687231640214)) ;
#17169=CARTESIAN_POINT('Ctrl Pts',(85.5906768567795,51.6695124897975,29.6318508476192)) ;
#17170=CARTESIAN_POINT('Ctrl Pts',(85.7377998938059,52.6584737756706,29.6949785312171)) ;
#17171=CARTESIAN_POINT('Ctrl Pts',(84.9906585566257,53.3229054390162,29.7581062148149)) ;
#17172=CARTESIAN_POINT('Ctrl Pts',(84.0256468036988,53.0612913535924,29.8212338984128)) ;
#17173=CARTESIAN_POINT('Ctrl Pts',(83.71639869466,52.110473169061,29.8843615820107)) ;
#17174=CARTESIAN_POINT('Ctrl Pts',(84.3428794010367,51.3312353763962,29.9474892656085)) ;
#17175=CARTESIAN_POINT('Ctrl Pts',(85.3379301487158,51.4290291518787,30.0106169492064)) ;
#17176=CARTESIAN_POINT('Ctrl Pts',(85.8007222984588,52.3153208866449,30.0737446328043)) ;
#17177=CARTESIAN_POINT('Ctrl Pts',(85.3122858394649,53.1877424811199,30.1368723164021)) ;
#17178=CARTESIAN_POINT('Ctrl Pts',(84.3148068127324,53.2564826019327,30.2)) ;
#17179=CARTESIAN_POINT('Ctrl Pts',(83.7113122009735,52.4593101823462,30.2631276835979)) ;
#17180=CARTESIAN_POINT('Ctrl Pts',(84.0481512543769,51.5179127821498,30.3262553671957)) ;
#17181=CARTESIAN_POINT('Ctrl Pts',(85.0203804644637,51.2845461692128,30.3893830507936)) ;
#17182=CARTESIAN_POINT('Ctrl Pts',(85.7478317409044,51.9704792951971,30.4525107343915)) ;
#17183=CARTESIAN_POINT('Ctrl Pts',(85.5719367192567,52.9547305611222,30.5156384179893)) ;
#17184=CARTESIAN_POINT('Ctrl Pts',(84.6519347883698,53.3462481981409,30.5787661015872)) ;
#17185=CARTESIAN_POINT('Ctrl Pts',(83.8207122000886,52.7905876711508,30.6418937851851)) ;
#17186=CARTESIAN_POINT('Ctrl Pts',(83.830782446396,51.7907935901891,30.7050214687829)) ;
#17187=CARTESIAN_POINT('Ctrl Pts',(84.6730288407783,51.2519887801469,30.7681491523808)) ;
#17188=CARTESIAN_POINT('Ctrl Pts',(85.5849579363108,51.6619582113453,30.8312768359787)) ;
#17189=CARTESIAN_POINT('Ctrl Pts',(85.7409918960066,52.6495527773432,30.8944045195766)) ;
#17190=CARTESIAN_POINT('Ctrl Pts',(84.9998717293271,53.320693970801,30.9575322031744)) ;
#17191=CARTESIAN_POINT('Ctrl Pts',(84.0325403827313,53.0677915029774,31.0206598867723)) ;
#17192=CARTESIAN_POINT('Ctrl Pts',(83.7147318465533,52.1198002402525,31.0837875703701)) ;
#17193=CARTESIAN_POINT('Ctrl Pts',(84.3341611644685,51.3349455880624,31.146915253968)) ;
#17194=CARTESIAN_POINT('Ctrl Pts',(85.3300531717214,51.4237634072403,31.2100429375659)) ;
#17195=CARTESIAN_POINT('Ctrl Pts',(85.8008177868754,52.3058467348228,31.2731706211637)) ;
#17196=CARTESIAN_POINT('Ctrl Pts',(85.32026713213,53.1826361032949,31.3362983047616)) ;
#17197=CARTESIAN_POINT('Ctrl Pts',(84.323448807155,53.2603685863375,31.3994259883594)) ;
#17198=CARTESIAN_POINT('Ctrl Pts',(83.712790335882,52.4686669860253,31.4625536719573)) ;
#17199=CARTESIAN_POINT('Ctrl Pts',(84.0411291541956,51.5242767584075,31.5256813555552)) ;
#17200=CARTESIAN_POINT('Ctrl Pts',(85.0112116615207,51.2821414332617,31.5888090391531)) ;
#17201=CARTESIAN_POINT('Ctrl Pts',(85.7448242238094,51.9615123392732,31.6519367227509)) ;
#17202=CARTESIAN_POINT('Ctrl Pts',(85.5777982311225,52.9472594635888,31.7150644063488)) ;
#17203=CARTESIAN_POINT('Ctrl Pts',(84.6613892686054,53.3471579472617,31.7781920899466)) ;
#17204=CARTESIAN_POINT('Ctrl Pts',(83.825138676692,52.7988084219867,31.8413197735445)) ;
#17205=CARTESIAN_POINT('Ctrl Pts',(83.8262990058147,51.7993828754435,31.9044474571424)) ;
#17206=CARTESIAN_POINT('Ctrl Pts',(84.6634370147458,51.2521535395124,31.9675751407403)) ;
#17207=CARTESIAN_POINT('Ctrl Pts',(85.5794790605837,51.6556420626739,32.0307028243381)) ;
#17208=CARTESIAN_POINT('Ctrl Pts',(85.6881803685599,52.3101869753284,32.0727879467367)) ;
#17209=CARTESIAN_POINT('Ctrl Pts',(85.5927405196179,52.5887428689543,32.093830507936)) ;
#17210=CARTESIAN_POINT('Ctrl Pts',(85.2240382136892,51.6371448532496,26.456169492064)) ;
#17211=CARTESIAN_POINT('Ctrl Pts',(85.4431355555749,51.7938314431942,26.4772120532633)) ;
#17212=CARTESIAN_POINT('Ctrl Pts',(85.7100480952787,52.3389596343804,26.5192971756619)) ;
#17213=CARTESIAN_POINT('Ctrl Pts',(85.2424111737292,53.1262070986779,26.5824248592598)) ;
#17214=CARTESIAN_POINT('Ctrl Pts',(84.3282780980173,53.1636376164417,26.6455525428576)) ;
#17215=CARTESIAN_POINT('Ctrl Pts',(83.7962826514255,52.420103103029,26.7086802264555)) ;
#17216=CARTESIAN_POINT('Ctrl Pts',(84.1275240776153,51.567399308897,26.7718079100533)) ;
#17217=CARTESIAN_POINT('Ctrl Pts',(85.022383598147,51.3781418500553,26.8349355936512)) ;
#17218=CARTESIAN_POINT('Ctrl Pts',(85.6706098982882,52.0233445857054,26.8980632772491)) ;
#17219=CARTESIAN_POINT('Ctrl Pts',(85.4854201614629,52.9190585093486,26.9611909608469)) ;
#17220=CARTESIAN_POINT('Ctrl Pts',(84.6344375973004,53.254307179807,27.0243186444448)) ;
#17221=CARTESIAN_POINT('Ctrl Pts',(83.8880797498156,52.7256254839516,27.0874463280427)) ;
#17222=CARTESIAN_POINT('Ctrl Pts',(83.9220238051571,51.8116148233476,27.1505740116406)) ;
#17223=CARTESIAN_POINT('Ctrl Pts',(84.7055435781776,51.3397468719722,27.2137016952384)) ;
#17224=CARTESIAN_POINT('Ctrl Pts',(85.529309561871,51.7372034281971,27.2768293788363)) ;
#17225=CARTESIAN_POINT('Ctrl Pts',(85.6475596910871,52.6441656743055,27.3399570624341)) ;
#17226=CARTESIAN_POINT('Ctrl Pts',(84.9532405902877,53.239551184017,27.403084746032)) ;
#17227=CARTESIAN_POINT('Ctrl Pts',(84.0749259761894,52.9843525049285,27.4662124296298)) ;
#17228=CARTESIAN_POINT('Ctrl Pts',(83.8077620803171,52.1096030876684,27.5293401132278)) ;
#17229=CARTESIAN_POINT('Ctrl Pts',(84.3936148997444,51.4072217993087,27.5924677968256)) ;
#17230=CARTESIAN_POINT('Ctrl Pts',(85.3021064359653,51.5130808462494,27.6555954804235)) ;
#17231=CARTESIAN_POINT('Ctrl Pts',(85.7107709167511,52.3313450874201,27.7187231640213)) ;
#17232=CARTESIAN_POINT('Ctrl Pts',(85.2496406040083,53.1212323259216,27.7818508476192)) ;
#17233=CARTESIAN_POINT('Ctrl Pts',(84.336181035249,53.1676503516375,27.8449785312171)) ;
#17234=CARTESIAN_POINT('Ctrl Pts',(83.7973555997481,52.4285764929403,27.9081062148149)) ;
#17235=CARTESIAN_POINT('Ctrl Pts',(84.1209679454417,51.5731011473719,27.9712338984128)) ;
#17236=CARTESIAN_POINT('Ctrl Pts',(85.0140488242173,51.3756940515816,28.0343615820107)) ;
#17237=CARTESIAN_POINT('Ctrl Pts',(85.6680838618568,52.0150696745107,28.0974892656085)) ;
#17238=CARTESIAN_POINT('Ctrl Pts',(85.490969093377,52.9123953546719,28.1606169492064)) ;
#17239=CARTESIAN_POINT('Ctrl Pts',(84.6430481558181,53.255313859848,28.2237446328043)) ;
#17240=CARTESIAN_POINT('Ctrl Pts',(83.8919517113578,52.7333778976135,28.2868723164021)) ;
#17241=CARTESIAN_POINT('Ctrl Pts',(83.917654313644,51.8191009189187,28.35)) ;
#17242=CARTESIAN_POINT('Ctrl Pts',(84.6968871592499,51.3401863233258,28.4131276835978)) ;
#17243=CARTESIAN_POINT('Ctrl Pts',(85.5242035505155,51.7301999208923,28.4762553671958)) ;
#17244=CARTESIAN_POINT('Ctrl Pts',(85.6506263114499,52.6360587967991,28.5393830507936)) ;
#17245=CARTESIAN_POINT('Ctrl Pts',(84.9617037480403,53.2376805377356,28.6025107343915)) ;
#17246=CARTESIAN_POINT('Ctrl Pts',(84.0811238247283,52.9904114207747,28.6656384179893)) ;
#17247=CARTESIAN_POINT('Ctrl Pts',(83.8060836853867,52.1181064630375,28.7287661015872)) ;
#17248=CARTESIAN_POINT('Ctrl Pts',(84.3855797103871,51.4104714055744,28.791893785185)) ;
#17249=CARTESIAN_POINT('Ctrl Pts',(85.2949887919515,51.508134806656,28.8550214687829)) ;
#17250=CARTESIAN_POINT('Ctrl Pts',(85.7110144827702,52.3226810865697,28.9181491523808)) ;
#17251=CARTESIAN_POINT('Ctrl Pts',(85.257024879574,53.1166939691678,28.9812768359787)) ;
#17252=CARTESIAN_POINT('Ctrl Pts',(84.3440209664122,53.1713462526857,29.0444045195765)) ;
#17253=CARTESIAN_POINT('Ctrl Pts',(83.7985536248668,52.4371607196973,29.1075322031744)) ;
#17254=CARTESIAN_POINT('Ctrl Pts',(84.1144394810533,51.5788023193752,29.1706598867723)) ;
#17255=CARTESIAN_POINT('Ctrl Pts',(85.0057041495988,51.3733508454328,29.2337875703701)) ;
#17256=CARTESIAN_POINT('Ctrl Pts',(85.6654774880105,52.0068034162407,29.296915253968)) ;
#17257=CARTESIAN_POINT('Ctrl Pts',(85.4964605946667,52.9056895643745,29.3600429375659)) ;
#17258=CARTESIAN_POINT('Ctrl Pts',(84.6516660253531,53.2562393514243,29.4231706211637)) ;
#17259=CARTESIAN_POINT('Ctrl Pts',(83.8958941121992,52.7410968150035,29.4862983047616)) ;
#17260=CARTESIAN_POINT('Ctrl Pts',(83.9133521538666,51.8266252548534,29.5494259883595)) ;
#17261=CARTESIAN_POINT('Ctrl Pts',(84.6882352238673,51.3407042269396,29.6125536719573)) ;
#17262=CARTESIAN_POINT('Ctrl Pts',(85.5190345165994,51.7232425292544,29.6756813555552)) ;
#17263=CARTESIAN_POINT('Ctrl Pts',(85.6536197531831,52.6279247008683,29.7388090391531)) ;
#17264=CARTESIAN_POINT('Ctrl Pts',(84.9701496749526,53.2357336097418,29.8019367227509)) ;
#17265=CARTESIAN_POINT('Ctrl Pts',(84.0873760611197,52.9964142326266,29.8650644063488)) ;
#17266=CARTESIAN_POINT('Ctrl Pts',(83.8044820238616,52.1266246136808,29.9281920899467)) ;
#17267=CARTESIAN_POINT('Ctrl Pts',(84.3775741499287,51.4137933344974,29.9913197735445)) ;
#17268=CARTESIAN_POINT('Ctrl Pts',(85.2878268404389,51.5032531409002,30.0544474571424)) ;
#17269=CARTESIAN_POINT('Ctrl Pts',(85.7111799211065,52.3140152432647,30.1175751407402)) ;
#17270=CARTESIAN_POINT('Ctrl Pts',(85.2643679349042,53.1120892163585,30.1807028243381)) ;
#17271=CARTESIAN_POINT('Ctrl Pts',(84.3518939028729,53.17497131565,30.243830507936)) ;
#17272=CARTESIAN_POINT('Ctrl Pts',(83.7998290003106,52.4457337954316,30.3069581915338)) ;
#17273=CARTESIAN_POINT('Ctrl Pts',(84.1079626863004,51.5845621231658,30.3700858751317)) ;
#17274=CARTESIAN_POINT('Ctrl Pts',(84.9973386868094,51.3710829736887,30.4332135587296)) ;
#17275=CARTESIAN_POINT('Ctrl Pts',(85.662796687961,51.9985609941751,30.4963412423274)) ;
#17276=CARTESIAN_POINT('Ctrl Pts',(85.5018914104407,52.898934532948,30.5594689259253)) ;
#17277=CARTESIAN_POINT('Ctrl Pts',(84.6602918891925,53.2570871028643,30.6225966095231)) ;
#17278=CARTESIAN_POINT('Ctrl Pts',(83.8999059499221,52.7487798724213,30.6857242931211)) ;
#17279=CARTESIAN_POINT('Ctrl Pts',(83.9091180115348,51.8341880746922,30.7488519767189)) ;
#17280=CARTESIAN_POINT('Ctrl Pts',(84.6795883100066,51.3413001198369,30.8119796603168)) ;
#17281=CARTESIAN_POINT('Ctrl Pts',(85.51380296157,51.71633202514,30.8751073439147)) ;
#17282=CARTESIAN_POINT('Ctrl Pts',(85.6565397334938,52.6197639485163,30.9382350275125)) ;
#17283=CARTESIAN_POINT('Ctrl Pts',(84.9785777026277,53.2337106024755,31.0013627111104)) ;
#17284=CARTESIAN_POINT('Ctrl Pts',(84.0936821705079,53.0023604403756,31.0644903947082)) ;
#17285=CARTESIAN_POINT('Ctrl Pts',(83.8029572242698,52.1351568334358,31.1276180783061)) ;
#17286=CARTESIAN_POINT('Ctrl Pts',(84.3695988800129,51.4171873625503,31.190745761904)) ;
#17287=CARTESIAN_POINT('Ctrl Pts',(85.2806211380976,51.4984361421331,31.2538734455018)) ;
#17288=CARTESIAN_POINT('Ctrl Pts',(85.7112672720163,52.3053484770657,31.3170011290997)) ;
#17289=CARTESIAN_POINT('Ctrl Pts',(85.2716690631524,53.1074180031918,31.3801288126976)) ;
#17290=CARTESIAN_POINT('Ctrl Pts',(84.3597994279858,53.1785261371183,31.4432564962955)) ;
#17291=CARTESIAN_POINT('Ctrl Pts',(83.8011811688112,52.4542932138767,31.5063841798933)) ;
#17292=CARTESIAN_POINT('Ctrl Pts',(84.1015390083141,51.5903837624384,31.5695118634912)) ;
#17293=CARTESIAN_POINT('Ctrl Pts',(84.9889512477094,51.3688831689305,31.632639547089)) ;
#17294=CARTESIAN_POINT('Ctrl Pts',(85.6600454709664,51.9903582007252,31.6957672306869)) ;
#17295=CARTESIAN_POINT('Ctrl Pts',(85.5072534052524,52.8921001210884,31.7588949142848)) ;
#17296=CARTESIAN_POINT('Ctrl Pts',(84.6689406602144,53.2579193233183,31.8220225978826)) ;
#17297=CARTESIAN_POINT('Ctrl Pts',(83.9039552029347,52.7563000522551,31.8851502814805)) ;
#17298=CARTESIAN_POINT('Ctrl Pts',(83.9050166490049,51.8420453825035,31.9482779650783)) ;
#17299=CARTESIAN_POINT('Ctrl Pts',(84.6708138977735,51.3414508384369,32.0114056486762)) ;
#17300=CARTESIAN_POINT('Ctrl Pts',(85.5087909947098,51.7105541375948,32.0745333322741)) ;
#17301=CARTESIAN_POINT('Ctrl Pts',(85.6082287955236,52.3093188430062,32.1166184546727)) ;
#17302=CARTESIAN_POINT('Ctrl Pts',(85.5209223144381,52.5641362502811,32.137661015872)) ;
#17303=CARTESIAN_POINT('Ctrl Pts',(85.1798773779524,51.6988956497206,26.5)) ;
#17304=CARTESIAN_POINT('Ctrl Pts',(85.3785638722607,51.8409855034509,26.5210425611993)) ;
#17305=CARTESIAN_POINT('Ctrl Pts',(85.6206111574732,52.3353302012154,26.5631276835978)) ;
#17306=CARTESIAN_POINT('Ctrl Pts',(85.1965387349045,53.0492386288041,26.6262553671958)) ;
#17307=CARTESIAN_POINT('Ctrl Pts',(84.3675652084279,53.0831821640869,26.6893830507936)) ;
#17308=CARTESIAN_POINT('Ctrl Pts',(83.8851298244034,52.4089144409102,26.7525107343915)) ;
#17309=CARTESIAN_POINT('Ctrl Pts',(84.1855131936081,51.6356475172613,26.8156384179893)) ;
#17310=CARTESIAN_POINT('Ctrl Pts',(84.9970086663633,51.464021058011,26.8787661015872)) ;
#17311=CARTESIAN_POINT('Ctrl Pts',(85.584846975971,52.0491174747966,26.941893785185)) ;
#17312=CARTESIAN_POINT('Ctrl Pts',(85.4169092945958,52.8613877554865,27.0050214687829)) ;
#17313=CARTESIAN_POINT('Ctrl Pts',(84.6452032531813,53.1654050588536,27.0681491523808)) ;
#17314=CARTESIAN_POINT('Ctrl Pts',(83.968375214374,52.685974720491,27.1312768359787)) ;
#17315=CARTESIAN_POINT('Ctrl Pts',(83.9991570819239,51.8571122050768,27.1944045195765)) ;
#17316=CARTESIAN_POINT('Ctrl Pts',(84.7096850855178,51.4292029103844,27.2575322031744)) ;
#17317=CARTESIAN_POINT('Ctrl Pts',(85.4567100107038,51.7896328869262,27.3206598867723)) ;
#17318=CARTESIAN_POINT('Ctrl Pts',(85.5639440986358,52.6121036097496,27.3837875703701)) ;
#17319=CARTESIAN_POINT('Ctrl Pts',(84.934306938815,53.1520237140672,27.446915253968)) ;
#17320=CARTESIAN_POINT('Ctrl Pts',(84.1378150687031,52.9205990401581,27.5100429375658)) ;
#17321=CARTESIAN_POINT('Ctrl Pts',(83.8955398433635,52.1273402373907,27.5731706211637)) ;
#17322=CARTESIAN_POINT('Ctrl Pts',(84.4268153114771,51.490391953806,27.6362983047616)) ;
#17323=CARTESIAN_POINT('Ctrl Pts',(85.2506728575663,51.5863892979384,27.6994259883594)) ;
#17324=CARTESIAN_POINT('Ctrl Pts',(85.6212666417578,52.3284250163863,27.7625536719573)) ;
#17325=CARTESIAN_POINT('Ctrl Pts',(85.203094680064,53.0447272999564,27.8256813555552)) ;
#17326=CARTESIAN_POINT('Ctrl Pts',(84.3747319174341,53.0868210776482,27.8888090391531)) ;
#17327=CARTESIAN_POINT('Ctrl Pts',(83.8861028181374,52.4165984599033,27.9519367227509)) ;
#17328=CARTESIAN_POINT('Ctrl Pts',(84.1795678229038,51.6408181792509,28.0150644063488)) ;
#17329=CARTESIAN_POINT('Ctrl Pts',(84.989450350052,51.4618012935295,28.0781920899466)) ;
#17330=CARTESIAN_POINT('Ctrl Pts',(85.5825562620867,52.0416134444791,28.1413197735445)) ;
#17331=CARTESIAN_POINT('Ctrl Pts',(85.4219412946177,52.8553453323684,28.2044474571424)) ;
#17332=CARTESIAN_POINT('Ctrl Pts',(84.6530116623168,53.1663179577801,28.2675751407402)) ;
#17333=CARTESIAN_POINT('Ctrl Pts',(83.9718864685879,52.693004928524,28.3307028243381)) ;
#17334=CARTESIAN_POINT('Ctrl Pts',(83.9951946470391,51.8639009048952,28.393830507936)) ;
#17335=CARTESIAN_POINT('Ctrl Pts',(84.7018350882737,51.4296014229731,28.4569581915339)) ;
#17336=CARTESIAN_POINT('Ctrl Pts',(85.4520796692884,51.7832818180256,28.5200858751317)) ;
#17337=CARTESIAN_POINT('Ctrl Pts',(85.566725036296,52.6047519593021,28.5832135587296)) ;
#17338=CARTESIAN_POINT('Ctrl Pts',(84.9419816788649,53.1503273349667,28.6463412423274)) ;
#17339=CARTESIAN_POINT('Ctrl Pts',(84.1434355330495,52.9260935146161,28.7094689259253)) ;
#17340=CARTESIAN_POINT('Ctrl Pts',(83.8940178057069,52.1350514484319,28.7725966095232)) ;
#17341=CARTESIAN_POINT('Ctrl Pts',(84.4195286707959,51.4933388306201,28.835724293121)) ;
#17342=CARTESIAN_POINT('Ctrl Pts',(85.2442182847965,51.5819040255063,28.8988519767189)) ;
#17343=CARTESIAN_POINT('Ctrl Pts',(85.6214875174565,52.3205681435423,28.9619796603168)) ;
#17344=CARTESIAN_POINT('Ctrl Pts',(85.2097910453075,53.0406117311157,29.0251073439146)) ;
#17345=CARTESIAN_POINT('Ctrl Pts',(84.3818414899421,53.090172672954,29.0882350275125)) ;
#17346=CARTESIAN_POINT('Ctrl Pts',(83.887189236662,52.4243829903134,29.1513627111104)) ;
#17347=CARTESIAN_POINT('Ctrl Pts',(84.1736475424871,51.6459882368565,29.2144903947082)) ;
#17348=CARTESIAN_POINT('Ctrl Pts',(84.9818830553883,51.4596763776764,29.2776180783061)) ;
#17349=CARTESIAN_POINT('Ctrl Pts',(85.5801926949256,52.0341172609902,29.340745761904)) ;
#17350=CARTESIAN_POINT('Ctrl Pts',(85.4269212141838,52.8492642455131,29.4038734455019)) ;
#17351=CARTESIAN_POINT('Ctrl Pts',(84.6608267013838,53.1671572316628,29.4670011290997)) ;
#17352=CARTESIAN_POINT('Ctrl Pts',(83.9754616000595,52.7000047607579,29.5301288126976)) ;
#17353=CARTESIAN_POINT('Ctrl Pts',(83.9912932713457,51.8707242826505,29.5932564962954)) ;
#17354=CARTESIAN_POINT('Ctrl Pts',(84.6939891568927,51.4300710793027,29.6563841798933)) ;
#17355=CARTESIAN_POINT('Ctrl Pts',(85.4473921764194,51.7769725687113,29.7195118634912)) ;
#17356=CARTESIAN_POINT('Ctrl Pts',(85.5694396125602,52.5973756260661,29.7826395470891)) ;
#17357=CARTESIAN_POINT('Ctrl Pts',(84.9496407932796,53.1485617804674,29.8457672306869)) ;
#17358=CARTESIAN_POINT('Ctrl Pts',(84.1491053185406,52.9315371116611,29.9088949142848)) ;
#17359=CARTESIAN_POINT('Ctrl Pts',(83.8925653530632,52.1427760583006,29.9720225978826)) ;
#17360=CARTESIAN_POINT('Ctrl Pts',(84.4122688988207,51.4963512925987,30.0351502814805)) ;
#17361=CARTESIAN_POINT('Ctrl Pts',(85.237723532162,51.5774771299215,30.0982779650784)) ;
#17362=CARTESIAN_POINT('Ctrl Pts',(85.6216375437542,52.3127095998846,30.1614056486762)) ;
#17363=CARTESIAN_POINT('Ctrl Pts',(85.2164500303437,53.036435951597,30.2245333322741)) ;
#17364=CARTESIAN_POINT('Ctrl Pts',(84.3889809930133,53.0934600293675,30.2876610158719)) ;
#17365=CARTESIAN_POINT('Ctrl Pts',(83.8883457996475,52.4321574085169,30.3507886994698)) ;
#17366=CARTESIAN_POINT('Ctrl Pts',(84.167774118224,51.6512114641819,30.4139163830677)) ;
#17367=CARTESIAN_POINT('Ctrl Pts',(84.9742969091548,51.4576197781646,30.4770440666656)) ;
#17368=CARTESIAN_POINT('Ctrl Pts',(85.5777616350177,52.0266426931532,30.5401717502634)) ;
#17369=CARTESIAN_POINT('Ctrl Pts',(85.4318461016247,52.8431385047737,30.6032994338613)) ;
#17370=CARTESIAN_POINT('Ctrl Pts',(84.6686489900153,53.1679260075878,30.6664271174592)) ;
#17371=CARTESIAN_POINT('Ctrl Pts',(83.9790996997554,52.7069720736917,30.729554801057)) ;
#17372=CARTESIAN_POINT('Ctrl Pts',(83.9874535766736,51.8775825591953,30.7926824846549)) ;
#17373=CARTESIAN_POINT('Ctrl Pts',(84.6861477792349,51.4306114595269,30.8558101682528)) ;
#17374=CARTESIAN_POINT('Ctrl Pts',(85.4426479868293,51.7707058389346,30.9189378518506)) ;
#17375=CARTESIAN_POINT('Ctrl Pts',(85.5720875709808,52.5899751196893,30.9820655354485)) ;
#17376=CARTESIAN_POINT('Ctrl Pts',(84.9572836759283,53.14672723415,31.0451932190464)) ;
#17377=CARTESIAN_POINT('Ctrl Pts',(84.1548239582845,52.9369293777739,31.1083209026442)) ;
#17378=CARTESIAN_POINT('Ctrl Pts',(83.8911826019863,52.1505134266192,31.1714485862421)) ;
#17379=CARTESIAN_POINT('Ctrl Pts',(84.4050365955573,51.4994291370381,31.2345762698399)) ;
#17380=CARTESIAN_POINT('Ctrl Pts',(85.2311891044738,51.5731088770259,31.2977039534378)) ;
#17381=CARTESIAN_POINT('Ctrl Pts',(85.6217167571572,52.3048502193085,31.3608316370357)) ;
#17382=CARTESIAN_POINT('Ctrl Pts',(85.2230709941749,53.0321999030888,31.4239593206336)) ;
#17383=CARTESIAN_POINT('Ctrl Pts',(84.3961500488167,53.0966836878991,31.4870870042314)) ;
#17384=CARTESIAN_POINT('Ctrl Pts',(83.8895720017401,52.439919441728,31.5502146878293)) ;
#17385=CARTESIAN_POINT('Ctrl Pts',(84.1619488624328,51.6564907664694,31.6133423714271)) ;
#17386=CARTESIAN_POINT('Ctrl Pts',(84.9666908338978,51.4556249045992,31.676470055025)) ;
#17387=CARTESIAN_POINT('Ctrl Pts',(85.5752667181236,52.0192040621772,31.7395977386228)) ;
#17388=CARTESIAN_POINT('Ctrl Pts',(85.4367085793821,52.836940778588,31.8027254222208)) ;
#17389=CARTESIAN_POINT('Ctrl Pts',(84.6764920518234,53.1686806993748,31.8658531058186)) ;
#17390=CARTESIAN_POINT('Ctrl Pts',(83.9827717291772,52.7137916825236,31.9289807894165)) ;
#17391=CARTESIAN_POINT('Ctrl Pts',(83.9837342921951,51.8847078895634,31.9921084730144)) ;
#17392=CARTESIAN_POINT('Ctrl Pts',(84.6781907808013,51.4307481373616,32.0552361566122)) ;
#17393=CARTESIAN_POINT('Ctrl Pts',(85.4381029288359,51.7654662125157,32.1183638402101)) ;
#17394=CARTESIAN_POINT('Ctrl Pts',(85.5282772224873,52.308450710684,32.1604489626087)) ;
#17395=CARTESIAN_POINT('Ctrl Pts',(85.4491041092583,52.5395296316078,32.181491523808)) ;
#17396=CARTESIAN_POINT('Ctrl Pts',(85.6645587247977,52.6133494876276,32.05)) ;
#17397=CARTESIAN_POINT('Ctrl Pts',(85.7681319415962,52.3110551076505,32.0289574388007)) ;
#17398=CARTESIAN_POINT('Ctrl Pts',(85.7091495340268,51.9558925477018,32.0079148776014)) ;
#17399=CARTESIAN_POINT('Ctrl Pts',(85.5139738311189,51.7053323098666,31.9868723164021)) ;
#17400=CARTESIAN_POINT('Ctrl Pts',(85.318798128211,51.4547720720313,31.9658297552029)) ;
#17401=CARTESIAN_POINT('Ctrl Pts',(84.9874291299646,51.3088141563095,31.9447871940036)) ;
#17402=CARTESIAN_POINT('Ctrl Pts',(84.6703315026591,51.3348125530812,31.9237446328043)) ;
#17403=CARTESIAN_POINT('Ctrl Pts',(84.3532338753536,51.360810949853,31.902702071605)) ;
#17404=CARTESIAN_POINT('Ctrl Pts',(84.0504076189891,51.5587656591183,31.8816595104057)) ;
#17405=CARTESIAN_POINT('Ctrl Pts',(83.898784622111,51.8385090843067,31.8606169492064)) ;
#17406=CARTESIAN_POINT('Ctrl Pts',(83.8228117423715,51.9786785443315,31.8500732717675)) ;
#17407=CARTESIAN_POINT('Ctrl Pts',(83.7848007833449,52.1393823285476,31.8395295943286)) ;
#17408=CARTESIAN_POINT('Ctrl Pts',(83.7847843561952,52.3000678891362,31.8289859168897)) ;
#17409=CARTESIAN_POINT('Origin',(84.75,52.3,26.5)) ;
#17410=CARTESIAN_POINT('',(85.81675,52.3,26.4)) ;
#17411=CARTESIAN_POINT('Origin',(85.81675,52.3,26.5)) ;
#17412=CARTESIAN_POINT('Origin',(84.75,52.3,26.4)) ;
#17413=CARTESIAN_POINT('Origin',(84.75,52.3,26.4)) ;
#17414=CARTESIAN_POINT('Origin',(84.75,52.3,32.05)) ;
#17415=CARTESIAN_POINT('Origin',(84.75,52.3,26.4)) ;
#17416=CARTESIAN_POINT('',(83.05,52.3,26.4)) ;
#17417=CARTESIAN_POINT('Origin',(84.75,52.3,26.4)) ;
#17418=CARTESIAN_POINT('Origin',(84.75,52.3,32.225)) ;
#17419=CARTESIAN_POINT('',(84.13325,52.3,32.4)) ;
#17420=CARTESIAN_POINT('',(83.95825,52.3,32.225)) ;
#17421=CARTESIAN_POINT('Origin',(84.75,52.3,32.4)) ;
#17422=CARTESIAN_POINT('Origin',(84.75,52.3,32.4)) ;
#17423=CARTESIAN_POINT('Origin',(86.6949953121991,51.9570448491078,25.8)) ;
#17424=CARTESIAN_POINT('',(86.6111892234686,51.9179336779508,25.8)) ;
#17425=CARTESIAN_POINT('',(86.6296201574069,52.0224606985135,25.8)) ;
#17426=CARTESIAN_POINT('Origin',(84.75,52.3,25.8)) ;
#17427=CARTESIAN_POINT('',(86.4734135677714,51.9961156890829,25.8)) ;
#17428=CARTESIAN_POINT('',(86.4734135677714,51.9961156890829,25.8)) ;
#17429=CARTESIAN_POINT('',(86.9443607650536,52.0755432496147,25.8)) ;
#17430=CARTESIAN_POINT('Origin',(86.9443607650536,52.0755432496147,24.4)) ;
#17431=CARTESIAN_POINT('',(86.6296201574069,52.0224606985135,24.7)) ;
#17432=CARTESIAN_POINT('',(86.6296201574069,52.0224606985135,26.4)) ;
#17433=CARTESIAN_POINT('',(86.4734135677714,51.9961156890829,24.55)) ;
#17434=CARTESIAN_POINT('',(86.4734135677714,51.9961156890829,24.4)) ;
#17435=CARTESIAN_POINT('Ctrl Pts',(86.6296201574069,52.0224606985136,24.7)) ;
#17436=CARTESIAN_POINT('Ctrl Pts',(86.5483071381441,52.0087468579879,24.6215623892917)) ;
#17437=CARTESIAN_POINT('Ctrl Pts',(86.4734135677714,51.9961156890829,24.55)) ;
#17438=CARTESIAN_POINT('Origin',(86.4734135677714,51.9961156890829,24.4)) ;
#17439=CARTESIAN_POINT('',(86.6111892234686,51.9179336779508,24.7)) ;
#17440=CARTESIAN_POINT('',(86.6111892234686,51.9179336779508,26.4)) ;
#17441=CARTESIAN_POINT('Ctrl Pts',(86.4734135677714,51.9961156890829,24.55)) ;
#17442=CARTESIAN_POINT('Ctrl Pts',(86.539470388997,51.9586311631971,24.6215623892931)) ;
#17443=CARTESIAN_POINT('Ctrl Pts',(86.6111892234686,51.9179336779507,24.7)) ;
#17444=CARTESIAN_POINT('Origin',(84.75,52.3,26.4)) ;
#17445=CARTESIAN_POINT('',(86.6492586976664,52.2469302408297,24.7)) ;
#17446=CARTESIAN_POINT('Origin',(84.75,52.3,24.7)) ;
#17447=CARTESIAN_POINT('',(86.6492586976664,52.2469302408297,25.8)) ;
#17448=CARTESIAN_POINT('',(86.6492586976664,52.2469302408297,26.4)) ;
#17449=CARTESIAN_POINT('',(86.6492586976664,52.3530697591703,25.8)) ;
#17450=CARTESIAN_POINT('Origin',(84.75,52.3,25.8)) ;
#17451=CARTESIAN_POINT('',(86.6492586976664,52.3530697591703,24.7)) ;
#17452=CARTESIAN_POINT('',(86.6492586976664,52.3530697591703,26.4)) ;
#17453=CARTESIAN_POINT('',(86.6296201574069,52.5775393014865,24.7)) ;
#17454=CARTESIAN_POINT('Origin',(84.75,52.3,24.7)) ;
#17455=CARTESIAN_POINT('',(86.6296201574069,52.5775393014865,25.8)) ;
#17456=CARTESIAN_POINT('',(86.6296201574069,52.5775393014865,26.4)) ;
#17457=CARTESIAN_POINT('',(86.6111892234686,52.6820663220492,25.8)) ;
#17458=CARTESIAN_POINT('Origin',(84.75,52.3,25.8)) ;
#17459=CARTESIAN_POINT('',(86.6111892234686,52.6820663220492,24.7)) ;
#17460=CARTESIAN_POINT('',(86.6111892234686,52.6820663220492,26.4)) ;
#17461=CARTESIAN_POINT('',(86.5528703097983,52.8997154709092,24.7)) ;
#17462=CARTESIAN_POINT('Origin',(84.75,52.3,24.7)) ;
#17463=CARTESIAN_POINT('',(86.5528703097983,52.8997154709092,25.8)) ;
#17464=CARTESIAN_POINT('',(86.5528703097983,52.8997154709092,26.4)) ;
#17465=CARTESIAN_POINT('',(86.5165684565229,52.9994539930676,25.8)) ;
#17466=CARTESIAN_POINT('Origin',(84.75,52.3,25.8)) ;
#17467=CARTESIAN_POINT('',(86.5165684565229,52.9994539930676,24.7)) ;
#17468=CARTESIAN_POINT('',(86.5165684565229,52.9994539930676,26.4)) ;
#17469=CARTESIAN_POINT('',(86.4213411601228,53.203669589219,24.7)) ;
#17470=CARTESIAN_POINT('Origin',(84.75,52.3,24.7)) ;
#17471=CARTESIAN_POINT('',(86.4213411601228,53.203669589219,25.8)) ;
#17472=CARTESIAN_POINT('',(86.4213411601228,53.203669589219,26.4)) ;
#17473=CARTESIAN_POINT('',(86.3682714009525,53.2955891084474,25.8)) ;
#17474=CARTESIAN_POINT('Origin',(84.75,52.3,25.8)) ;
#17475=CARTESIAN_POINT('',(86.3682714009525,53.2955891084474,24.7)) ;
#17476=CARTESIAN_POINT('',(86.3682714009525,53.2955891084474,26.4)) ;
#17477=CARTESIAN_POINT('',(86.2390291550365,53.4801661643393,24.7)) ;
#17478=CARTESIAN_POINT('Origin',(84.75,52.3,24.7)) ;
#17479=CARTESIAN_POINT('',(86.2390291550365,53.4801661643393,25.8)) ;
#17480=CARTESIAN_POINT('',(86.2390291550365,53.4801661643393,26.4)) ;
#17481=CARTESIAN_POINT('',(86.170803987749,53.5614737525594,25.8)) ;
#17482=CARTESIAN_POINT('Origin',(84.75,52.3,25.8)) ;
#17483=CARTESIAN_POINT('',(86.170803987749,53.5614737525594,24.7)) ;
#17484=CARTESIAN_POINT('',(86.170803987749,53.5614737525594,26.4)) ;
#17485=CARTESIAN_POINT('',(86.0114737525594,53.7208039877491,24.7)) ;
#17486=CARTESIAN_POINT('Origin',(84.75,52.3,24.7)) ;
#17487=CARTESIAN_POINT('',(86.0114737525594,53.7208039877491,25.8)) ;
#17488=CARTESIAN_POINT('',(86.0114737525594,53.7208039877491,26.4)) ;
#17489=CARTESIAN_POINT('',(85.9301661643393,53.7890291550365,25.8)) ;
#17490=CARTESIAN_POINT('Origin',(84.75,52.3,25.8)) ;
#17491=CARTESIAN_POINT('',(85.9301661643393,53.7890291550365,24.7)) ;
#17492=CARTESIAN_POINT('',(85.9301661643393,53.7890291550365,26.4)) ;
#17493=CARTESIAN_POINT('',(85.7455891084474,53.9182714009525,24.7)) ;
#17494=CARTESIAN_POINT('Origin',(84.75,52.3,24.7)) ;
#17495=CARTESIAN_POINT('',(85.7455891084474,53.9182714009525,25.8)) ;
#17496=CARTESIAN_POINT('',(85.7455891084474,53.9182714009525,26.4)) ;
#17497=CARTESIAN_POINT('',(85.653669589219,53.9713411601228,25.8)) ;
#17498=CARTESIAN_POINT('Origin',(84.75,52.3,25.8)) ;
#17499=CARTESIAN_POINT('',(85.653669589219,53.9713411601228,24.7)) ;
#17500=CARTESIAN_POINT('',(85.653669589219,53.9713411601228,26.4)) ;
#17501=CARTESIAN_POINT('',(85.4494539930676,54.0665684565229,24.7)) ;
#17502=CARTESIAN_POINT('Origin',(84.75,52.3,24.7)) ;
#17503=CARTESIAN_POINT('',(85.4494539930676,54.0665684565229,25.8)) ;
#17504=CARTESIAN_POINT('',(85.4494539930676,54.0665684565229,26.4)) ;
#17505=CARTESIAN_POINT('',(85.3497154709092,54.1028703097983,25.8)) ;
#17506=CARTESIAN_POINT('Origin',(84.75,52.3,25.8)) ;
#17507=CARTESIAN_POINT('',(85.3497154709092,54.1028703097983,24.7)) ;
#17508=CARTESIAN_POINT('',(85.3497154709092,54.1028703097983,26.4)) ;
#17509=CARTESIAN_POINT('',(85.1320663220492,54.1611892234686,24.7)) ;
#17510=CARTESIAN_POINT('Origin',(84.75,52.3,24.7)) ;
#17511=CARTESIAN_POINT('',(85.1320663220492,54.1611892234686,25.8)) ;
#17512=CARTESIAN_POINT('',(85.1320663220492,54.1611892234686,26.4)) ;
#17513=CARTESIAN_POINT('',(85.0275393014864,54.1796201574069,25.8)) ;
#17514=CARTESIAN_POINT('Origin',(84.75,52.3,25.8)) ;
#17515=CARTESIAN_POINT('',(85.0275393014864,54.1796201574069,24.7)) ;
#17516=CARTESIAN_POINT('',(85.0275393014864,54.1796201574069,26.4)) ;
#17517=CARTESIAN_POINT('',(84.8030697591703,54.1992586976664,24.7)) ;
#17518=CARTESIAN_POINT('Origin',(84.75,52.3,24.7)) ;
#17519=CARTESIAN_POINT('',(84.8030697591703,54.1992586976664,25.8)) ;
#17520=CARTESIAN_POINT('',(84.8030697591703,54.1992586976664,26.4)) ;
#17521=CARTESIAN_POINT('',(84.6969302408297,54.1992586976664,25.8)) ;
#17522=CARTESIAN_POINT('Origin',(84.75,52.3,25.8)) ;
#17523=CARTESIAN_POINT('',(84.6969302408297,54.1992586976664,24.7)) ;
#17524=CARTESIAN_POINT('',(84.6969302408297,54.1992586976664,26.4)) ;
#17525=CARTESIAN_POINT('',(84.4724606985135,54.1796201574069,24.7)) ;
#17526=CARTESIAN_POINT('Origin',(84.75,52.3,24.7)) ;
#17527=CARTESIAN_POINT('',(84.4724606985135,54.1796201574069,25.8)) ;
#17528=CARTESIAN_POINT('',(84.4724606985135,54.1796201574069,26.4)) ;
#17529=CARTESIAN_POINT('',(84.3679336779508,54.1611892234686,25.8)) ;
#17530=CARTESIAN_POINT('Origin',(84.75,52.3,25.8)) ;
#17531=CARTESIAN_POINT('',(84.3679336779508,54.1611892234686,24.7)) ;
#17532=CARTESIAN_POINT('',(84.3679336779508,54.1611892234686,26.4)) ;
#17533=CARTESIAN_POINT('',(84.1502845290908,54.1028703097983,24.7)) ;
#17534=CARTESIAN_POINT('Origin',(84.75,52.3,24.7)) ;
#17535=CARTESIAN_POINT('',(84.1502845290908,54.1028703097983,25.8)) ;
#17536=CARTESIAN_POINT('',(84.1502845290908,54.1028703097983,26.4)) ;
#17537=CARTESIAN_POINT('',(84.0505460069324,54.0665684565229,25.8)) ;
#17538=CARTESIAN_POINT('Origin',(84.75,52.3,25.8)) ;
#17539=CARTESIAN_POINT('',(84.0505460069324,54.0665684565229,24.7)) ;
#17540=CARTESIAN_POINT('',(84.0505460069324,54.0665684565229,26.4)) ;
#17541=CARTESIAN_POINT('',(83.8463304107809,53.9713411601228,24.7)) ;
#17542=CARTESIAN_POINT('Origin',(84.75,52.3,24.7)) ;
#17543=CARTESIAN_POINT('',(83.8463304107809,53.9713411601228,25.8)) ;
#17544=CARTESIAN_POINT('',(83.8463304107809,53.9713411601228,26.4)) ;
#17545=CARTESIAN_POINT('',(83.7544108915526,53.9182714009525,25.8)) ;
#17546=CARTESIAN_POINT('Origin',(84.75,52.3,25.8)) ;
#17547=CARTESIAN_POINT('',(83.7544108915526,53.9182714009525,24.7)) ;
#17548=CARTESIAN_POINT('',(83.7544108915526,53.9182714009525,26.4)) ;
#17549=CARTESIAN_POINT('',(83.5698338356607,53.7890291550365,24.7)) ;
#17550=CARTESIAN_POINT('Origin',(84.75,52.3,24.7)) ;
#17551=CARTESIAN_POINT('',(83.5698338356607,53.7890291550365,25.8)) ;
#17552=CARTESIAN_POINT('',(83.5698338356607,53.7890291550365,26.4)) ;
#17553=CARTESIAN_POINT('',(83.4885262474406,53.7208039877491,25.8)) ;
#17554=CARTESIAN_POINT('Origin',(84.75,52.3,25.8)) ;
#17555=CARTESIAN_POINT('',(83.4885262474406,53.7208039877491,24.7)) ;
#17556=CARTESIAN_POINT('',(83.4885262474406,53.7208039877491,26.4)) ;
#17557=CARTESIAN_POINT('',(83.3291960122509,53.5614737525594,24.7)) ;
#17558=CARTESIAN_POINT('Origin',(84.75,52.3,24.7)) ;
#17559=CARTESIAN_POINT('',(83.3291960122509,53.5614737525594,25.8)) ;
#17560=CARTESIAN_POINT('',(83.3291960122509,53.5614737525594,26.4)) ;
#17561=CARTESIAN_POINT('',(83.2609708449635,53.4801661643393,25.8)) ;
#17562=CARTESIAN_POINT('Origin',(84.75,52.3,25.8)) ;
#17563=CARTESIAN_POINT('',(83.2609708449635,53.4801661643393,24.7)) ;
#17564=CARTESIAN_POINT('',(83.2609708449635,53.4801661643393,26.4)) ;
#17565=CARTESIAN_POINT('',(83.1317285990475,53.2955891084474,24.7)) ;
#17566=CARTESIAN_POINT('Origin',(84.75,52.3,24.7)) ;
#17567=CARTESIAN_POINT('',(83.1317285990475,53.2955891084474,25.8)) ;
#17568=CARTESIAN_POINT('',(83.1317285990475,53.2955891084474,26.4)) ;
#17569=CARTESIAN_POINT('',(83.0786588398772,53.203669589219,25.8)) ;
#17570=CARTESIAN_POINT('Origin',(84.75,52.3,25.8)) ;
#17571=CARTESIAN_POINT('',(83.0786588398772,53.203669589219,24.7)) ;
#17572=CARTESIAN_POINT('',(83.0786588398772,53.203669589219,26.4)) ;
#17573=CARTESIAN_POINT('',(82.9834315434771,52.9994539930676,24.7)) ;
#17574=CARTESIAN_POINT('Origin',(84.75,52.3,24.7)) ;
#17575=CARTESIAN_POINT('',(82.9834315434771,52.9994539930676,25.8)) ;
#17576=CARTESIAN_POINT('',(82.9834315434771,52.9994539930676,26.4)) ;
#17577=CARTESIAN_POINT('',(82.9471296902017,52.8997154709092,25.8)) ;
#17578=CARTESIAN_POINT('Origin',(84.75,52.3,25.8)) ;
#17579=CARTESIAN_POINT('',(82.9471296902017,52.8997154709092,24.7)) ;
#17580=CARTESIAN_POINT('',(82.9471296902017,52.8997154709092,26.4)) ;
#17581=CARTESIAN_POINT('',(82.8888107765314,52.6820663220492,24.7)) ;
#17582=CARTESIAN_POINT('Origin',(84.75,52.3,24.7)) ;
#17583=CARTESIAN_POINT('',(82.8888107765314,52.6820663220492,25.8)) ;
#17584=CARTESIAN_POINT('',(82.8888107765314,52.6820663220492,26.4)) ;
#17585=CARTESIAN_POINT('',(82.8703798425931,52.5775393014865,25.8)) ;
#17586=CARTESIAN_POINT('Origin',(84.75,52.3,25.8)) ;
#17587=CARTESIAN_POINT('',(82.8703798425931,52.5775393014865,24.7)) ;
#17588=CARTESIAN_POINT('',(82.8703798425931,52.5775393014865,26.4)) ;
#17589=CARTESIAN_POINT('',(82.8507413023336,52.3530697591703,24.7)) ;
#17590=CARTESIAN_POINT('Origin',(84.75,52.3,24.7)) ;
#17591=CARTESIAN_POINT('',(82.8507413023336,52.3530697591703,25.8)) ;
#17592=CARTESIAN_POINT('',(82.8507413023336,52.3530697591703,26.4)) ;
#17593=CARTESIAN_POINT('',(82.85,52.3,25.8)) ;
#17594=CARTESIAN_POINT('Origin',(84.75,52.3,25.8)) ;
#17595=CARTESIAN_POINT('',(82.85,52.3,26.2)) ;
#17596=CARTESIAN_POINT('',(82.85,52.3,26.4)) ;
#17597=CARTESIAN_POINT('Origin',(84.75,52.3,26.2)) ;
#17598=CARTESIAN_POINT('',(82.8507413023336,52.2469302408297,25.8)) ;
#17599=CARTESIAN_POINT('Origin',(84.75,52.3,25.8)) ;
#17600=CARTESIAN_POINT('',(82.8507413023336,52.2469302408297,24.7)) ;
#17601=CARTESIAN_POINT('',(82.8507413023336,52.2469302408297,26.4)) ;
#17602=CARTESIAN_POINT('',(82.8703798425931,52.0224606985135,24.7)) ;
#17603=CARTESIAN_POINT('Origin',(84.75,52.3,24.7)) ;
#17604=CARTESIAN_POINT('',(82.8703798425931,52.0224606985135,25.8)) ;
#17605=CARTESIAN_POINT('',(82.8703798425931,52.0224606985135,26.4)) ;
#17606=CARTESIAN_POINT('',(82.8888107765314,51.9179336779508,25.8)) ;
#17607=CARTESIAN_POINT('Origin',(84.75,52.3,25.8)) ;
#17608=CARTESIAN_POINT('',(82.8888107765314,51.9179336779508,24.7)) ;
#17609=CARTESIAN_POINT('',(82.8888107765314,51.9179336779508,26.4)) ;
#17610=CARTESIAN_POINT('',(82.9471296902017,51.7002845290908,24.7)) ;
#17611=CARTESIAN_POINT('Origin',(84.75,52.3,24.7)) ;
#17612=CARTESIAN_POINT('',(82.9471296902017,51.7002845290908,25.8)) ;
#17613=CARTESIAN_POINT('',(82.9471296902017,51.7002845290908,26.4)) ;
#17614=CARTESIAN_POINT('',(82.9834315434771,51.6005460069324,25.8)) ;
#17615=CARTESIAN_POINT('Origin',(84.75,52.3,25.8)) ;
#17616=CARTESIAN_POINT('',(82.9834315434771,51.6005460069324,24.7)) ;
#17617=CARTESIAN_POINT('',(82.9834315434771,51.6005460069324,26.4)) ;
#17618=CARTESIAN_POINT('',(83.0786588398772,51.396330410781,24.7)) ;
#17619=CARTESIAN_POINT('Origin',(84.75,52.3,24.7)) ;
#17620=CARTESIAN_POINT('',(83.0786588398772,51.396330410781,25.8)) ;
#17621=CARTESIAN_POINT('',(83.0786588398772,51.396330410781,26.4)) ;
#17622=CARTESIAN_POINT('',(83.1317285990474,51.3044108915526,25.8)) ;
#17623=CARTESIAN_POINT('Origin',(84.75,52.3,25.8)) ;
#17624=CARTESIAN_POINT('',(83.1317285990474,51.3044108915526,24.7)) ;
#17625=CARTESIAN_POINT('',(83.1317285990474,51.3044108915526,26.4)) ;
#17626=CARTESIAN_POINT('',(83.2609708449635,51.1198338356607,24.7)) ;
#17627=CARTESIAN_POINT('Origin',(84.75,52.3,24.7)) ;
#17628=CARTESIAN_POINT('',(83.2609708449635,51.1198338356607,25.8)) ;
#17629=CARTESIAN_POINT('',(83.2609708449635,51.1198338356607,26.4)) ;
#17630=CARTESIAN_POINT('',(83.3291960122509,51.0385262474406,25.8)) ;
#17631=CARTESIAN_POINT('Origin',(84.75,52.3,25.8)) ;
#17632=CARTESIAN_POINT('',(83.3291960122509,51.0385262474406,24.7)) ;
#17633=CARTESIAN_POINT('',(83.3291960122509,51.0385262474406,26.4)) ;
#17634=CARTESIAN_POINT('',(83.4885262474406,50.8791960122509,24.7)) ;
#17635=CARTESIAN_POINT('Origin',(84.75,52.3,24.7)) ;
#17636=CARTESIAN_POINT('',(83.4885262474406,50.8791960122509,25.8)) ;
#17637=CARTESIAN_POINT('',(83.4885262474406,50.8791960122509,26.4)) ;
#17638=CARTESIAN_POINT('',(83.5698338356607,50.8109708449635,25.8)) ;
#17639=CARTESIAN_POINT('Origin',(84.75,52.3,25.8)) ;
#17640=CARTESIAN_POINT('',(83.5698338356607,50.8109708449635,24.7)) ;
#17641=CARTESIAN_POINT('',(83.5698338356607,50.8109708449635,26.4)) ;
#17642=CARTESIAN_POINT('',(83.7544108915526,50.6817285990475,24.7)) ;
#17643=CARTESIAN_POINT('Origin',(84.75,52.3,24.7)) ;
#17644=CARTESIAN_POINT('',(83.7544108915526,50.6817285990475,25.8)) ;
#17645=CARTESIAN_POINT('',(83.7544108915526,50.6817285990475,26.4)) ;
#17646=CARTESIAN_POINT('',(83.846330410781,50.6286588398772,25.8)) ;
#17647=CARTESIAN_POINT('Origin',(84.75,52.3,25.8)) ;
#17648=CARTESIAN_POINT('',(83.846330410781,50.6286588398772,24.7)) ;
#17649=CARTESIAN_POINT('',(83.846330410781,50.6286588398772,26.4)) ;
#17650=CARTESIAN_POINT('',(84.0505460069324,50.5334315434771,24.7)) ;
#17651=CARTESIAN_POINT('Origin',(84.75,52.3,24.7)) ;
#17652=CARTESIAN_POINT('',(84.0505460069324,50.5334315434771,25.8)) ;
#17653=CARTESIAN_POINT('',(84.0505460069324,50.5334315434771,26.4)) ;
#17654=CARTESIAN_POINT('',(84.1502845290908,50.4971296902017,25.8)) ;
#17655=CARTESIAN_POINT('Origin',(84.75,52.3,25.8)) ;
#17656=CARTESIAN_POINT('',(84.1502845290908,50.4971296902017,24.7)) ;
#17657=CARTESIAN_POINT('',(84.1502845290908,50.4971296902017,26.4)) ;
#17658=CARTESIAN_POINT('',(84.3679336779508,50.4388107765314,24.7)) ;
#17659=CARTESIAN_POINT('Origin',(84.75,52.3,24.7)) ;
#17660=CARTESIAN_POINT('',(84.3679336779508,50.4388107765314,25.8)) ;
#17661=CARTESIAN_POINT('',(84.3679336779508,50.4388107765314,26.4)) ;
#17662=CARTESIAN_POINT('',(84.4724606985135,50.4203798425931,25.8)) ;
#17663=CARTESIAN_POINT('Origin',(84.75,52.3,25.8)) ;
#17664=CARTESIAN_POINT('',(84.4724606985135,50.4203798425931,24.7)) ;
#17665=CARTESIAN_POINT('',(84.4724606985135,50.4203798425931,26.4)) ;
#17666=CARTESIAN_POINT('',(84.6969302408297,50.4007413023336,24.7)) ;
#17667=CARTESIAN_POINT('Origin',(84.75,52.3,24.7)) ;
#17668=CARTESIAN_POINT('',(84.6969302408297,50.4007413023336,25.8)) ;
#17669=CARTESIAN_POINT('',(84.6969302408297,50.4007413023336,26.4)) ;
#17670=CARTESIAN_POINT('',(84.8030697591703,50.4007413023336,25.8)) ;
#17671=CARTESIAN_POINT('Origin',(84.75,52.3,25.8)) ;
#17672=CARTESIAN_POINT('',(84.8030697591703,50.4007413023336,24.7)) ;
#17673=CARTESIAN_POINT('',(84.8030697591703,50.4007413023336,26.4)) ;
#17674=CARTESIAN_POINT('',(85.0275393014864,50.4203798425931,24.7)) ;
#17675=CARTESIAN_POINT('Origin',(84.75,52.3,24.7)) ;
#17676=CARTESIAN_POINT('',(85.0275393014864,50.4203798425931,25.8)) ;
#17677=CARTESIAN_POINT('',(85.0275393014864,50.4203798425931,26.4)) ;
#17678=CARTESIAN_POINT('',(85.1320663220492,50.4388107765314,25.8)) ;
#17679=CARTESIAN_POINT('Origin',(84.75,52.3,25.8)) ;
#17680=CARTESIAN_POINT('',(85.1320663220492,50.4388107765314,24.7)) ;
#17681=CARTESIAN_POINT('',(85.1320663220492,50.4388107765314,26.4)) ;
#17682=CARTESIAN_POINT('',(85.3497154709092,50.4971296902017,24.7)) ;
#17683=CARTESIAN_POINT('Origin',(84.75,52.3,24.7)) ;
#17684=CARTESIAN_POINT('',(85.3497154709092,50.4971296902017,25.8)) ;
#17685=CARTESIAN_POINT('',(85.3497154709092,50.4971296902017,26.4)) ;
#17686=CARTESIAN_POINT('',(85.4494539930676,50.5334315434771,25.8)) ;
#17687=CARTESIAN_POINT('Origin',(84.75,52.3,25.8)) ;
#17688=CARTESIAN_POINT('',(85.4494539930676,50.5334315434771,24.7)) ;
#17689=CARTESIAN_POINT('',(85.4494539930676,50.5334315434771,26.4)) ;
#17690=CARTESIAN_POINT('',(85.653669589219,50.6286588398772,24.7)) ;
#17691=CARTESIAN_POINT('Origin',(84.75,52.3,24.7)) ;
#17692=CARTESIAN_POINT('',(85.653669589219,50.6286588398772,25.8)) ;
#17693=CARTESIAN_POINT('',(85.653669589219,50.6286588398772,26.4)) ;
#17694=CARTESIAN_POINT('',(85.7455891084474,50.6817285990475,25.8)) ;
#17695=CARTESIAN_POINT('Origin',(84.75,52.3,25.8)) ;
#17696=CARTESIAN_POINT('',(85.7455891084474,50.6817285990475,24.7)) ;
#17697=CARTESIAN_POINT('',(85.7455891084474,50.6817285990475,26.4)) ;
#17698=CARTESIAN_POINT('',(85.9301661643393,50.8109708449635,24.7)) ;
#17699=CARTESIAN_POINT('Origin',(84.75,52.3,24.7)) ;
#17700=CARTESIAN_POINT('',(85.9301661643393,50.8109708449635,25.8)) ;
#17701=CARTESIAN_POINT('',(85.9301661643393,50.8109708449635,26.4)) ;
#17702=CARTESIAN_POINT('',(86.0114737525594,50.879196012251,25.8)) ;
#17703=CARTESIAN_POINT('Origin',(84.75,52.3,25.8)) ;
#17704=CARTESIAN_POINT('',(86.0114737525594,50.879196012251,24.7)) ;
#17705=CARTESIAN_POINT('',(86.0114737525594,50.879196012251,26.4)) ;
#17706=CARTESIAN_POINT('',(86.170803987749,51.0385262474406,24.7)) ;
#17707=CARTESIAN_POINT('Origin',(84.75,52.3,24.7)) ;
#17708=CARTESIAN_POINT('',(86.170803987749,51.0385262474406,25.8)) ;
#17709=CARTESIAN_POINT('',(86.170803987749,51.0385262474406,26.4)) ;
#17710=CARTESIAN_POINT('',(86.2390291550365,51.1198338356607,25.8)) ;
#17711=CARTESIAN_POINT('Origin',(84.75,52.3,25.8)) ;
#17712=CARTESIAN_POINT('',(86.2390291550365,51.1198338356607,24.7)) ;
#17713=CARTESIAN_POINT('',(86.2390291550365,51.1198338356607,26.4)) ;
#17714=CARTESIAN_POINT('',(86.3682714009525,51.3044108915526,24.7)) ;
#17715=CARTESIAN_POINT('Origin',(84.75,52.3,24.7)) ;
#17716=CARTESIAN_POINT('',(86.3682714009525,51.3044108915526,25.8)) ;
#17717=CARTESIAN_POINT('',(86.3682714009525,51.3044108915526,26.4)) ;
#17718=CARTESIAN_POINT('',(86.4213411601228,51.396330410781,25.8)) ;
#17719=CARTESIAN_POINT('Origin',(84.75,52.3,25.8)) ;
#17720=CARTESIAN_POINT('',(86.4213411601228,51.396330410781,24.7)) ;
#17721=CARTESIAN_POINT('',(86.4213411601228,51.396330410781,26.4)) ;
#17722=CARTESIAN_POINT('',(86.5165684565229,51.6005460069324,24.7)) ;
#17723=CARTESIAN_POINT('Origin',(84.75,52.3,24.7)) ;
#17724=CARTESIAN_POINT('',(86.5165684565229,51.6005460069324,25.8)) ;
#17725=CARTESIAN_POINT('',(86.5165684565229,51.6005460069324,26.4)) ;
#17726=CARTESIAN_POINT('',(86.5528703097983,51.7002845290908,25.8)) ;
#17727=CARTESIAN_POINT('Origin',(84.75,52.3,25.8)) ;
#17728=CARTESIAN_POINT('',(86.5528703097983,51.7002845290908,24.7)) ;
#17729=CARTESIAN_POINT('',(86.5528703097983,51.7002845290908,26.4)) ;
#17730=CARTESIAN_POINT('Origin',(84.75,52.3,24.7)) ;
#17731=CARTESIAN_POINT('Origin',(86.8720469886611,51.6979065040093,24.4)) ;
#17732=CARTESIAN_POINT('',(86.3944620863754,51.7014647491801,25.8)) ;
#17733=CARTESIAN_POINT('',(86.8720469886611,51.6979065040093,25.8)) ;
#17734=CARTESIAN_POINT('',(86.3944620863754,51.7014647491801,24.55)) ;
#17735=CARTESIAN_POINT('',(86.3944620863754,51.7014647491801,24.4)) ;
#17736=CARTESIAN_POINT('Ctrl Pts',(86.5528703097983,51.7002845290908,24.7)) ;
#17737=CARTESIAN_POINT('Ctrl Pts',(86.4704112345923,51.7008988902332,24.6215623892926)) ;
#17738=CARTESIAN_POINT('Ctrl Pts',(86.3944620863753,51.7014647491801,24.55)) ;
#17739=CARTESIAN_POINT('Origin',(86.3944620863754,51.7014647491801,24.4)) ;
#17740=CARTESIAN_POINT('Ctrl Pts',(86.3944620863754,51.7014647491801,24.55)) ;
#17741=CARTESIAN_POINT('Ctrl Pts',(86.4530062364447,51.6530790508433,24.6215623892904)) ;
#17742=CARTESIAN_POINT('Ctrl Pts',(86.5165684565229,51.6005460069324,24.7)) ;
#17743=CARTESIAN_POINT('',(86.3944620863754,51.7014647491801,25.8)) ;
#17744=CARTESIAN_POINT('Origin',(86.6058929260522,51.6245102169318,25.8)) ;
#17745=CARTESIAN_POINT('Origin',(84.75,52.3,24.55)) ;
#17746=CARTESIAN_POINT('',(83.15,52.3,24.4)) ;
#17747=CARTESIAN_POINT('Origin',(84.75,52.3,24.4)) ;
#17748=CARTESIAN_POINT('',(83.,52.3,24.55)) ;
#17749=CARTESIAN_POINT('',(83.,52.3,24.55)) ;
#17750=CARTESIAN_POINT('Ctrl Pts',(83.,52.3,24.55)) ;
#17751=CARTESIAN_POINT('Ctrl Pts',(82.9284376107081,52.3254444050815,24.6215623892919)) ;
#17752=CARTESIAN_POINT('Ctrl Pts',(82.8507413023335,52.3530697591703,24.7)) ;
#17753=CARTESIAN_POINT('',(83.0265864322286,52.6038843109171,24.55)) ;
#17754=CARTESIAN_POINT('Ctrl Pts',(82.8703798425931,52.5775393014865,24.7)) ;
#17755=CARTESIAN_POINT('Ctrl Pts',(82.9516928618558,52.5912531420121,24.6215623892918)) ;
#17756=CARTESIAN_POINT('Ctrl Pts',(83.0265864322286,52.6038843109171,24.55)) ;
#17757=CARTESIAN_POINT('Ctrl Pts',(83.0265864322286,52.6038843109171,24.55)) ;
#17758=CARTESIAN_POINT('Ctrl Pts',(82.9605296110049,52.6413688368018,24.6215623892911)) ;
#17759=CARTESIAN_POINT('Ctrl Pts',(82.8888107765314,52.6820663220492,24.7)) ;
#17760=CARTESIAN_POINT('',(83.1055379136246,52.8985352508199,24.55)) ;
#17761=CARTESIAN_POINT('Ctrl Pts',(82.9471296902017,52.8997154709092,24.7)) ;
#17762=CARTESIAN_POINT('Ctrl Pts',(83.0295887654089,52.8991011097668,24.6215623892915)) ;
#17763=CARTESIAN_POINT('Ctrl Pts',(83.1055379136246,52.8985352508199,24.55)) ;
#17764=CARTESIAN_POINT('Ctrl Pts',(83.1055379136246,52.8985352508199,24.55)) ;
#17765=CARTESIAN_POINT('Ctrl Pts',(83.0469937635528,52.9469209491587,24.6215623892935)) ;
#17766=CARTESIAN_POINT('Ctrl Pts',(82.9834315434771,52.9994539930676,24.7)) ;
#17767=CARTESIAN_POINT('',(83.2344555433772,53.175,24.55)) ;
#17768=CARTESIAN_POINT('Ctrl Pts',(83.0786588398772,53.203669589219,24.7)) ;
#17769=CARTESIAN_POINT('Ctrl Pts',(83.159758493753,53.1887456934613,24.621562389293)) ;
#17770=CARTESIAN_POINT('Ctrl Pts',(83.2344555433772,53.175,24.55)) ;
#17771=CARTESIAN_POINT('Ctrl Pts',(83.2344555433772,53.175,24.55)) ;
#17772=CARTESIAN_POINT('Ctrl Pts',(83.185202898835,53.2328166958316,24.621562389293)) ;
#17773=CARTESIAN_POINT('Ctrl Pts',(83.1317285990475,53.2955891084474,24.7)) ;
#17774=CARTESIAN_POINT('',(83.4094222245417,53.4248783169514,24.55)) ;
#17775=CARTESIAN_POINT('Ctrl Pts',(83.2609708449635,53.4801661643393,24.7)) ;
#17776=CARTESIAN_POINT('Ctrl Pts',(83.3382469055668,53.4513861889864,24.6215623892912)) ;
#17777=CARTESIAN_POINT('Ctrl Pts',(83.4094222245417,53.4248783169514,24.5500000000001)) ;
#17778=CARTESIAN_POINT('Ctrl Pts',(83.4094222245417,53.4248783169514,24.55)) ;
#17779=CARTESIAN_POINT('Ctrl Pts',(83.3709576022104,53.4903692792295,24.6215623892924)) ;
#17780=CARTESIAN_POINT('Ctrl Pts',(83.3291960122509,53.5614737525594,24.7)) ;
#17781=CARTESIAN_POINT('',(83.6251216830486,53.6405777754582,24.55)) ;
#17782=CARTESIAN_POINT('Ctrl Pts',(83.4885262474406,53.7208039877491,24.7)) ;
#17783=CARTESIAN_POINT('Ctrl Pts',(83.5596307207712,53.6790423977892,24.6215623892917)) ;
#17784=CARTESIAN_POINT('Ctrl Pts',(83.6251216830486,53.6405777754582,24.55)) ;
#17785=CARTESIAN_POINT('Ctrl Pts',(83.6251216830486,53.6405777754582,24.55)) ;
#17786=CARTESIAN_POINT('Ctrl Pts',(83.5986138110136,53.7117530944334,24.6215623892914)) ;
#17787=CARTESIAN_POINT('Ctrl Pts',(83.5698338356607,53.7890291550365,24.7)) ;
#17788=CARTESIAN_POINT('',(83.875,53.8155444566228,24.55)) ;
#17789=CARTESIAN_POINT('Ctrl Pts',(83.7544108915526,53.9182714009525,24.7)) ;
#17790=CARTESIAN_POINT('Ctrl Pts',(83.8171833041694,53.8647971011641,24.6215623892916)) ;
#17791=CARTESIAN_POINT('Ctrl Pts',(83.875,53.8155444566228,24.55)) ;
#17792=CARTESIAN_POINT('Ctrl Pts',(83.875,53.8155444566228,24.55)) ;
#17793=CARTESIAN_POINT('Ctrl Pts',(83.8612543065387,53.8902415062464,24.6215623892925)) ;
#17794=CARTESIAN_POINT('Ctrl Pts',(83.846330410781,53.9713411601228,24.7)) ;
#17795=CARTESIAN_POINT('',(84.1514647491801,53.9444620863754,24.55)) ;
#17796=CARTESIAN_POINT('Ctrl Pts',(84.0505460069324,54.0665684565229,24.7)) ;
#17797=CARTESIAN_POINT('Ctrl Pts',(84.1030790508414,54.003006236447,24.6215623892933)) ;
#17798=CARTESIAN_POINT('Ctrl Pts',(84.1514647491801,53.9444620863754,24.55)) ;
#17799=CARTESIAN_POINT('Ctrl Pts',(84.1514647491801,53.9444620863754,24.55)) ;
#17800=CARTESIAN_POINT('Ctrl Pts',(84.1508988902332,54.0204112345913,24.6215623892916)) ;
#17801=CARTESIAN_POINT('Ctrl Pts',(84.1502845290908,54.1028703097983,24.7)) ;
#17802=CARTESIAN_POINT('',(84.4461156890829,54.0234135677714,24.55)) ;
#17803=CARTESIAN_POINT('Ctrl Pts',(84.3679336779508,54.1611892234686,24.7)) ;
#17804=CARTESIAN_POINT('Ctrl Pts',(84.4086311631982,54.089470388995,24.6215623892909)) ;
#17805=CARTESIAN_POINT('Ctrl Pts',(84.4461156890829,54.0234135677714,24.55)) ;
#17806=CARTESIAN_POINT('Ctrl Pts',(84.4461156890829,54.0234135677714,24.55)) ;
#17807=CARTESIAN_POINT('Ctrl Pts',(84.4587468579881,54.0983071381452,24.6215623892927)) ;
#17808=CARTESIAN_POINT('Ctrl Pts',(84.4724606985135,54.1796201574069,24.7)) ;
#17809=CARTESIAN_POINT('',(84.75,54.05,24.55)) ;
#17810=CARTESIAN_POINT('Ctrl Pts',(84.6969302408297,54.1992586976664,24.7)) ;
#17811=CARTESIAN_POINT('Ctrl Pts',(84.724555594918,54.1215623892931,24.6215623892931)) ;
#17812=CARTESIAN_POINT('Ctrl Pts',(84.75,54.05,24.55)) ;
#17813=CARTESIAN_POINT('Ctrl Pts',(84.75,54.05,24.55)) ;
#17814=CARTESIAN_POINT('Ctrl Pts',(84.7754444050815,54.1215623892917,24.6215623892917)) ;
#17815=CARTESIAN_POINT('Ctrl Pts',(84.8030697591703,54.1992586976664,24.7)) ;
#17816=CARTESIAN_POINT('',(85.0538843109171,54.0234135677714,24.55)) ;
#17817=CARTESIAN_POINT('Ctrl Pts',(85.0275393014864,54.1796201574069,24.7)) ;
#17818=CARTESIAN_POINT('Ctrl Pts',(85.041253142012,54.0983071381446,24.6215623892922)) ;
#17819=CARTESIAN_POINT('Ctrl Pts',(85.0538843109171,54.0234135677714,24.55)) ;
#17820=CARTESIAN_POINT('Ctrl Pts',(85.0538843109171,54.0234135677714,24.55)) ;
#17821=CARTESIAN_POINT('Ctrl Pts',(85.0913688368026,54.0894703889965,24.6215623892926)) ;
#17822=CARTESIAN_POINT('Ctrl Pts',(85.1320663220492,54.1611892234686,24.7)) ;
#17823=CARTESIAN_POINT('',(85.3485352508199,53.9444620863754,24.55)) ;
#17824=CARTESIAN_POINT('Ctrl Pts',(85.3497154709092,54.1028703097983,24.7)) ;
#17825=CARTESIAN_POINT('Ctrl Pts',(85.3491011097668,54.0204112345911,24.6215623892915)) ;
#17826=CARTESIAN_POINT('Ctrl Pts',(85.3485352508199,53.9444620863754,24.55)) ;
#17827=CARTESIAN_POINT('Ctrl Pts',(85.3485352508199,53.9444620863754,24.55)) ;
#17828=CARTESIAN_POINT('Ctrl Pts',(85.3969209491569,54.0030062364449,24.6215623892907)) ;
#17829=CARTESIAN_POINT('Ctrl Pts',(85.4494539930676,54.0665684565229,24.7)) ;
#17830=CARTESIAN_POINT('',(85.625,53.8155444566228,24.55)) ;
#17831=CARTESIAN_POINT('Ctrl Pts',(85.653669589219,53.9713411601228,24.7)) ;
#17832=CARTESIAN_POINT('Ctrl Pts',(85.6387456934611,53.890241506246,24.6215623892921)) ;
#17833=CARTESIAN_POINT('Ctrl Pts',(85.625,53.8155444566228,24.55)) ;
#17834=CARTESIAN_POINT('Ctrl Pts',(85.625,53.8155444566228,24.55)) ;
#17835=CARTESIAN_POINT('Ctrl Pts',(85.6828166958308,53.8647971011643,24.6215623892919)) ;
#17836=CARTESIAN_POINT('Ctrl Pts',(85.7455891084474,53.9182714009525,24.7)) ;
#17837=CARTESIAN_POINT('',(85.8748783169514,53.6405777754582,24.55)) ;
#17838=CARTESIAN_POINT('Ctrl Pts',(85.9301661643393,53.7890291550365,24.7)) ;
#17839=CARTESIAN_POINT('Ctrl Pts',(85.9013861889865,53.7117530944334,24.6215623892915)) ;
#17840=CARTESIAN_POINT('Ctrl Pts',(85.8748783169514,53.6405777754582,24.55)) ;
#17841=CARTESIAN_POINT('Ctrl Pts',(85.8748783169514,53.6405777754582,24.55)) ;
#17842=CARTESIAN_POINT('Ctrl Pts',(85.9403692792289,53.6790423977892,24.6215623892918)) ;
#17843=CARTESIAN_POINT('Ctrl Pts',(86.0114737525594,53.7208039877491,24.7)) ;
#17844=CARTESIAN_POINT('',(86.0905777754582,53.4248783169514,24.55)) ;
#17845=CARTESIAN_POINT('Ctrl Pts',(86.1708039877491,53.5614737525594,24.7)) ;
#17846=CARTESIAN_POINT('Ctrl Pts',(86.1290423977896,53.4903692792295,24.6215623892925)) ;
#17847=CARTESIAN_POINT('Ctrl Pts',(86.0905777754582,53.4248783169514,24.55)) ;
#17848=CARTESIAN_POINT('Ctrl Pts',(86.0905777754582,53.4248783169514,24.55)) ;
#17849=CARTESIAN_POINT('Ctrl Pts',(86.1617530944339,53.4513861889867,24.621562389292)) ;
#17850=CARTESIAN_POINT('Ctrl Pts',(86.2390291550365,53.4801661643393,24.7)) ;
#17851=CARTESIAN_POINT('',(86.2655444566228,53.175,24.55)) ;
#17852=CARTESIAN_POINT('Ctrl Pts',(86.3682714009525,53.2955891084474,24.7)) ;
#17853=CARTESIAN_POINT('Ctrl Pts',(86.3147971011637,53.2328166958301,24.6215623892911)) ;
#17854=CARTESIAN_POINT('Ctrl Pts',(86.2655444566228,53.175,24.55)) ;
#17855=CARTESIAN_POINT('Ctrl Pts',(86.2655444566228,53.175,24.55)) ;
#17856=CARTESIAN_POINT('Ctrl Pts',(86.3402415062452,53.188745693461,24.6215623892913)) ;
#17857=CARTESIAN_POINT('Ctrl Pts',(86.4213411601228,53.203669589219,24.7)) ;
#17858=CARTESIAN_POINT('',(86.3944620863754,52.8985352508199,24.55)) ;
#17859=CARTESIAN_POINT('Ctrl Pts',(86.5165684565229,52.9994539930676,24.7)) ;
#17860=CARTESIAN_POINT('Ctrl Pts',(86.4530062364461,52.9469209491579,24.6215623892922)) ;
#17861=CARTESIAN_POINT('Ctrl Pts',(86.3944620863754,52.8985352508199,24.55)) ;
#17862=CARTESIAN_POINT('Ctrl Pts',(86.3944620863754,52.8985352508199,24.55)) ;
#17863=CARTESIAN_POINT('Ctrl Pts',(86.4704112345918,52.8991011097668,24.6215623892921)) ;
#17864=CARTESIAN_POINT('Ctrl Pts',(86.5528703097983,52.8997154709092,24.7)) ;
#17865=CARTESIAN_POINT('',(86.4734135677714,52.6038843109171,24.55)) ;
#17866=CARTESIAN_POINT('Ctrl Pts',(86.6111892234686,52.6820663220492,24.7)) ;
#17867=CARTESIAN_POINT('Ctrl Pts',(86.539470388997,52.6413688368029,24.6215623892932)) ;
#17868=CARTESIAN_POINT('Ctrl Pts',(86.4734135677714,52.6038843109171,24.55)) ;
#17869=CARTESIAN_POINT('Ctrl Pts',(86.4734135677714,52.6038843109171,24.55)) ;
#17870=CARTESIAN_POINT('Ctrl Pts',(86.5483071381438,52.5912531420121,24.6215623892914)) ;
#17871=CARTESIAN_POINT('Ctrl Pts',(86.6296201574069,52.5775393014865,24.7)) ;
#17872=CARTESIAN_POINT('',(86.5,52.3,24.55)) ;
#17873=CARTESIAN_POINT('Ctrl Pts',(86.6492586976664,52.3530697591703,24.7)) ;
#17874=CARTESIAN_POINT('Ctrl Pts',(86.571562389291,52.3254444050812,24.621562389291)) ;
#17875=CARTESIAN_POINT('Ctrl Pts',(86.5,52.3,24.55)) ;
#17876=CARTESIAN_POINT('Ctrl Pts',(86.5,52.3,24.55)) ;
#17877=CARTESIAN_POINT('Ctrl Pts',(86.5715623892916,52.2745555949185,24.6215623892916)) ;
#17878=CARTESIAN_POINT('Ctrl Pts',(86.6492586976664,52.2469302408297,24.7)) ;
#17879=CARTESIAN_POINT('',(86.2655444566228,51.425,24.55)) ;
#17880=CARTESIAN_POINT('Ctrl Pts',(86.4213411601228,51.396330410781,24.7)) ;
#17881=CARTESIAN_POINT('Ctrl Pts',(86.340241506248,51.4112543065385,24.621562389294)) ;
#17882=CARTESIAN_POINT('Ctrl Pts',(86.2655444566228,51.425,24.55)) ;
#17883=CARTESIAN_POINT('Ctrl Pts',(86.2655444566228,51.425,24.55)) ;
#17884=CARTESIAN_POINT('Ctrl Pts',(86.3147971011642,51.3671833041693,24.6215623892918)) ;
#17885=CARTESIAN_POINT('Ctrl Pts',(86.3682714009526,51.3044108915526,24.7)) ;
#17886=CARTESIAN_POINT('',(86.0905777754582,51.1751216830486,24.55)) ;
#17887=CARTESIAN_POINT('Ctrl Pts',(86.2390291550365,51.1198338356607,24.7)) ;
#17888=CARTESIAN_POINT('Ctrl Pts',(86.1617530944332,51.1486138110136,24.6215623892913)) ;
#17889=CARTESIAN_POINT('Ctrl Pts',(86.0905777754582,51.1751216830486,24.55)) ;
#17890=CARTESIAN_POINT('Ctrl Pts',(86.0905777754582,51.1751216830486,24.55)) ;
#17891=CARTESIAN_POINT('Ctrl Pts',(86.1290423977896,51.1096307207706,24.6215623892924)) ;
#17892=CARTESIAN_POINT('Ctrl Pts',(86.1708039877491,51.0385262474406,24.7)) ;
#17893=CARTESIAN_POINT('',(85.8748783169514,50.9594222245418,24.55)) ;
#17894=CARTESIAN_POINT('Ctrl Pts',(86.0114737525595,50.8791960122509,24.7)) ;
#17895=CARTESIAN_POINT('Ctrl Pts',(85.940369279228,50.9209576022113,24.6215623892908)) ;
#17896=CARTESIAN_POINT('Ctrl Pts',(85.8748783169514,50.9594222245418,24.55)) ;
#17897=CARTESIAN_POINT('Ctrl Pts',(85.8748783169514,50.9594222245418,24.55)) ;
#17898=CARTESIAN_POINT('Ctrl Pts',(85.9013861889867,50.8882469055658,24.6215623892922)) ;
#17899=CARTESIAN_POINT('Ctrl Pts',(85.9301661643393,50.8109708449635,24.7)) ;
#17900=CARTESIAN_POINT('',(85.625,50.7844555433772,24.55)) ;
#17901=CARTESIAN_POINT('Ctrl Pts',(85.7455891084474,50.6817285990474,24.7)) ;
#17902=CARTESIAN_POINT('Ctrl Pts',(85.6828166958308,50.7352028988357,24.6215623892919)) ;
#17903=CARTESIAN_POINT('Ctrl Pts',(85.625,50.7844555433772,24.55)) ;
#17904=CARTESIAN_POINT('Ctrl Pts',(85.625,50.7844555433772,24.55)) ;
#17905=CARTESIAN_POINT('Ctrl Pts',(85.6387456934614,50.7097584937526,24.6215623892934)) ;
#17906=CARTESIAN_POINT('Ctrl Pts',(85.653669589219,50.6286588398772,24.7)) ;
#17907=CARTESIAN_POINT('',(85.3485352508199,50.6555379136246,24.55)) ;
#17908=CARTESIAN_POINT('Ctrl Pts',(85.4494539930676,50.5334315434771,24.7)) ;
#17909=CARTESIAN_POINT('Ctrl Pts',(85.3969209491577,50.5969937635541,24.6215623892919)) ;
#17910=CARTESIAN_POINT('Ctrl Pts',(85.3485352508199,50.6555379136246,24.55)) ;
#17911=CARTESIAN_POINT('Ctrl Pts',(85.3485352508199,50.6555379136246,24.55)) ;
#17912=CARTESIAN_POINT('Ctrl Pts',(85.3491011097668,50.5795887654084,24.6215623892919)) ;
#17913=CARTESIAN_POINT('Ctrl Pts',(85.3497154709092,50.4971296902017,24.7)) ;
#17914=CARTESIAN_POINT('',(85.0538843109171,50.5765864322286,24.55)) ;
#17915=CARTESIAN_POINT('Ctrl Pts',(85.1320663220493,50.4388107765314,24.7)) ;
#17916=CARTESIAN_POINT('Ctrl Pts',(85.0913688368028,50.5105296110033,24.6215623892928)) ;
#17917=CARTESIAN_POINT('Ctrl Pts',(85.0538843109171,50.5765864322286,24.55)) ;
#17918=CARTESIAN_POINT('Ctrl Pts',(85.0538843109171,50.5765864322286,24.55)) ;
#17919=CARTESIAN_POINT('Ctrl Pts',(85.041253142012,50.5016928618549,24.6215623892927)) ;
#17920=CARTESIAN_POINT('Ctrl Pts',(85.0275393014865,50.4203798425931,24.7)) ;
#17921=CARTESIAN_POINT('',(84.75,50.55,24.55)) ;
#17922=CARTESIAN_POINT('Ctrl Pts',(84.8030697591703,50.4007413023336,24.7)) ;
#17923=CARTESIAN_POINT('Ctrl Pts',(84.7754444050818,50.4784376107076,24.6215623892924)) ;
#17924=CARTESIAN_POINT('Ctrl Pts',(84.75,50.55,24.55)) ;
#17925=CARTESIAN_POINT('Ctrl Pts',(84.75,50.55,24.55)) ;
#17926=CARTESIAN_POINT('Ctrl Pts',(84.7245555949187,50.4784376107088,24.6215623892912)) ;
#17927=CARTESIAN_POINT('Ctrl Pts',(84.6969302408297,50.4007413023336,24.7)) ;
#17928=CARTESIAN_POINT('',(84.4461156890829,50.5765864322286,24.55)) ;
#17929=CARTESIAN_POINT('Ctrl Pts',(84.4724606985135,50.4203798425931,24.7)) ;
#17930=CARTESIAN_POINT('Ctrl Pts',(84.458746857988,50.5016928618554,24.6215623892922)) ;
#17931=CARTESIAN_POINT('Ctrl Pts',(84.4461156890829,50.5765864322286,24.55)) ;
#17932=CARTESIAN_POINT('Ctrl Pts',(84.4461156890829,50.5765864322286,24.55)) ;
#17933=CARTESIAN_POINT('Ctrl Pts',(84.4086311631976,50.5105296110039,24.6215623892921)) ;
#17934=CARTESIAN_POINT('Ctrl Pts',(84.3679336779508,50.4388107765314,24.7)) ;
#17935=CARTESIAN_POINT('',(84.1514647491801,50.6555379136246,24.55)) ;
#17936=CARTESIAN_POINT('Ctrl Pts',(84.1502845290908,50.4971296902017,24.7)) ;
#17937=CARTESIAN_POINT('Ctrl Pts',(84.1508988902331,50.5795887654091,24.6215623892912)) ;
#17938=CARTESIAN_POINT('Ctrl Pts',(84.1514647491801,50.6555379136246,24.55)) ;
#17939=CARTESIAN_POINT('Ctrl Pts',(84.1514647491801,50.6555379136246,24.55)) ;
#17940=CARTESIAN_POINT('Ctrl Pts',(84.1030790508424,50.5969937635541,24.6215623892919)) ;
#17941=CARTESIAN_POINT('Ctrl Pts',(84.0505460069324,50.5334315434771,24.7)) ;
#17942=CARTESIAN_POINT('',(83.875,50.7844555433772,24.55)) ;
#17943=CARTESIAN_POINT('Ctrl Pts',(83.846330410781,50.6286588398772,24.7)) ;
#17944=CARTESIAN_POINT('Ctrl Pts',(83.8612543065388,50.7097584937536,24.6215623892925)) ;
#17945=CARTESIAN_POINT('Ctrl Pts',(83.875,50.7844555433772,24.55)) ;
#17946=CARTESIAN_POINT('Ctrl Pts',(83.875,50.7844555433772,24.55)) ;
#17947=CARTESIAN_POINT('Ctrl Pts',(83.8171833041691,50.7352028988356,24.621562389292)) ;
#17948=CARTESIAN_POINT('Ctrl Pts',(83.7544108915526,50.6817285990475,24.7)) ;
#17949=CARTESIAN_POINT('',(83.6251216830486,50.9594222245418,24.55)) ;
#17950=CARTESIAN_POINT('Ctrl Pts',(83.5698338356607,50.8109708449635,24.7)) ;
#17951=CARTESIAN_POINT('Ctrl Pts',(83.5986138110132,50.8882469055657,24.6215623892923)) ;
#17952=CARTESIAN_POINT('Ctrl Pts',(83.6251216830486,50.9594222245418,24.55)) ;
#17953=CARTESIAN_POINT('Ctrl Pts',(83.6251216830486,50.9594222245418,24.55)) ;
#17954=CARTESIAN_POINT('Ctrl Pts',(83.5596307207711,50.9209576022107,24.6215623892917)) ;
#17955=CARTESIAN_POINT('Ctrl Pts',(83.4885262474406,50.8791960122509,24.7)) ;
#17956=CARTESIAN_POINT('',(83.4094222245418,51.1751216830486,24.55)) ;
#17957=CARTESIAN_POINT('Ctrl Pts',(83.3291960122509,51.0385262474406,24.7)) ;
#17958=CARTESIAN_POINT('Ctrl Pts',(83.3709576022109,51.1096307207714,24.6215623892914)) ;
#17959=CARTESIAN_POINT('Ctrl Pts',(83.4094222245418,51.1751216830486,24.55)) ;
#17960=CARTESIAN_POINT('Ctrl Pts',(83.4094222245418,51.1751216830486,24.55)) ;
#17961=CARTESIAN_POINT('Ctrl Pts',(83.3382469055639,51.1486138110125,24.6215623892941)) ;
#17962=CARTESIAN_POINT('Ctrl Pts',(83.2609708449635,51.1198338356607,24.7)) ;
#17963=CARTESIAN_POINT('',(83.2344555433772,51.425,24.55)) ;
#17964=CARTESIAN_POINT('Ctrl Pts',(83.1317285990474,51.3044108915526,24.7)) ;
#17965=CARTESIAN_POINT('Ctrl Pts',(83.1852028988347,51.3671833041681,24.6215623892934)) ;
#17966=CARTESIAN_POINT('Ctrl Pts',(83.2344555433772,51.425,24.55)) ;
#17967=CARTESIAN_POINT('Ctrl Pts',(83.2344555433772,51.425,24.55)) ;
#17968=CARTESIAN_POINT('Ctrl Pts',(83.1597584937539,51.4112543065388,24.6215623892922)) ;
#17969=CARTESIAN_POINT('Ctrl Pts',(83.0786588398772,51.396330410781,24.7)) ;
#17970=CARTESIAN_POINT('',(83.1055379136246,51.7014647491801,24.55)) ;
#17971=CARTESIAN_POINT('Ctrl Pts',(82.9834315434771,51.6005460069324,24.7)) ;
#17972=CARTESIAN_POINT('Ctrl Pts',(83.0469937635532,51.6530790508416,24.621562389293)) ;
#17973=CARTESIAN_POINT('Ctrl Pts',(83.1055379136246,51.7014647491801,24.55)) ;
#17974=CARTESIAN_POINT('Ctrl Pts',(83.1055379136246,51.7014647491801,24.55)) ;
#17975=CARTESIAN_POINT('Ctrl Pts',(83.0295887654081,51.7008988902332,24.6215623892922)) ;
#17976=CARTESIAN_POINT('Ctrl Pts',(82.9471296902017,51.7002845290908,24.7)) ;
#17977=CARTESIAN_POINT('',(83.0265864322286,51.9961156890829,24.55)) ;
#17978=CARTESIAN_POINT('Ctrl Pts',(82.8888107765314,51.9179336779508,24.7)) ;
#17979=CARTESIAN_POINT('Ctrl Pts',(82.9605296110043,51.9586311631978,24.6215623892918)) ;
#17980=CARTESIAN_POINT('Ctrl Pts',(83.0265864322286,51.9961156890829,24.55)) ;
#17981=CARTESIAN_POINT('Ctrl Pts',(83.0265864322286,51.9961156890829,24.55)) ;
#17982=CARTESIAN_POINT('Ctrl Pts',(82.9516928618564,52.0087468579878,24.6215623892912)) ;
#17983=CARTESIAN_POINT('Ctrl Pts',(82.8703798425931,52.0224606985135,24.7)) ;
#17984=CARTESIAN_POINT('Ctrl Pts',(82.8507413023335,52.2469302408297,24.7)) ;
#17985=CARTESIAN_POINT('Ctrl Pts',(82.928437610706,52.2745555949177,24.621562389294)) ;
#17986=CARTESIAN_POINT('Ctrl Pts',(83.,52.3,24.55)) ;
#17987=CARTESIAN_POINT('Origin',(86.4604001724743,51.3125,25.8)) ;
#17988=CARTESIAN_POINT('',(86.2655444566228,51.425,25.8)) ;
#17989=CARTESIAN_POINT('',(86.2655444566228,51.425,25.8)) ;
#17990=CARTESIAN_POINT('',(86.7352558883258,51.3385640646055,25.8)) ;
#17991=CARTESIAN_POINT('Origin',(86.7352558883258,51.3385640646055,24.4)) ;
#17992=CARTESIAN_POINT('',(86.2655444566228,51.425,24.4)) ;
#17993=CARTESIAN_POINT('Origin',(86.2655444566228,51.425,24.4)) ;
#17994=CARTESIAN_POINT('Origin',(86.5381437924116,51.0084343695886,24.4)) ;
#17995=CARTESIAN_POINT('',(86.0905777754582,51.1751216830486,25.8)) ;
#17996=CARTESIAN_POINT('',(86.5381437924116,51.0084343695886,25.8)) ;
#17997=CARTESIAN_POINT('',(86.0905777754582,51.1751216830486,24.4)) ;
#17998=CARTESIAN_POINT('Origin',(86.0905777754582,51.1751216830486,24.4)) ;
#17999=CARTESIAN_POINT('',(86.0905777754582,51.1751216830486,25.8)) ;
#18000=CARTESIAN_POINT('Origin',(86.26293777516,51.0304944708691,25.8)) ;
#18001=CARTESIAN_POINT('Origin',(86.0195055291309,50.78706222484,25.8)) ;
#18002=CARTESIAN_POINT('',(85.8748783169514,50.9594222245418,25.8)) ;
#18003=CARTESIAN_POINT('',(85.8748783169514,50.9594222245418,25.8)) ;
#18004=CARTESIAN_POINT('',(86.2866998522094,50.7175482426881,25.8)) ;
#18005=CARTESIAN_POINT('Origin',(86.2866998522094,50.7175482426881,24.4)) ;
#18006=CARTESIAN_POINT('',(85.8748783169514,50.9594222245418,24.4)) ;
#18007=CARTESIAN_POINT('Origin',(85.8748783169514,50.9594222245418,24.4)) ;
#18008=CARTESIAN_POINT('Origin',(85.9885640646055,50.4747441116742,24.4)) ;
#18009=CARTESIAN_POINT('',(85.625,50.7844555433772,25.8)) ;
#18010=CARTESIAN_POINT('',(85.9885640646055,50.4747441116742,25.8)) ;
#18011=CARTESIAN_POINT('',(85.625,50.7844555433772,24.4)) ;
#18012=CARTESIAN_POINT('Origin',(85.625,50.7844555433772,24.4)) ;
#18013=CARTESIAN_POINT('',(85.625,50.7844555433772,25.8)) ;
#18014=CARTESIAN_POINT('Origin',(85.7375,50.5895998275257,25.8)) ;
#18015=CARTESIAN_POINT('Origin',(85.4254897830682,50.4441070739478,25.8)) ;
#18016=CARTESIAN_POINT('',(85.3485352508199,50.6555379136246,25.8)) ;
#18017=CARTESIAN_POINT('',(85.3485352508199,50.6555379136246,25.8)) ;
#18018=CARTESIAN_POINT('',(85.6527951346422,50.2873994572031,25.8)) ;
#18019=CARTESIAN_POINT('Origin',(85.6527951346422,50.2873994572031,24.4)) ;
#18020=CARTESIAN_POINT('',(85.3485352508199,50.6555379136246,24.4)) ;
#18021=CARTESIAN_POINT('Origin',(85.3485352508199,50.6555379136246,24.4)) ;
#18022=CARTESIAN_POINT('Origin',(85.2895952313492,50.1612066517998,24.4)) ;
#18023=CARTESIAN_POINT('',(85.0538843109171,50.5765864322286,25.8)) ;
#18024=CARTESIAN_POINT('',(85.2895952313492,50.1612066517998,25.8)) ;
#18025=CARTESIAN_POINT('',(85.0538843109171,50.5765864322286,24.4)) ;
#18026=CARTESIAN_POINT('Origin',(85.0538843109171,50.5765864322286,24.4)) ;
#18027=CARTESIAN_POINT('',(85.0538843109171,50.5765864322286,25.8)) ;
#18028=CARTESIAN_POINT('Origin',(85.0929551508922,50.3550046878009,25.8)) ;
#18029=CARTESIAN_POINT('Origin',(84.75,50.325,25.8)) ;
#18030=CARTESIAN_POINT('',(84.75,50.55,25.8)) ;
#18031=CARTESIAN_POINT('',(84.75,50.55,25.8)) ;
#18032=CARTESIAN_POINT('',(84.91,50.1,25.8)) ;
#18033=CARTESIAN_POINT('Origin',(84.91,50.1,24.4)) ;
#18034=CARTESIAN_POINT('',(84.75,50.55,24.4)) ;
#18035=CARTESIAN_POINT('Origin',(84.75,50.55,24.4)) ;
#18036=CARTESIAN_POINT('Origin',(84.5255432496147,50.1056392349464,24.4)) ;
#18037=CARTESIAN_POINT('',(84.4461156890829,50.5765864322286,25.8)) ;
#18038=CARTESIAN_POINT('',(84.5255432496147,50.1056392349464,25.8)) ;
#18039=CARTESIAN_POINT('',(84.4461156890829,50.5765864322286,24.4)) ;
#18040=CARTESIAN_POINT('Origin',(84.4461156890829,50.5765864322286,24.4)) ;
#18041=CARTESIAN_POINT('',(84.4461156890829,50.5765864322286,25.8)) ;
#18042=CARTESIAN_POINT('Origin',(84.4070448491078,50.3550046878009,25.8)) ;
#18043=CARTESIAN_POINT('Origin',(84.0745102169318,50.4441070739478,25.8)) ;
#18044=CARTESIAN_POINT('',(84.1514647491801,50.6555379136246,25.8)) ;
#18045=CARTESIAN_POINT('',(84.1514647491801,50.6555379136246,25.8)) ;
#18046=CARTESIAN_POINT('',(84.1479065040093,50.1779530113389,25.8)) ;
#18047=CARTESIAN_POINT('Origin',(84.1479065040093,50.1779530113389,24.4)) ;
#18048=CARTESIAN_POINT('',(84.1514647491801,50.6555379136246,24.4)) ;
#18049=CARTESIAN_POINT('Origin',(84.1514647491801,50.6555379136246,24.4)) ;
#18050=CARTESIAN_POINT('Origin',(83.7885640646055,50.3147441116742,24.4)) ;
#18051=CARTESIAN_POINT('',(83.875,50.7844555433772,25.8)) ;
#18052=CARTESIAN_POINT('',(83.7885640646055,50.3147441116742,25.8)) ;
#18053=CARTESIAN_POINT('',(83.875,50.7844555433772,24.4)) ;
#18054=CARTESIAN_POINT('Origin',(83.875,50.7844555433772,24.4)) ;
#18055=CARTESIAN_POINT('',(83.875,50.7844555433772,25.8)) ;
#18056=CARTESIAN_POINT('Origin',(83.7625,50.5895998275257,25.8)) ;
#18057=CARTESIAN_POINT('Origin',(83.4804944708691,50.78706222484,25.8)) ;
#18058=CARTESIAN_POINT('',(83.6251216830486,50.9594222245418,25.8)) ;
#18059=CARTESIAN_POINT('',(83.6251216830486,50.9594222245418,25.8)) ;
#18060=CARTESIAN_POINT('',(83.4584343695887,50.5118562075884,25.8)) ;
#18061=CARTESIAN_POINT('Origin',(83.4584343695887,50.5118562075884,24.4)) ;
#18062=CARTESIAN_POINT('',(83.6251216830486,50.9594222245418,24.4)) ;
#18063=CARTESIAN_POINT('Origin',(83.6251216830486,50.9594222245418,24.4)) ;
#18064=CARTESIAN_POINT('Origin',(83.1675482426881,50.7633001477906,24.4)) ;
#18065=CARTESIAN_POINT('',(83.4094222245418,51.1751216830486,25.8)) ;
#18066=CARTESIAN_POINT('',(83.1675482426881,50.7633001477906,25.8)) ;
#18067=CARTESIAN_POINT('',(83.4094222245418,51.1751216830486,24.4)) ;
#18068=CARTESIAN_POINT('Origin',(83.4094222245418,51.1751216830486,24.4)) ;
#18069=CARTESIAN_POINT('',(83.4094222245418,51.1751216830486,25.8)) ;
#18070=CARTESIAN_POINT('Origin',(83.23706222484,51.0304944708691,25.8)) ;
#18071=CARTESIAN_POINT('Origin',(83.0395998275257,51.3125,25.8)) ;
#18072=CARTESIAN_POINT('',(83.2344555433772,51.425,25.8)) ;
#18073=CARTESIAN_POINT('',(83.2344555433772,51.425,25.8)) ;
#18074=CARTESIAN_POINT('',(82.9247441116742,51.0614359353945,25.8)) ;
#18075=CARTESIAN_POINT('Origin',(82.9247441116742,51.0614359353945,24.4)) ;
#18076=CARTESIAN_POINT('',(83.2344555433772,51.425,24.4)) ;
#18077=CARTESIAN_POINT('Origin',(83.2344555433772,51.425,24.4)) ;
#18078=CARTESIAN_POINT('Origin',(82.7373994572031,51.3972048653578,24.4)) ;
#18079=CARTESIAN_POINT('',(83.1055379136246,51.7014647491801,25.8)) ;
#18080=CARTESIAN_POINT('',(82.7373994572031,51.3972048653578,25.8)) ;
#18081=CARTESIAN_POINT('',(83.1055379136246,51.7014647491801,24.4)) ;
#18082=CARTESIAN_POINT('Origin',(83.1055379136246,51.7014647491801,24.4)) ;
#18083=CARTESIAN_POINT('',(83.1055379136246,51.7014647491801,25.8)) ;
#18084=CARTESIAN_POINT('Origin',(82.8941070739478,51.6245102169318,25.8)) ;
#18085=CARTESIAN_POINT('Origin',(82.8050046878009,51.9570448491078,25.8)) ;
#18086=CARTESIAN_POINT('',(83.0265864322286,51.9961156890829,25.8)) ;
#18087=CARTESIAN_POINT('',(83.0265864322286,51.9961156890829,25.8)) ;
#18088=CARTESIAN_POINT('',(82.6112066517998,51.7604047686508,25.8)) ;
#18089=CARTESIAN_POINT('Origin',(82.6112066517998,51.7604047686508,24.4)) ;
#18090=CARTESIAN_POINT('',(83.0265864322286,51.9961156890829,24.4)) ;
#18091=CARTESIAN_POINT('Origin',(83.0265864322286,51.9961156890829,24.4)) ;
#18092=CARTESIAN_POINT('Origin',(82.55,52.14,24.4)) ;
#18093=CARTESIAN_POINT('',(83.,52.3,25.8)) ;
#18094=CARTESIAN_POINT('',(82.55,52.14,25.8)) ;
#18095=CARTESIAN_POINT('',(83.,52.3,24.4)) ;
#18096=CARTESIAN_POINT('Origin',(83.,52.3,24.4)) ;
#18097=CARTESIAN_POINT('',(83.,52.3,25.8)) ;
#18098=CARTESIAN_POINT('Origin',(82.775,52.3,25.8)) ;
#18099=CARTESIAN_POINT('Origin',(82.8050046878009,52.6429551508922,25.8)) ;
#18100=CARTESIAN_POINT('',(83.0265864322286,52.6038843109171,25.8)) ;
#18101=CARTESIAN_POINT('',(83.0265864322286,52.6038843109171,25.8)) ;
#18102=CARTESIAN_POINT('',(82.5556392349464,52.5244567503853,25.8)) ;
#18103=CARTESIAN_POINT('Origin',(82.5556392349464,52.5244567503853,24.4)) ;
#18104=CARTESIAN_POINT('',(83.0265864322286,52.6038843109171,24.4)) ;
#18105=CARTESIAN_POINT('Origin',(83.0265864322286,52.6038843109171,24.4)) ;
#18106=CARTESIAN_POINT('Origin',(82.6279530113389,52.9020934959907,24.4)) ;
#18107=CARTESIAN_POINT('',(83.1055379136246,52.8985352508199,25.8)) ;
#18108=CARTESIAN_POINT('',(82.6279530113389,52.9020934959907,25.8)) ;
#18109=CARTESIAN_POINT('',(83.1055379136246,52.8985352508199,24.4)) ;
#18110=CARTESIAN_POINT('Origin',(83.1055379136246,52.8985352508199,24.4)) ;
#18111=CARTESIAN_POINT('',(83.1055379136246,52.8985352508199,25.8)) ;
#18112=CARTESIAN_POINT('Origin',(82.8941070739478,52.9754897830682,25.8)) ;
#18113=CARTESIAN_POINT('Origin',(83.0395998275257,53.2875,25.8)) ;
#18114=CARTESIAN_POINT('',(83.2344555433772,53.175,25.8)) ;
#18115=CARTESIAN_POINT('',(83.2344555433772,53.175,25.8)) ;
#18116=CARTESIAN_POINT('',(82.7647441116742,53.2614359353945,25.8)) ;
#18117=CARTESIAN_POINT('Origin',(82.7647441116742,53.2614359353945,24.4)) ;
#18118=CARTESIAN_POINT('',(83.2344555433772,53.175,24.4)) ;
#18119=CARTESIAN_POINT('Origin',(83.2344555433772,53.175,24.4)) ;
#18120=CARTESIAN_POINT('Origin',(82.9618562075884,53.5915656304114,24.4)) ;
#18121=CARTESIAN_POINT('',(83.4094222245417,53.4248783169514,25.8)) ;
#18122=CARTESIAN_POINT('',(82.9618562075884,53.5915656304114,25.8)) ;
#18123=CARTESIAN_POINT('',(83.4094222245417,53.4248783169514,24.4)) ;
#18124=CARTESIAN_POINT('Origin',(83.4094222245417,53.4248783169514,24.4)) ;
#18125=CARTESIAN_POINT('',(83.4094222245417,53.4248783169514,25.8)) ;
#18126=CARTESIAN_POINT('Origin',(83.23706222484,53.5695055291309,25.8)) ;
#18127=CARTESIAN_POINT('Origin',(83.4804944708691,53.81293777516,25.8)) ;
#18128=CARTESIAN_POINT('',(83.6251216830486,53.6405777754582,25.8)) ;
#18129=CARTESIAN_POINT('',(83.6251216830486,53.6405777754582,25.8)) ;
#18130=CARTESIAN_POINT('',(83.2133001477906,53.8824517573119,25.8)) ;
#18131=CARTESIAN_POINT('Origin',(83.2133001477906,53.8824517573119,24.4)) ;
#18132=CARTESIAN_POINT('',(83.6251216830486,53.6405777754582,24.4)) ;
#18133=CARTESIAN_POINT('Origin',(83.6251216830486,53.6405777754582,24.4)) ;
#18134=CARTESIAN_POINT('Origin',(83.5114359353945,54.1252558883258,24.4)) ;
#18135=CARTESIAN_POINT('',(83.875,53.8155444566228,25.8)) ;
#18136=CARTESIAN_POINT('',(83.5114359353945,54.1252558883258,25.8)) ;
#18137=CARTESIAN_POINT('',(83.875,53.8155444566228,24.4)) ;
#18138=CARTESIAN_POINT('Origin',(83.875,53.8155444566228,24.4)) ;
#18139=CARTESIAN_POINT('',(83.875,53.8155444566228,25.8)) ;
#18140=CARTESIAN_POINT('Origin',(83.7625,54.0104001724743,25.8)) ;
#18141=CARTESIAN_POINT('Origin',(84.0745102169318,54.1558929260522,25.8)) ;
#18142=CARTESIAN_POINT('',(84.1514647491801,53.9444620863754,25.8)) ;
#18143=CARTESIAN_POINT('',(84.1514647491801,53.9444620863754,25.8)) ;
#18144=CARTESIAN_POINT('',(83.8472048653578,54.3126005427969,25.8)) ;
#18145=CARTESIAN_POINT('Origin',(83.8472048653578,54.3126005427969,24.4)) ;
#18146=CARTESIAN_POINT('',(84.1514647491801,53.9444620863754,24.4)) ;
#18147=CARTESIAN_POINT('Origin',(84.1514647491801,53.9444620863754,24.4)) ;
#18148=CARTESIAN_POINT('Origin',(84.2104047686508,54.4387933482002,24.4)) ;
#18149=CARTESIAN_POINT('',(84.4461156890829,54.0234135677714,25.8)) ;
#18150=CARTESIAN_POINT('',(84.2104047686508,54.4387933482002,25.8)) ;
#18151=CARTESIAN_POINT('',(84.4461156890829,54.0234135677714,24.4)) ;
#18152=CARTESIAN_POINT('Origin',(84.4461156890829,54.0234135677714,24.4)) ;
#18153=CARTESIAN_POINT('',(84.4461156890829,54.0234135677714,25.8)) ;
#18154=CARTESIAN_POINT('Origin',(84.4070448491078,54.2449953121991,25.8)) ;
#18155=CARTESIAN_POINT('Origin',(84.75,54.275,25.8)) ;
#18156=CARTESIAN_POINT('',(84.75,54.05,25.8)) ;
#18157=CARTESIAN_POINT('',(84.75,54.05,25.8)) ;
#18158=CARTESIAN_POINT('',(84.59,54.5,25.8)) ;
#18159=CARTESIAN_POINT('Origin',(84.59,54.5,24.4)) ;
#18160=CARTESIAN_POINT('',(84.75,54.05,24.4)) ;
#18161=CARTESIAN_POINT('Origin',(84.75,54.05,24.4)) ;
#18162=CARTESIAN_POINT('Origin',(84.9744567503853,54.4943607650536,24.4)) ;
#18163=CARTESIAN_POINT('',(85.0538843109171,54.0234135677714,25.8)) ;
#18164=CARTESIAN_POINT('',(84.9744567503853,54.4943607650536,25.8)) ;
#18165=CARTESIAN_POINT('',(85.0538843109171,54.0234135677714,24.4)) ;
#18166=CARTESIAN_POINT('Origin',(85.0538843109171,54.0234135677714,24.4)) ;
#18167=CARTESIAN_POINT('',(85.0538843109171,54.0234135677714,25.8)) ;
#18168=CARTESIAN_POINT('Origin',(85.0929551508922,54.2449953121991,25.8)) ;
#18169=CARTESIAN_POINT('Origin',(85.4254897830682,54.1558929260522,25.8)) ;
#18170=CARTESIAN_POINT('',(85.3485352508199,53.9444620863754,25.8)) ;
#18171=CARTESIAN_POINT('',(85.3485352508199,53.9444620863754,25.8)) ;
#18172=CARTESIAN_POINT('',(85.3520934959907,54.4220469886611,25.8)) ;
#18173=CARTESIAN_POINT('Origin',(85.3520934959907,54.4220469886611,24.4)) ;
#18174=CARTESIAN_POINT('',(85.3485352508199,53.9444620863754,24.4)) ;
#18175=CARTESIAN_POINT('Origin',(85.3485352508199,53.9444620863754,24.4)) ;
#18176=CARTESIAN_POINT('Origin',(85.7114359353945,54.2852558883258,24.4)) ;
#18177=CARTESIAN_POINT('',(85.625,53.8155444566228,25.8)) ;
#18178=CARTESIAN_POINT('',(85.7114359353945,54.2852558883258,25.8)) ;
#18179=CARTESIAN_POINT('',(85.625,53.8155444566228,24.4)) ;
#18180=CARTESIAN_POINT('Origin',(85.625,53.8155444566228,24.4)) ;
#18181=CARTESIAN_POINT('',(85.625,53.8155444566228,25.8)) ;
#18182=CARTESIAN_POINT('Origin',(85.7375,54.0104001724743,25.8)) ;
#18183=CARTESIAN_POINT('Origin',(86.0195055291309,53.81293777516,25.8)) ;
#18184=CARTESIAN_POINT('',(85.8748783169514,53.6405777754582,25.8)) ;
#18185=CARTESIAN_POINT('',(85.8748783169514,53.6405777754582,25.8)) ;
#18186=CARTESIAN_POINT('',(86.0415656304114,54.0881437924116,25.8)) ;
#18187=CARTESIAN_POINT('Origin',(86.0415656304114,54.0881437924116,24.4)) ;
#18188=CARTESIAN_POINT('',(85.8748783169514,53.6405777754582,24.4)) ;
#18189=CARTESIAN_POINT('Origin',(85.8748783169514,53.6405777754582,24.4)) ;
#18190=CARTESIAN_POINT('Origin',(86.3324517573119,53.8366998522094,24.4)) ;
#18191=CARTESIAN_POINT('',(86.0905777754582,53.4248783169514,25.8)) ;
#18192=CARTESIAN_POINT('',(86.3324517573119,53.8366998522094,25.8)) ;
#18193=CARTESIAN_POINT('',(86.0905777754582,53.4248783169514,24.4)) ;
#18194=CARTESIAN_POINT('Origin',(86.0905777754582,53.4248783169514,24.4)) ;
#18195=CARTESIAN_POINT('',(86.0905777754582,53.4248783169514,25.8)) ;
#18196=CARTESIAN_POINT('Origin',(86.26293777516,53.5695055291309,25.8)) ;
#18197=CARTESIAN_POINT('Origin',(86.4604001724743,53.2875,25.8)) ;
#18198=CARTESIAN_POINT('',(86.2655444566228,53.175,25.8)) ;
#18199=CARTESIAN_POINT('',(86.2655444566228,53.175,25.8)) ;
#18200=CARTESIAN_POINT('',(86.5752558883258,53.5385640646055,25.8)) ;
#18201=CARTESIAN_POINT('Origin',(86.5752558883258,53.5385640646055,24.4)) ;
#18202=CARTESIAN_POINT('',(86.2655444566228,53.175,24.4)) ;
#18203=CARTESIAN_POINT('Origin',(86.2655444566228,53.175,24.4)) ;
#18204=CARTESIAN_POINT('Origin',(86.7626005427969,53.2027951346422,24.4)) ;
#18205=CARTESIAN_POINT('',(86.3944620863754,52.8985352508199,25.8)) ;
#18206=CARTESIAN_POINT('',(86.7626005427969,53.2027951346422,25.8)) ;
#18207=CARTESIAN_POINT('',(86.3944620863754,52.8985352508199,24.4)) ;
#18208=CARTESIAN_POINT('Origin',(86.3944620863754,52.8985352508199,24.4)) ;
#18209=CARTESIAN_POINT('',(86.3944620863754,52.8985352508199,25.8)) ;
#18210=CARTESIAN_POINT('Origin',(86.6058929260522,52.9754897830682,25.8)) ;
#18211=CARTESIAN_POINT('Origin',(86.6949953121991,52.6429551508922,25.8)) ;
#18212=CARTESIAN_POINT('',(86.4734135677714,52.6038843109171,25.8)) ;
#18213=CARTESIAN_POINT('',(86.4734135677714,52.6038843109171,25.8)) ;
#18214=CARTESIAN_POINT('',(86.8887933482002,52.8395952313492,25.8)) ;
#18215=CARTESIAN_POINT('Origin',(86.8887933482002,52.8395952313492,24.4)) ;
#18216=CARTESIAN_POINT('',(86.4734135677714,52.6038843109171,24.4)) ;
#18217=CARTESIAN_POINT('Origin',(86.4734135677714,52.6038843109171,24.4)) ;
#18218=CARTESIAN_POINT('Origin',(86.95,52.46,24.4)) ;
#18219=CARTESIAN_POINT('',(86.5,52.3,25.8)) ;
#18220=CARTESIAN_POINT('',(86.95,52.46,25.8)) ;
#18221=CARTESIAN_POINT('',(86.5,52.3,24.4)) ;
#18222=CARTESIAN_POINT('Origin',(86.5,52.3,24.4)) ;
#18223=CARTESIAN_POINT('',(86.5,52.3,25.8)) ;
#18224=CARTESIAN_POINT('Origin',(86.725,52.3,25.8)) ;
#18225=CARTESIAN_POINT('Origin',(84.75,52.3,26.2)) ;
#18226=CARTESIAN_POINT('Origin',(83.05,52.3,26.2)) ;
#18227=CARTESIAN_POINT('Origin',(84.75,52.3,24.4)) ;
#18228=CARTESIAN_POINT('',(83.7339745962156,52.3,24.4)) ;
#18229=CARTESIAN_POINT('Origin',(84.75,52.3,24.4)) ;
#18230=CARTESIAN_POINT('Origin',(84.75,52.3,24.5)) ;
#18231=CARTESIAN_POINT('',(83.8839745962156,52.3,24.55)) ;
#18232=CARTESIAN_POINT('',(83.8339745962156,52.3,24.5)) ;
#18233=CARTESIAN_POINT('',(83.9397035703159,52.2034745854044,24.6)) ;
#18234=CARTESIAN_POINT('Ctrl Pts',(83.9397035703159,52.2034745854044,24.6)) ;
#18235=CARTESIAN_POINT('Ctrl Pts',(83.9126673723676,52.2503026538944,24.5786927761521)) ;
#18236=CARTESIAN_POINT('Ctrl Pts',(83.8839745962156,52.3,24.55)) ;
#18237=CARTESIAN_POINT('',(84.2612583240074,51.6465254145956,24.6)) ;
#18238=CARTESIAN_POINT('Origin',(84.75,52.3,24.6)) ;
#18239=CARTESIAN_POINT('',(84.3169872981078,51.55,24.55)) ;
#18240=CARTESIAN_POINT('Ctrl Pts',(84.3169872981078,51.55,24.55)) ;
#18241=CARTESIAN_POINT('Ctrl Pts',(84.2882945219557,51.5996973461057,24.5786927761521)) ;
#18242=CARTESIAN_POINT('Ctrl Pts',(84.2612583240074,51.6465254145956,24.6)) ;
#18243=CARTESIAN_POINT('',(84.4284452463086,51.55,24.6)) ;
#18244=CARTESIAN_POINT('Ctrl Pts',(84.4284452463086,51.55,24.6)) ;
#18245=CARTESIAN_POINT('Ctrl Pts',(84.374372850412,51.55,24.5786927761522)) ;
#18246=CARTESIAN_POINT('Ctrl Pts',(84.3169872981078,51.55,24.55)) ;
#18247=CARTESIAN_POINT('',(85.0715547536914,51.55,24.6)) ;
#18248=CARTESIAN_POINT('Origin',(84.75,52.3,24.6)) ;
#18249=CARTESIAN_POINT('',(85.1830127018922,51.55,24.55)) ;
#18250=CARTESIAN_POINT('Ctrl Pts',(85.1830127018922,51.55,24.55)) ;
#18251=CARTESIAN_POINT('Ctrl Pts',(85.125627149588,51.55,24.5786927761521)) ;
#18252=CARTESIAN_POINT('Ctrl Pts',(85.0715547536914,51.55,24.6)) ;
#18253=CARTESIAN_POINT('',(85.2387416759926,51.6465254145956,24.6)) ;
#18254=CARTESIAN_POINT('Ctrl Pts',(85.2387416759926,51.6465254145956,24.6)) ;
#18255=CARTESIAN_POINT('Ctrl Pts',(85.2117054780443,51.5996973461057,24.5786927761521)) ;
#18256=CARTESIAN_POINT('Ctrl Pts',(85.1830127018922,51.55,24.55)) ;
#18257=CARTESIAN_POINT('',(85.560296429684,52.2034745854045,24.6)) ;
#18258=CARTESIAN_POINT('Origin',(84.75,52.3,24.6)) ;
#18259=CARTESIAN_POINT('',(85.6160254037844,52.3,24.55)) ;
#18260=CARTESIAN_POINT('Ctrl Pts',(85.6160254037844,52.3,24.55)) ;
#18261=CARTESIAN_POINT('Ctrl Pts',(85.5873326276323,52.2503026538944,24.5786927761521)) ;
#18262=CARTESIAN_POINT('Ctrl Pts',(85.5602964296841,52.2034745854045,24.6)) ;
#18263=CARTESIAN_POINT('',(85.560296429684,52.3965254145956,24.6)) ;
#18264=CARTESIAN_POINT('Ctrl Pts',(85.560296429684,52.3965254145956,24.6)) ;
#18265=CARTESIAN_POINT('Ctrl Pts',(85.5873326276323,52.3496973461056,24.5786927761521)) ;
#18266=CARTESIAN_POINT('Ctrl Pts',(85.6160254037844,52.3,24.55)) ;
#18267=CARTESIAN_POINT('',(85.2387416759926,52.9534745854044,24.6)) ;
#18268=CARTESIAN_POINT('Origin',(84.75,52.3,24.6)) ;
#18269=CARTESIAN_POINT('',(85.1830127018922,53.05,24.55)) ;
#18270=CARTESIAN_POINT('Ctrl Pts',(85.1830127018922,53.05,24.55)) ;
#18271=CARTESIAN_POINT('Ctrl Pts',(85.2117054780443,53.0003026538944,24.5786927761521)) ;
#18272=CARTESIAN_POINT('Ctrl Pts',(85.2387416759926,52.9534745854044,24.6)) ;
#18273=CARTESIAN_POINT('',(85.0715547536915,53.05,24.6)) ;
#18274=CARTESIAN_POINT('Ctrl Pts',(85.0715547536915,53.05,24.6)) ;
#18275=CARTESIAN_POINT('Ctrl Pts',(85.125627149588,53.05,24.5786927761521)) ;
#18276=CARTESIAN_POINT('Ctrl Pts',(85.1830127018922,53.05,24.55)) ;
#18277=CARTESIAN_POINT('',(84.4284452463085,53.05,24.6)) ;
#18278=CARTESIAN_POINT('Origin',(84.75,52.3,24.6)) ;
#18279=CARTESIAN_POINT('',(84.3169872981078,53.05,24.55)) ;
#18280=CARTESIAN_POINT('Ctrl Pts',(84.3169872981078,53.05,24.55)) ;
#18281=CARTESIAN_POINT('Ctrl Pts',(84.374372850412,53.05,24.5786927761522)) ;
#18282=CARTESIAN_POINT('Ctrl Pts',(84.4284452463085,53.05,24.6)) ;
#18283=CARTESIAN_POINT('',(84.2612583240074,52.9534745854045,24.6)) ;
#18284=CARTESIAN_POINT('Ctrl Pts',(84.2612583240074,52.9534745854045,24.6)) ;
#18285=CARTESIAN_POINT('Ctrl Pts',(84.2882945219557,53.0003026538944,24.5786927761521)) ;
#18286=CARTESIAN_POINT('Ctrl Pts',(84.3169872981078,53.05,24.55)) ;
#18287=CARTESIAN_POINT('',(83.9397035703159,52.3965254145955,24.6)) ;
#18288=CARTESIAN_POINT('Origin',(84.75,52.3,24.6)) ;
#18289=CARTESIAN_POINT('Ctrl Pts',(83.8839745962156,52.3,24.55)) ;
#18290=CARTESIAN_POINT('Ctrl Pts',(83.9126673723676,52.3496973461056,24.5786927761521)) ;
#18291=CARTESIAN_POINT('Ctrl Pts',(83.9397035703159,52.3965254145955,24.6)) ;
#18292=CARTESIAN_POINT('Origin',(84.75,52.3,24.5)) ;
#18293=CARTESIAN_POINT('',(85.560296429684,52.2034745854045,24.4)) ;
#18294=CARTESIAN_POINT('',(85.560296429684,52.2034745854045,24.5)) ;
#18295=CARTESIAN_POINT('',(85.2387416759926,51.6465254145956,24.4)) ;
#18296=CARTESIAN_POINT('',(85.2387416759926,51.6465254145956,24.5)) ;
#18297=CARTESIAN_POINT('Origin',(84.75,52.3,24.4)) ;
#18298=CARTESIAN_POINT('Origin',(84.75,52.3,24.5)) ;
#18299=CARTESIAN_POINT('',(85.2387416759926,52.9534745854044,24.4)) ;
#18300=CARTESIAN_POINT('',(85.2387416759926,52.9534745854044,24.5)) ;
#18301=CARTESIAN_POINT('',(85.560296429684,52.3965254145956,24.4)) ;
#18302=CARTESIAN_POINT('',(85.560296429684,52.3965254145956,24.5)) ;
#18303=CARTESIAN_POINT('Origin',(84.75,52.3,24.4)) ;
#18304=CARTESIAN_POINT('Origin',(84.75,52.3,24.5)) ;
#18305=CARTESIAN_POINT('',(84.4284452463086,51.55,24.4)) ;
#18306=CARTESIAN_POINT('',(84.4284452463086,51.55,24.5)) ;
#18307=CARTESIAN_POINT('',(85.0715547536914,51.55,24.4)) ;
#18308=CARTESIAN_POINT('Origin',(84.75,52.3,24.4)) ;
#18309=CARTESIAN_POINT('',(85.0715547536914,51.55,24.5)) ;
#18310=CARTESIAN_POINT('Origin',(84.75,52.3,24.5)) ;
#18311=CARTESIAN_POINT('',(84.4284452463085,53.05,24.4)) ;
#18312=CARTESIAN_POINT('',(84.4284452463085,53.05,24.5)) ;
#18313=CARTESIAN_POINT('',(85.0715547536915,53.05,24.4)) ;
#18314=CARTESIAN_POINT('',(85.0715547536915,53.05,24.5)) ;
#18315=CARTESIAN_POINT('Origin',(84.75,52.3,24.4)) ;
#18316=CARTESIAN_POINT('Origin',(84.75,52.3,24.5)) ;
#18317=CARTESIAN_POINT('',(83.9397035703159,52.2034745854044,24.4)) ;
#18318=CARTESIAN_POINT('',(83.9397035703159,52.2034745854044,24.5)) ;
#18319=CARTESIAN_POINT('',(84.2612583240074,51.6465254145956,24.4)) ;
#18320=CARTESIAN_POINT('Origin',(84.75,52.3,24.4)) ;
#18321=CARTESIAN_POINT('',(84.2612583240074,51.6465254145956,24.5)) ;
#18322=CARTESIAN_POINT('Origin',(84.75,52.3,24.5)) ;
#18323=CARTESIAN_POINT('',(84.2612583240074,52.9534745854045,24.4)) ;
#18324=CARTESIAN_POINT('',(84.2612583240074,52.9534745854045,24.5)) ;
#18325=CARTESIAN_POINT('',(83.9397035703159,52.3965254145955,24.4)) ;
#18326=CARTESIAN_POINT('Origin',(84.75,52.3,24.4)) ;
#18327=CARTESIAN_POINT('',(83.9397035703159,52.3965254145955,24.5)) ;
#18328=CARTESIAN_POINT('Origin',(85.1830127018922,53.05,24.4)) ;
#18329=CARTESIAN_POINT('',(84.9665063509461,53.05,24.4)) ;
#18330=CARTESIAN_POINT('',(85.1830127018922,53.05,25.4)) ;
#18331=CARTESIAN_POINT('',(85.1830127018922,53.05,24.4)) ;
#18332=CARTESIAN_POINT('',(84.3169872981078,53.05,25.4)) ;
#18333=CARTESIAN_POINT('',(85.1830127018922,53.05,25.4)) ;
#18334=CARTESIAN_POINT('',(84.3169872981078,53.05,24.4)) ;
#18335=CARTESIAN_POINT('Origin',(85.6160254037844,52.3,24.4)) ;
#18336=CARTESIAN_POINT('',(85.5077722283114,52.4875,24.4)) ;
#18337=CARTESIAN_POINT('',(85.6160254037844,52.3,25.4)) ;
#18338=CARTESIAN_POINT('',(85.6160254037844,52.3,24.4)) ;
#18339=CARTESIAN_POINT('',(85.6160254037844,52.3,25.4)) ;
#18340=CARTESIAN_POINT('Origin',(85.1830127018922,51.55,24.4)) ;
#18341=CARTESIAN_POINT('',(85.2912658773653,51.7375,24.4)) ;
#18342=CARTESIAN_POINT('',(85.1830127018922,51.55,25.4)) ;
#18343=CARTESIAN_POINT('',(85.1830127018922,51.55,24.4)) ;
#18344=CARTESIAN_POINT('',(85.1830127018922,51.55,25.4)) ;
#18345=CARTESIAN_POINT('Origin',(84.75,52.3,24.4)) ;
#18346=CARTESIAN_POINT('Origin',(84.75,52.3,24.4)) ;
#18347=CARTESIAN_POINT('Origin',(84.75,52.3,24.4)) ;
#18348=CARTESIAN_POINT('',(84.5334936490539,51.55,24.4)) ;
#18349=CARTESIAN_POINT('Origin',(84.75,52.3,24.4)) ;
#18350=CARTESIAN_POINT('Origin',(84.75,52.3,24.4)) ;
#18351=CARTESIAN_POINT('',(83.9922277716886,52.1125,24.4)) ;
#18352=CARTESIAN_POINT('Origin',(84.75,52.3,24.4)) ;
#18353=CARTESIAN_POINT('',(84.2087341226347,52.8625,24.4)) ;
#18354=CARTESIAN_POINT('Origin',(85.6160254037844,52.3,25.4)) ;
#18355=CARTESIAN_POINT('',(84.3169872981078,51.55,25.4)) ;
#18356=CARTESIAN_POINT('',(84.3169872981078,51.55,25.4)) ;
#18357=CARTESIAN_POINT('Origin',(84.75,52.3,25.4)) ;
#18358=CARTESIAN_POINT('Origin',(85.6160254037844,52.3,25.4)) ;
#18359=CARTESIAN_POINT('Origin',(84.75,52.3,25.4)) ;
#18360=CARTESIAN_POINT('Origin',(85.6160254037844,52.3,25.4)) ;
#18361=CARTESIAN_POINT('Origin',(84.75,52.3,25.4)) ;
#18362=CARTESIAN_POINT('Origin',(85.6160254037844,52.3,25.4)) ;
#18363=CARTESIAN_POINT('Origin',(84.75,52.3,25.4)) ;
#18364=CARTESIAN_POINT('Origin',(85.6160254037844,52.3,25.4)) ;
#18365=CARTESIAN_POINT('',(83.8839745962156,52.3,25.4)) ;
#18366=CARTESIAN_POINT('',(84.3169872981078,53.05,25.4)) ;
#18367=CARTESIAN_POINT('Origin',(84.75,52.3,25.4)) ;
#18368=CARTESIAN_POINT('Origin',(85.6160254037844,52.3,25.4)) ;
#18369=CARTESIAN_POINT('',(83.8839745962156,52.3,25.4)) ;
#18370=CARTESIAN_POINT('Origin',(84.75,52.3,25.4)) ;
#18371=CARTESIAN_POINT('Origin',(84.75,52.3,25.4)) ;
#18372=CARTESIAN_POINT('',(84.75,52.3,25.9203605602115)) ;
#18373=CARTESIAN_POINT('',(83.8839745962156,52.3,25.4)) ;
#18374=CARTESIAN_POINT('Origin',(84.3169872981078,51.55,24.4)) ;
#18375=CARTESIAN_POINT('',(84.3169872981078,51.55,24.4)) ;
#18376=CARTESIAN_POINT('Origin',(83.8839745962156,52.3,24.4)) ;
#18377=CARTESIAN_POINT('',(83.8839745962156,52.3,24.4)) ;
#18378=CARTESIAN_POINT('Origin',(84.3169872981078,53.05,24.4)) ;
#18734=UNCERTAINTY_MEASURE_WITH_UNIT(LENGTH_MEASURE(0.01),#18758,
'DISTANCE_ACCURACY_VALUE',
'Maximum model space distance between geometric entities at asserted c
onnectivities') ;
#18738=UNCERTAINTY_MEASURE_WITH_UNIT(LENGTH_MEASURE(0.01),#18758,
'DISTANCE_ACCURACY_VALUE',
'Maximum model space distance between geometric entities at asserted c
onnectivities') ;
#18753=(
GEOMETRIC_REPRESENTATION_CONTEXT(3)
GLOBAL_UNCERTAINTY_ASSIGNED_CONTEXT((#18734))
GLOBAL_UNIT_ASSIGNED_CONTEXT((#18758,#18760,#18761))
REPRESENTATION_CONTEXT('','3D')
) ;
#18757=(
GEOMETRIC_REPRESENTATION_CONTEXT(3)
GLOBAL_UNCERTAINTY_ASSIGNED_CONTEXT((#18738))
GLOBAL_UNIT_ASSIGNED_CONTEXT((#18758,#18760,#18761))
REPRESENTATION_CONTEXT('','3D')
) ;
#18758=(
LENGTH_UNIT()
NAMED_UNIT(*)
SI_UNIT(.MILLI.,.METRE.)
) ;
#18760=(
NAMED_UNIT(*)
PLANE_ANGLE_UNIT()
SI_UNIT($,.RADIAN.)
) ;
#18761=(
NAMED_UNIT(*)
SI_UNIT($,.STERADIAN.)
SOLID_ANGLE_UNIT()
) ;
#18776=SHAPE_DEFINITION_REPRESENTATION(#18794,#18870) ;
#18794=PRODUCT_DEFINITION_SHAPE('',$,#18889) ;
#18870=SHAPE_REPRESENTATION('',(#10270),#18753) ;
#18874=PRODUCT_DEFINITION_CONTEXT('part definition',#18930,'design') ;
#18889=PRODUCT_DEFINITION('ISO 4762 - M2 x 6 - 12.9',
'ISO 4762 - M2 x 6 - 12.9',#18907,#18874) ;
#18907=PRODUCT_DEFINITION_FORMATION('',$,#18946) ;
#18930=APPLICATION_CONTEXT(
'Core Data for Automotive Mechanical Design Process') ;
#18931=PRODUCT_CONTEXT('part definition',#18930,'mechanical') ;
#18946=PRODUCT('ISO 4762 - M2 x 6 - 12.9','ISO 4762 - M2 x 6 - 12.9',$,(#18931)) ;
#18964=PRESENTATION_STYLE_ASSIGNMENT((#18982)) ;
#18982=SURFACE_STYLE_USAGE(.BOTH.,#19000) ;
#19000=SURFACE_SIDE_STYLE('',(#19018)) ;
#19018=SURFACE_STYLE_FILL_AREA(#19036) ;
#19036=FILL_AREA_STYLE(
'MAS-253 Metallic Sheet - ISO 4762 - M2 x 6 - 12.9',(#19054)) ;
#19054=FILL_AREA_STYLE_COLOUR(
'MAS-253 Metallic Sheet - ISO 4762 - M2 x 6 - 12.9',#19072) ;
#19072=COLOUR_RGB('MAS-253 Metallic Sheet - ISO 4762 - M2 x 6 - 12.9', 0.31764706, 0.68627451, 0.89019608) ;
ENDSEC;
END-ISO-10303-21;
